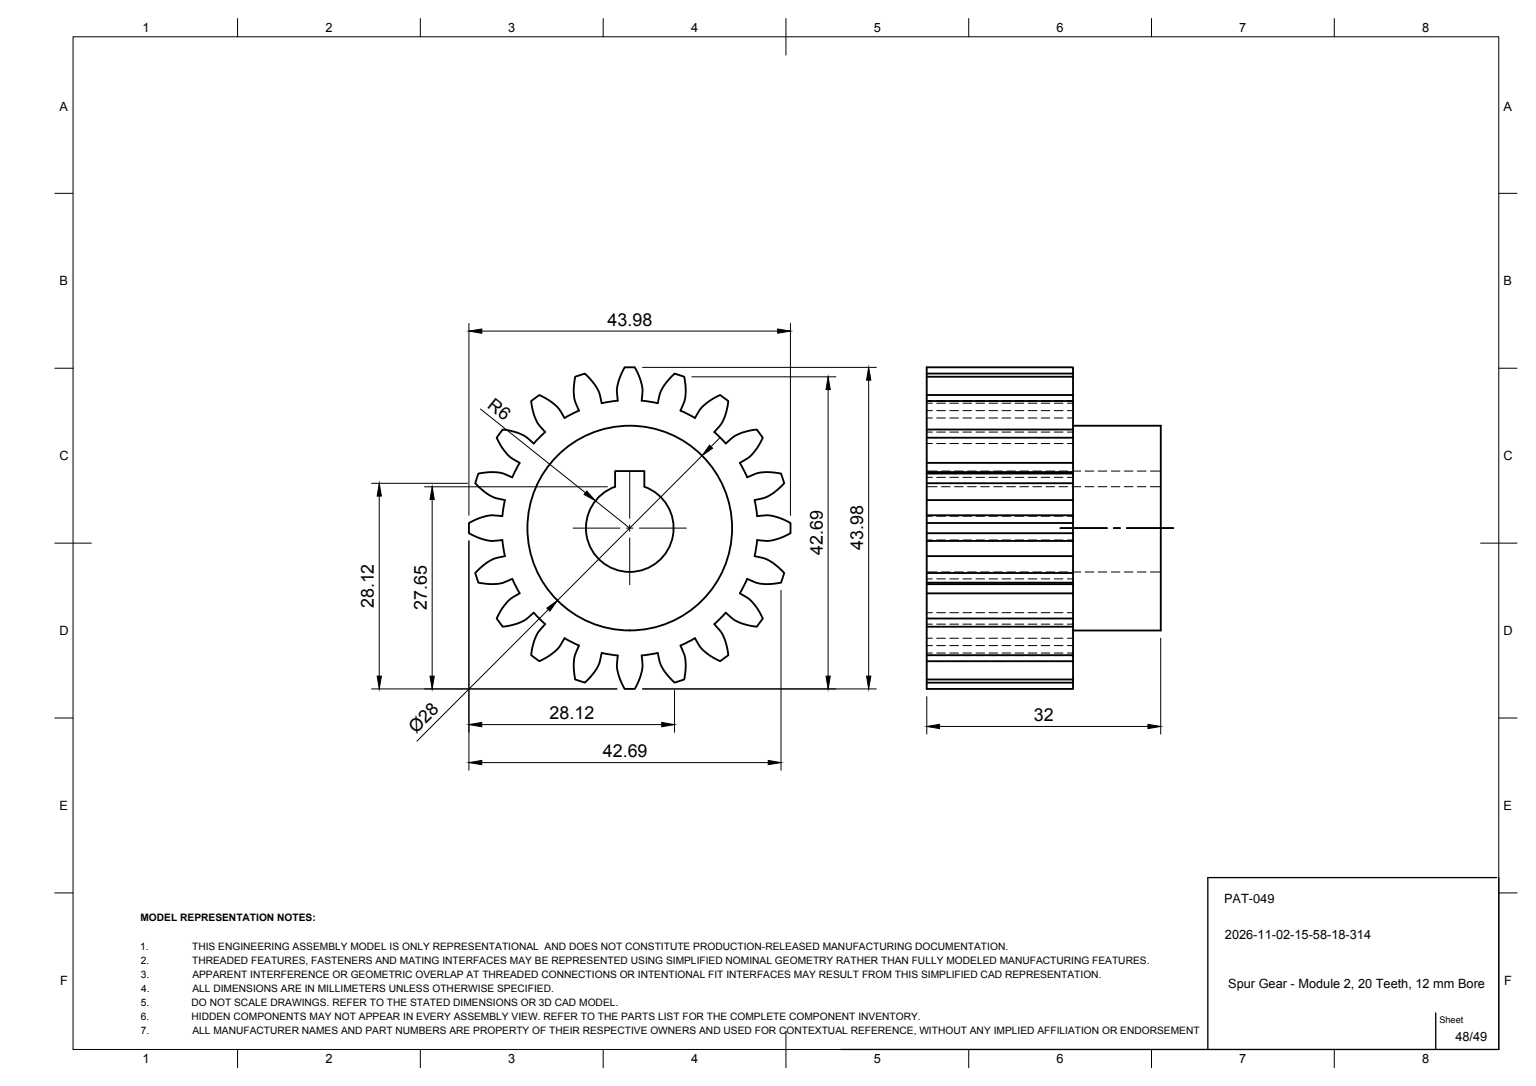
ISO-10303-21;
HEADER;
/* Generated by software containing ST-Developer
 * from STEP Tools, Inc. (www.steptools.com) 
 */

FILE_DESCRIPTION(
/* description */ ('Hand drill press frame (manual)'),
/* implementation_level */ '2;1');

FILE_NAME(
/* name */ 'Spur Gear - Module 2, 20 Teeth, 12 mm Bore.step',
/* time_stamp */ '2026-10-28T03:25:28-07:00',
/* author */ (''),
/* organization */ (''),
/* preprocessor_version */ 'ST-DEVELOPER v20.2',
/* originating_system */ 'Autodesk Translation Framework v15.17.0.0',
/* authorisation */ '');

FILE_SCHEMA (('AUTOMOTIVE_DESIGN { 1 0 10303 214 3 1 1 }'));
ENDSEC;

DATA;
#10=MECHANICAL_DESIGN_GEOMETRIC_PRESENTATION_REPRESENTATION('',(#666),#33299);
#11=(
BOUNDED_SURFACE()
B_SPLINE_SURFACE(5,1,((#24315,#24316),(#24317,#24318),(#24319,#24320),(#24321,
#24322),(#24323,#24324),(#24325,#24326),(#24327,#24328),(#24329,#24330),
(#24331,#24332),(#24333,#24334),(#24335,#24336),(#24337,#24338),(#24339,
#24340),(#24341,#24342),(#24343,#24344),(#24345,#24346),(#24347,#24348),
(#24349,#24350),(#24351,#24352),(#24353,#24354),(#24355,#24356),(#24357,
#24358),(#24359,#24360),(#24361,#24362),(#24363,#24364),(#24365,#24366),
(#24367,#24368),(#24369,#24370),(#24371,#24372),(#24373,#24374),(#24375,
#24376),(#24377,#24378),(#24379,#24380),(#24381,#24382),(#24383,#24384),
(#24385,#24386),(#24387,#24388),(#24389,#24390),(#24391,#24392),(#24393,
#24394),(#24395,#24396),(#24397,#24398),(#24399,#24400),(#24401,#24402),
(#24403,#24404),(#24405,#24406),(#24407,#24408),(#24409,#24410),(#24411,
#24412),(#24413,#24414),(#24415,#24416),(#24417,#24418),(#24419,#24420),
(#24421,#24422),(#24423,#24424),(#24425,#24426),(#24427,#24428),(#24429,
#24430),(#24431,#24432),(#24433,#24434),(#24435,#24436),(#24437,#24438),
(#24439,#24440),(#24441,#24442),(#24443,#24444),(#24445,#24446),(#24447,
#24448),(#24449,#24450),(#24451,#24452),(#24453,#24454)),.UNSPECIFIED.,
 .F.,.F.,.F.)
B_SPLINE_SURFACE_WITH_KNOTS((6,1,1,1,1,1,1,1,1,1,1,1,1,1,1,1,1,1,1,1,1,
1,1,1,1,1,1,1,1,1,1,1,1,1,1,1,1,1,1,1,1,1,1,1,1,1,1,1,1,1,1,1,1,1,1,1,1,
1,1,1,1,1,1,1,1,6),(2,2),(-1.,-0.984615384615383,-0.969230769230768,-0.953846153846152,
-0.938461538461537,-0.923076923076922,-0.907692307692306,-0.892307692307691,
-0.876923076923076,-0.86153846153846,-0.846153846153845,-0.83076923076923,
-0.815384615384614,-0.799999999999999,-0.784615384615384,-0.769230769230768,
-0.753846153846153,-0.738461538461538,-0.723076923076922,-0.707692307692307,
-0.692307692307692,-0.676923076923076,-0.661538461538461,-0.646153846153846,
-0.63076923076923,-0.615384615384615,-0.6,-0.584615384615384,-0.569230769230769,
-0.553846153846154,-0.538461538461538,-0.523076923076923,-0.507692307692308,
-0.492307692307692,-0.476923076923077,-0.461538461538462,-0.446153846153846,
-0.430769230769231,-0.415384615384615,-0.4,-0.384615384615385,-0.369230769230769,
-0.353846153846154,-0.338461538461538,-0.323076923076923,-0.307692307692308,
-0.292307692307692,-0.276923076923077,-0.261538461538462,-0.246153846153846,
-0.230769230769231,-0.215384615384615,-0.2,-0.184615384615385,-0.169230769230769,
-0.153846153846154,-0.138461538461538,-0.123076923076923,-0.107692307692308,
-0.0923076923076923,-0.0769230769230769,-0.0615384615384615,-0.0461538461538462,
-0.0307692307692308,-0.0153846153846154,0.),(-1.,1.),.UNSPECIFIED.)
GEOMETRIC_REPRESENTATION_ITEM()
RATIONAL_B_SPLINE_SURFACE(((1.,1.),(1.,1.),(1.,1.),(1.,1.),(1.,1.),(1.,
1.),(1.,1.),(1.,1.),(1.,1.),(1.,1.),(1.,1.),(1.,1.),(1.,1.),(1.,1.),(1.,
1.),(1.,1.),(1.,1.),(1.,1.),(1.,1.),(1.,1.),(1.,1.),(1.,1.),(1.,1.),(1.,
1.),(1.,1.),(1.,1.),(1.,1.),(1.,1.),(1.,1.),(1.,1.),(1.,1.),(1.,1.),(1.,
1.),(1.,1.),(1.,1.),(1.,1.),(1.,1.),(1.,1.),(1.,1.),(1.,1.),(1.,1.),(1.,
1.),(1.,1.),(1.,1.),(1.,1.),(1.,1.),(1.,1.),(1.,1.),(1.,1.),(1.,1.),(1.,
1.),(1.,1.),(1.,1.),(1.,1.),(1.,1.),(1.,1.),(1.,1.),(1.,1.),(1.,1.),(1.,
1.),(1.,1.),(1.,1.),(1.,1.),(1.,1.),(1.,1.),(1.,1.),(1.,1.),(1.,1.),(1.,
1.),(1.,1.)))
REPRESENTATION_ITEM('')
SURFACE()
);
#12=(
BOUNDED_SURFACE()
B_SPLINE_SURFACE(5,1,((#24533,#24534),(#24535,#24536),(#24537,#24538),(#24539,
#24540),(#24541,#24542),(#24543,#24544),(#24545,#24546),(#24547,#24548),
(#24549,#24550),(#24551,#24552),(#24553,#24554),(#24555,#24556),(#24557,
#24558),(#24559,#24560),(#24561,#24562),(#24563,#24564),(#24565,#24566),
(#24567,#24568),(#24569,#24570),(#24571,#24572),(#24573,#24574),(#24575,
#24576),(#24577,#24578),(#24579,#24580),(#24581,#24582),(#24583,#24584),
(#24585,#24586),(#24587,#24588),(#24589,#24590),(#24591,#24592),(#24593,
#24594),(#24595,#24596),(#24597,#24598),(#24599,#24600),(#24601,#24602),
(#24603,#24604),(#24605,#24606),(#24607,#24608),(#24609,#24610),(#24611,
#24612),(#24613,#24614),(#24615,#24616),(#24617,#24618),(#24619,#24620),
(#24621,#24622),(#24623,#24624),(#24625,#24626),(#24627,#24628),(#24629,
#24630),(#24631,#24632),(#24633,#24634),(#24635,#24636),(#24637,#24638),
(#24639,#24640),(#24641,#24642),(#24643,#24644),(#24645,#24646),(#24647,
#24648),(#24649,#24650),(#24651,#24652),(#24653,#24654),(#24655,#24656),
(#24657,#24658),(#24659,#24660),(#24661,#24662),(#24663,#24664),(#24665,
#24666),(#24667,#24668),(#24669,#24670),(#24671,#24672)),.UNSPECIFIED.,
 .F.,.F.,.F.)
B_SPLINE_SURFACE_WITH_KNOTS((6,1,1,1,1,1,1,1,1,1,1,1,1,1,1,1,1,1,1,1,1,
1,1,1,1,1,1,1,1,1,1,1,1,1,1,1,1,1,1,1,1,1,1,1,1,1,1,1,1,1,1,1,1,1,1,1,1,
1,1,1,1,1,1,1,1,6),(2,2),(-1.,-0.984615384615383,-0.969230769230768,-0.953846153846152,
-0.938461538461537,-0.923076923076922,-0.907692307692306,-0.892307692307691,
-0.876923076923076,-0.86153846153846,-0.846153846153845,-0.83076923076923,
-0.815384615384614,-0.799999999999999,-0.784615384615384,-0.769230769230768,
-0.753846153846153,-0.738461538461538,-0.723076923076922,-0.707692307692307,
-0.692307692307692,-0.676923076923076,-0.661538461538461,-0.646153846153846,
-0.63076923076923,-0.615384615384615,-0.6,-0.584615384615384,-0.569230769230769,
-0.553846153846154,-0.538461538461538,-0.523076923076923,-0.507692307692308,
-0.492307692307692,-0.476923076923077,-0.461538461538462,-0.446153846153846,
-0.430769230769231,-0.415384615384615,-0.4,-0.384615384615385,-0.369230769230769,
-0.353846153846154,-0.338461538461538,-0.323076923076923,-0.307692307692308,
-0.292307692307692,-0.276923076923077,-0.261538461538462,-0.246153846153846,
-0.230769230769231,-0.215384615384615,-0.2,-0.184615384615385,-0.169230769230769,
-0.153846153846154,-0.138461538461538,-0.123076923076923,-0.107692307692308,
-0.0923076923076923,-0.0769230769230769,-0.0615384615384615,-0.0461538461538462,
-0.0307692307692308,-0.0153846153846154,0.),(-1.,1.),.UNSPECIFIED.)
GEOMETRIC_REPRESENTATION_ITEM()
RATIONAL_B_SPLINE_SURFACE(((1.,1.),(1.,1.),(1.,1.),(1.,1.),(1.,1.),(1.,
1.),(1.,1.),(1.,1.),(1.,1.),(1.,1.),(1.,1.),(1.,1.),(1.,1.),(1.,1.),(1.,
1.),(1.,1.),(1.,1.),(1.,1.),(1.,1.),(1.,1.),(1.,1.),(1.,1.),(1.,1.),(1.,
1.),(1.,1.),(1.,1.),(1.,1.),(1.,1.),(1.,1.),(1.,1.),(1.,1.),(1.,1.),(1.,
1.),(1.,1.),(1.,1.),(1.,1.),(1.,1.),(1.,1.),(1.,1.),(1.,1.),(1.,1.),(1.,
1.),(1.,1.),(1.,1.),(1.,1.),(1.,1.),(1.,1.),(1.,1.),(1.,1.),(1.,1.),(1.,
1.),(1.,1.),(1.,1.),(1.,1.),(1.,1.),(1.,1.),(1.,1.),(1.,1.),(1.,1.),(1.,
1.),(1.,1.),(1.,1.),(1.,1.),(1.,1.),(1.,1.),(1.,1.),(1.,1.),(1.,1.),(1.,
1.),(1.,1.)))
REPRESENTATION_ITEM('')
SURFACE()
);
#13=(
BOUNDED_SURFACE()
B_SPLINE_SURFACE(5,1,((#24749,#24750),(#24751,#24752),(#24753,#24754),(#24755,
#24756),(#24757,#24758),(#24759,#24760),(#24761,#24762),(#24763,#24764),
(#24765,#24766),(#24767,#24768),(#24769,#24770),(#24771,#24772),(#24773,
#24774),(#24775,#24776),(#24777,#24778),(#24779,#24780),(#24781,#24782),
(#24783,#24784),(#24785,#24786),(#24787,#24788),(#24789,#24790),(#24791,
#24792),(#24793,#24794),(#24795,#24796),(#24797,#24798),(#24799,#24800),
(#24801,#24802),(#24803,#24804),(#24805,#24806),(#24807,#24808),(#24809,
#24810),(#24811,#24812),(#24813,#24814),(#24815,#24816),(#24817,#24818),
(#24819,#24820),(#24821,#24822),(#24823,#24824),(#24825,#24826),(#24827,
#24828),(#24829,#24830),(#24831,#24832),(#24833,#24834),(#24835,#24836),
(#24837,#24838),(#24839,#24840),(#24841,#24842),(#24843,#24844),(#24845,
#24846),(#24847,#24848),(#24849,#24850),(#24851,#24852),(#24853,#24854),
(#24855,#24856),(#24857,#24858),(#24859,#24860),(#24861,#24862),(#24863,
#24864),(#24865,#24866),(#24867,#24868),(#24869,#24870),(#24871,#24872),
(#24873,#24874),(#24875,#24876),(#24877,#24878),(#24879,#24880),(#24881,
#24882),(#24883,#24884),(#24885,#24886),(#24887,#24888)),.UNSPECIFIED.,
 .F.,.F.,.F.)
B_SPLINE_SURFACE_WITH_KNOTS((6,1,1,1,1,1,1,1,1,1,1,1,1,1,1,1,1,1,1,1,1,
1,1,1,1,1,1,1,1,1,1,1,1,1,1,1,1,1,1,1,1,1,1,1,1,1,1,1,1,1,1,1,1,1,1,1,1,
1,1,1,1,1,1,1,1,6),(2,2),(-1.,-0.984615384615383,-0.969230769230768,-0.953846153846152,
-0.938461538461537,-0.923076923076922,-0.907692307692306,-0.892307692307691,
-0.876923076923076,-0.86153846153846,-0.846153846153845,-0.83076923076923,
-0.815384615384614,-0.799999999999999,-0.784615384615384,-0.769230769230768,
-0.753846153846153,-0.738461538461538,-0.723076923076922,-0.707692307692307,
-0.692307692307692,-0.676923076923076,-0.661538461538461,-0.646153846153846,
-0.63076923076923,-0.615384615384615,-0.6,-0.584615384615384,-0.569230769230769,
-0.553846153846154,-0.538461538461538,-0.523076923076923,-0.507692307692308,
-0.492307692307692,-0.476923076923077,-0.461538461538462,-0.446153846153846,
-0.430769230769231,-0.415384615384615,-0.4,-0.384615384615385,-0.369230769230769,
-0.353846153846154,-0.338461538461538,-0.323076923076923,-0.307692307692308,
-0.292307692307692,-0.276923076923077,-0.261538461538462,-0.246153846153846,
-0.230769230769231,-0.215384615384615,-0.2,-0.184615384615385,-0.169230769230769,
-0.153846153846154,-0.138461538461538,-0.123076923076923,-0.107692307692308,
-0.0923076923076923,-0.0769230769230769,-0.0615384615384615,-0.0461538461538462,
-0.0307692307692308,-0.0153846153846154,0.),(-1.,1.),.UNSPECIFIED.)
GEOMETRIC_REPRESENTATION_ITEM()
RATIONAL_B_SPLINE_SURFACE(((1.,1.),(1.,1.),(1.,1.),(1.,1.),(1.,1.),(1.,
1.),(1.,1.),(1.,1.),(1.,1.),(1.,1.),(1.,1.),(1.,1.),(1.,1.),(1.,1.),(1.,
1.),(1.,1.),(1.,1.),(1.,1.),(1.,1.),(1.,1.),(1.,1.),(1.,1.),(1.,1.),(1.,
1.),(1.,1.),(1.,1.),(1.,1.),(1.,1.),(1.,1.),(1.,1.),(1.,1.),(1.,1.),(1.,
1.),(1.,1.),(1.,1.),(1.,1.),(1.,1.),(1.,1.),(1.,1.),(1.,1.),(1.,1.),(1.,
1.),(1.,1.),(1.,1.),(1.,1.),(1.,1.),(1.,1.),(1.,1.),(1.,1.),(1.,1.),(1.,
1.),(1.,1.),(1.,1.),(1.,1.),(1.,1.),(1.,1.),(1.,1.),(1.,1.),(1.,1.),(1.,
1.),(1.,1.),(1.,1.),(1.,1.),(1.,1.),(1.,1.),(1.,1.),(1.,1.),(1.,1.),(1.,
1.),(1.,1.)))
REPRESENTATION_ITEM('')
SURFACE()
);
#14=(
BOUNDED_SURFACE()
B_SPLINE_SURFACE(5,1,((#24965,#24966),(#24967,#24968),(#24969,#24970),(#24971,
#24972),(#24973,#24974),(#24975,#24976),(#24977,#24978),(#24979,#24980),
(#24981,#24982),(#24983,#24984),(#24985,#24986),(#24987,#24988),(#24989,
#24990),(#24991,#24992),(#24993,#24994),(#24995,#24996),(#24997,#24998),
(#24999,#25000),(#25001,#25002),(#25003,#25004),(#25005,#25006),(#25007,
#25008),(#25009,#25010),(#25011,#25012),(#25013,#25014),(#25015,#25016),
(#25017,#25018),(#25019,#25020),(#25021,#25022),(#25023,#25024),(#25025,
#25026),(#25027,#25028),(#25029,#25030),(#25031,#25032),(#25033,#25034),
(#25035,#25036),(#25037,#25038),(#25039,#25040),(#25041,#25042),(#25043,
#25044),(#25045,#25046),(#25047,#25048),(#25049,#25050),(#25051,#25052),
(#25053,#25054),(#25055,#25056),(#25057,#25058),(#25059,#25060),(#25061,
#25062),(#25063,#25064),(#25065,#25066),(#25067,#25068),(#25069,#25070),
(#25071,#25072),(#25073,#25074),(#25075,#25076),(#25077,#25078),(#25079,
#25080),(#25081,#25082),(#25083,#25084),(#25085,#25086),(#25087,#25088),
(#25089,#25090),(#25091,#25092),(#25093,#25094),(#25095,#25096),(#25097,
#25098),(#25099,#25100),(#25101,#25102),(#25103,#25104)),.UNSPECIFIED.,
 .F.,.F.,.F.)
B_SPLINE_SURFACE_WITH_KNOTS((6,1,1,1,1,1,1,1,1,1,1,1,1,1,1,1,1,1,1,1,1,
1,1,1,1,1,1,1,1,1,1,1,1,1,1,1,1,1,1,1,1,1,1,1,1,1,1,1,1,1,1,1,1,1,1,1,1,
1,1,1,1,1,1,1,1,6),(2,2),(-1.,-0.984615384615383,-0.969230769230768,-0.953846153846152,
-0.938461538461537,-0.923076923076922,-0.907692307692306,-0.892307692307691,
-0.876923076923076,-0.86153846153846,-0.846153846153845,-0.83076923076923,
-0.815384615384614,-0.799999999999999,-0.784615384615384,-0.769230769230768,
-0.753846153846153,-0.738461538461538,-0.723076923076922,-0.707692307692307,
-0.692307692307692,-0.676923076923076,-0.661538461538461,-0.646153846153846,
-0.63076923076923,-0.615384615384615,-0.6,-0.584615384615384,-0.569230769230769,
-0.553846153846154,-0.538461538461538,-0.523076923076923,-0.507692307692308,
-0.492307692307692,-0.476923076923077,-0.461538461538462,-0.446153846153846,
-0.430769230769231,-0.415384615384615,-0.4,-0.384615384615385,-0.369230769230769,
-0.353846153846154,-0.338461538461538,-0.323076923076923,-0.307692307692308,
-0.292307692307692,-0.276923076923077,-0.261538461538462,-0.246153846153846,
-0.230769230769231,-0.215384615384615,-0.2,-0.184615384615385,-0.169230769230769,
-0.153846153846154,-0.138461538461538,-0.123076923076923,-0.107692307692308,
-0.0923076923076923,-0.0769230769230769,-0.0615384615384615,-0.0461538461538462,
-0.0307692307692308,-0.0153846153846154,0.),(-1.,1.),.UNSPECIFIED.)
GEOMETRIC_REPRESENTATION_ITEM()
RATIONAL_B_SPLINE_SURFACE(((1.,1.),(1.,1.),(1.,1.),(1.,1.),(1.,1.),(1.,
1.),(1.,1.),(1.,1.),(1.,1.),(1.,1.),(1.,1.),(1.,1.),(1.,1.),(1.,1.),(1.,
1.),(1.,1.),(1.,1.),(1.,1.),(1.,1.),(1.,1.),(1.,1.),(1.,1.),(1.,1.),(1.,
1.),(1.,1.),(1.,1.),(1.,1.),(1.,1.),(1.,1.),(1.,1.),(1.,1.),(1.,1.),(1.,
1.),(1.,1.),(1.,1.),(1.,1.),(1.,1.),(1.,1.),(1.,1.),(1.,1.),(1.,1.),(1.,
1.),(1.,1.),(1.,1.),(1.,1.),(1.,1.),(1.,1.),(1.,1.),(1.,1.),(1.,1.),(1.,
1.),(1.,1.),(1.,1.),(1.,1.),(1.,1.),(1.,1.),(1.,1.),(1.,1.),(1.,1.),(1.,
1.),(1.,1.),(1.,1.),(1.,1.),(1.,1.),(1.,1.),(1.,1.),(1.,1.),(1.,1.),(1.,
1.),(1.,1.)))
REPRESENTATION_ITEM('')
SURFACE()
);
#15=(
BOUNDED_SURFACE()
B_SPLINE_SURFACE(5,1,((#25181,#25182),(#25183,#25184),(#25185,#25186),(#25187,
#25188),(#25189,#25190),(#25191,#25192),(#25193,#25194),(#25195,#25196),
(#25197,#25198),(#25199,#25200),(#25201,#25202),(#25203,#25204),(#25205,
#25206),(#25207,#25208),(#25209,#25210),(#25211,#25212),(#25213,#25214),
(#25215,#25216),(#25217,#25218),(#25219,#25220),(#25221,#25222),(#25223,
#25224),(#25225,#25226),(#25227,#25228),(#25229,#25230),(#25231,#25232),
(#25233,#25234),(#25235,#25236),(#25237,#25238),(#25239,#25240),(#25241,
#25242),(#25243,#25244),(#25245,#25246),(#25247,#25248),(#25249,#25250),
(#25251,#25252),(#25253,#25254),(#25255,#25256),(#25257,#25258),(#25259,
#25260),(#25261,#25262),(#25263,#25264),(#25265,#25266),(#25267,#25268),
(#25269,#25270),(#25271,#25272),(#25273,#25274),(#25275,#25276),(#25277,
#25278),(#25279,#25280),(#25281,#25282),(#25283,#25284),(#25285,#25286),
(#25287,#25288),(#25289,#25290),(#25291,#25292),(#25293,#25294),(#25295,
#25296),(#25297,#25298),(#25299,#25300),(#25301,#25302),(#25303,#25304),
(#25305,#25306),(#25307,#25308),(#25309,#25310),(#25311,#25312),(#25313,
#25314),(#25315,#25316),(#25317,#25318),(#25319,#25320)),.UNSPECIFIED.,
 .F.,.F.,.F.)
B_SPLINE_SURFACE_WITH_KNOTS((6,1,1,1,1,1,1,1,1,1,1,1,1,1,1,1,1,1,1,1,1,
1,1,1,1,1,1,1,1,1,1,1,1,1,1,1,1,1,1,1,1,1,1,1,1,1,1,1,1,1,1,1,1,1,1,1,1,
1,1,1,1,1,1,1,1,6),(2,2),(-1.,-0.984615384615383,-0.969230769230768,-0.953846153846152,
-0.938461538461537,-0.923076923076922,-0.907692307692306,-0.892307692307691,
-0.876923076923076,-0.86153846153846,-0.846153846153845,-0.83076923076923,
-0.815384615384614,-0.799999999999999,-0.784615384615384,-0.769230769230768,
-0.753846153846153,-0.738461538461538,-0.723076923076922,-0.707692307692307,
-0.692307692307692,-0.676923076923076,-0.661538461538461,-0.646153846153846,
-0.63076923076923,-0.615384615384615,-0.6,-0.584615384615384,-0.569230769230769,
-0.553846153846154,-0.538461538461538,-0.523076923076923,-0.507692307692308,
-0.492307692307692,-0.476923076923077,-0.461538461538462,-0.446153846153846,
-0.430769230769231,-0.415384615384615,-0.4,-0.384615384615385,-0.369230769230769,
-0.353846153846154,-0.338461538461538,-0.323076923076923,-0.307692307692308,
-0.292307692307692,-0.276923076923077,-0.261538461538462,-0.246153846153846,
-0.230769230769231,-0.215384615384615,-0.2,-0.184615384615385,-0.169230769230769,
-0.153846153846154,-0.138461538461538,-0.123076923076923,-0.107692307692308,
-0.0923076923076923,-0.0769230769230769,-0.0615384615384615,-0.0461538461538462,
-0.0307692307692308,-0.0153846153846154,0.),(-1.,1.),.UNSPECIFIED.)
GEOMETRIC_REPRESENTATION_ITEM()
RATIONAL_B_SPLINE_SURFACE(((1.,1.),(1.,1.),(1.,1.),(1.,1.),(1.,1.),(1.,
1.),(1.,1.),(1.,1.),(1.,1.),(1.,1.),(1.,1.),(1.,1.),(1.,1.),(1.,1.),(1.,
1.),(1.,1.),(1.,1.),(1.,1.),(1.,1.),(1.,1.),(1.,1.),(1.,1.),(1.,1.),(1.,
1.),(1.,1.),(1.,1.),(1.,1.),(1.,1.),(1.,1.),(1.,1.),(1.,1.),(1.,1.),(1.,
1.),(1.,1.),(1.,1.),(1.,1.),(1.,1.),(1.,1.),(1.,1.),(1.,1.),(1.,1.),(1.,
1.),(1.,1.),(1.,1.),(1.,1.),(1.,1.),(1.,1.),(1.,1.),(1.,1.),(1.,1.),(1.,
1.),(1.,1.),(1.,1.),(1.,1.),(1.,1.),(1.,1.),(1.,1.),(1.,1.),(1.,1.),(1.,
1.),(1.,1.),(1.,1.),(1.,1.),(1.,1.),(1.,1.),(1.,1.),(1.,1.),(1.,1.),(1.,
1.),(1.,1.)))
REPRESENTATION_ITEM('')
SURFACE()
);
#16=(
BOUNDED_SURFACE()
B_SPLINE_SURFACE(5,1,((#25397,#25398),(#25399,#25400),(#25401,#25402),(#25403,
#25404),(#25405,#25406),(#25407,#25408),(#25409,#25410),(#25411,#25412),
(#25413,#25414),(#25415,#25416),(#25417,#25418),(#25419,#25420),(#25421,
#25422),(#25423,#25424),(#25425,#25426),(#25427,#25428),(#25429,#25430),
(#25431,#25432),(#25433,#25434),(#25435,#25436),(#25437,#25438),(#25439,
#25440),(#25441,#25442),(#25443,#25444),(#25445,#25446),(#25447,#25448),
(#25449,#25450),(#25451,#25452),(#25453,#25454),(#25455,#25456),(#25457,
#25458),(#25459,#25460),(#25461,#25462),(#25463,#25464),(#25465,#25466),
(#25467,#25468),(#25469,#25470),(#25471,#25472),(#25473,#25474),(#25475,
#25476),(#25477,#25478),(#25479,#25480),(#25481,#25482),(#25483,#25484),
(#25485,#25486),(#25487,#25488),(#25489,#25490),(#25491,#25492),(#25493,
#25494),(#25495,#25496),(#25497,#25498),(#25499,#25500),(#25501,#25502),
(#25503,#25504),(#25505,#25506),(#25507,#25508),(#25509,#25510),(#25511,
#25512),(#25513,#25514),(#25515,#25516),(#25517,#25518),(#25519,#25520),
(#25521,#25522),(#25523,#25524),(#25525,#25526),(#25527,#25528),(#25529,
#25530),(#25531,#25532),(#25533,#25534),(#25535,#25536)),.UNSPECIFIED.,
 .F.,.F.,.F.)
B_SPLINE_SURFACE_WITH_KNOTS((6,1,1,1,1,1,1,1,1,1,1,1,1,1,1,1,1,1,1,1,1,
1,1,1,1,1,1,1,1,1,1,1,1,1,1,1,1,1,1,1,1,1,1,1,1,1,1,1,1,1,1,1,1,1,1,1,1,
1,1,1,1,1,1,1,1,6),(2,2),(-1.,-0.984615384615383,-0.969230769230768,-0.953846153846152,
-0.938461538461537,-0.923076923076922,-0.907692307692306,-0.892307692307691,
-0.876923076923076,-0.86153846153846,-0.846153846153845,-0.83076923076923,
-0.815384615384614,-0.799999999999999,-0.784615384615384,-0.769230769230768,
-0.753846153846153,-0.738461538461538,-0.723076923076922,-0.707692307692307,
-0.692307692307692,-0.676923076923076,-0.661538461538461,-0.646153846153846,
-0.63076923076923,-0.615384615384615,-0.6,-0.584615384615384,-0.569230769230769,
-0.553846153846154,-0.538461538461538,-0.523076923076923,-0.507692307692308,
-0.492307692307692,-0.476923076923077,-0.461538461538462,-0.446153846153846,
-0.430769230769231,-0.415384615384615,-0.4,-0.384615384615385,-0.369230769230769,
-0.353846153846154,-0.338461538461538,-0.323076923076923,-0.307692307692308,
-0.292307692307692,-0.276923076923077,-0.261538461538462,-0.246153846153846,
-0.230769230769231,-0.215384615384615,-0.2,-0.184615384615385,-0.169230769230769,
-0.153846153846154,-0.138461538461538,-0.123076923076923,-0.107692307692308,
-0.0923076923076923,-0.0769230769230769,-0.0615384615384615,-0.0461538461538462,
-0.0307692307692308,-0.0153846153846154,0.),(-1.,1.),.UNSPECIFIED.)
GEOMETRIC_REPRESENTATION_ITEM()
RATIONAL_B_SPLINE_SURFACE(((1.,1.),(1.,1.),(1.,1.),(1.,1.),(1.,1.),(1.,
1.),(1.,1.),(1.,1.),(1.,1.),(1.,1.),(1.,1.),(1.,1.),(1.,1.),(1.,1.),(1.,
1.),(1.,1.),(1.,1.),(1.,1.),(1.,1.),(1.,1.),(1.,1.),(1.,1.),(1.,1.),(1.,
1.),(1.,1.),(1.,1.),(1.,1.),(1.,1.),(1.,1.),(1.,1.),(1.,1.),(1.,1.),(1.,
1.),(1.,1.),(1.,1.),(1.,1.),(1.,1.),(1.,1.),(1.,1.),(1.,1.),(1.,1.),(1.,
1.),(1.,1.),(1.,1.),(1.,1.),(1.,1.),(1.,1.),(1.,1.),(1.,1.),(1.,1.),(1.,
1.),(1.,1.),(1.,1.),(1.,1.),(1.,1.),(1.,1.),(1.,1.),(1.,1.),(1.,1.),(1.,
1.),(1.,1.),(1.,1.),(1.,1.),(1.,1.),(1.,1.),(1.,1.),(1.,1.),(1.,1.),(1.,
1.),(1.,1.)))
REPRESENTATION_ITEM('')
SURFACE()
);
#17=(
BOUNDED_SURFACE()
B_SPLINE_SURFACE(5,1,((#25613,#25614),(#25615,#25616),(#25617,#25618),(#25619,
#25620),(#25621,#25622),(#25623,#25624),(#25625,#25626),(#25627,#25628),
(#25629,#25630),(#25631,#25632),(#25633,#25634),(#25635,#25636),(#25637,
#25638),(#25639,#25640),(#25641,#25642),(#25643,#25644),(#25645,#25646),
(#25647,#25648),(#25649,#25650),(#25651,#25652),(#25653,#25654),(#25655,
#25656),(#25657,#25658),(#25659,#25660),(#25661,#25662),(#25663,#25664),
(#25665,#25666),(#25667,#25668),(#25669,#25670),(#25671,#25672),(#25673,
#25674),(#25675,#25676),(#25677,#25678),(#25679,#25680),(#25681,#25682),
(#25683,#25684),(#25685,#25686),(#25687,#25688),(#25689,#25690),(#25691,
#25692),(#25693,#25694),(#25695,#25696),(#25697,#25698),(#25699,#25700),
(#25701,#25702),(#25703,#25704),(#25705,#25706),(#25707,#25708),(#25709,
#25710),(#25711,#25712),(#25713,#25714),(#25715,#25716),(#25717,#25718),
(#25719,#25720),(#25721,#25722),(#25723,#25724),(#25725,#25726),(#25727,
#25728),(#25729,#25730),(#25731,#25732),(#25733,#25734),(#25735,#25736),
(#25737,#25738),(#25739,#25740),(#25741,#25742),(#25743,#25744),(#25745,
#25746),(#25747,#25748),(#25749,#25750),(#25751,#25752)),.UNSPECIFIED.,
 .F.,.F.,.F.)
B_SPLINE_SURFACE_WITH_KNOTS((6,1,1,1,1,1,1,1,1,1,1,1,1,1,1,1,1,1,1,1,1,
1,1,1,1,1,1,1,1,1,1,1,1,1,1,1,1,1,1,1,1,1,1,1,1,1,1,1,1,1,1,1,1,1,1,1,1,
1,1,1,1,1,1,1,1,6),(2,2),(-1.,-0.984615384615383,-0.969230769230768,-0.953846153846152,
-0.938461538461537,-0.923076923076922,-0.907692307692306,-0.892307692307691,
-0.876923076923076,-0.86153846153846,-0.846153846153845,-0.83076923076923,
-0.815384615384614,-0.799999999999999,-0.784615384615384,-0.769230769230768,
-0.753846153846153,-0.738461538461538,-0.723076923076922,-0.707692307692307,
-0.692307692307692,-0.676923076923076,-0.661538461538461,-0.646153846153846,
-0.63076923076923,-0.615384615384615,-0.6,-0.584615384615384,-0.569230769230769,
-0.553846153846154,-0.538461538461538,-0.523076923076923,-0.507692307692308,
-0.492307692307692,-0.476923076923077,-0.461538461538462,-0.446153846153846,
-0.430769230769231,-0.415384615384615,-0.4,-0.384615384615385,-0.369230769230769,
-0.353846153846154,-0.338461538461538,-0.323076923076923,-0.307692307692308,
-0.292307692307692,-0.276923076923077,-0.261538461538462,-0.246153846153846,
-0.230769230769231,-0.215384615384615,-0.2,-0.184615384615385,-0.169230769230769,
-0.153846153846154,-0.138461538461538,-0.123076923076923,-0.107692307692308,
-0.0923076923076923,-0.0769230769230769,-0.0615384615384615,-0.0461538461538462,
-0.0307692307692308,-0.0153846153846154,0.),(-1.,1.),.UNSPECIFIED.)
GEOMETRIC_REPRESENTATION_ITEM()
RATIONAL_B_SPLINE_SURFACE(((1.,1.),(1.,1.),(1.,1.),(1.,1.),(1.,1.),(1.,
1.),(1.,1.),(1.,1.),(1.,1.),(1.,1.),(1.,1.),(1.,1.),(1.,1.),(1.,1.),(1.,
1.),(1.,1.),(1.,1.),(1.,1.),(1.,1.),(1.,1.),(1.,1.),(1.,1.),(1.,1.),(1.,
1.),(1.,1.),(1.,1.),(1.,1.),(1.,1.),(1.,1.),(1.,1.),(1.,1.),(1.,1.),(1.,
1.),(1.,1.),(1.,1.),(1.,1.),(1.,1.),(1.,1.),(1.,1.),(1.,1.),(1.,1.),(1.,
1.),(1.,1.),(1.,1.),(1.,1.),(1.,1.),(1.,1.),(1.,1.),(1.,1.),(1.,1.),(1.,
1.),(1.,1.),(1.,1.),(1.,1.),(1.,1.),(1.,1.),(1.,1.),(1.,1.),(1.,1.),(1.,
1.),(1.,1.),(1.,1.),(1.,1.),(1.,1.),(1.,1.),(1.,1.),(1.,1.),(1.,1.),(1.,
1.),(1.,1.)))
REPRESENTATION_ITEM('')
SURFACE()
);
#18=(
BOUNDED_SURFACE()
B_SPLINE_SURFACE(5,1,((#25829,#25830),(#25831,#25832),(#25833,#25834),(#25835,
#25836),(#25837,#25838),(#25839,#25840),(#25841,#25842),(#25843,#25844),
(#25845,#25846),(#25847,#25848),(#25849,#25850),(#25851,#25852),(#25853,
#25854),(#25855,#25856),(#25857,#25858),(#25859,#25860),(#25861,#25862),
(#25863,#25864),(#25865,#25866),(#25867,#25868),(#25869,#25870),(#25871,
#25872),(#25873,#25874),(#25875,#25876),(#25877,#25878),(#25879,#25880),
(#25881,#25882),(#25883,#25884),(#25885,#25886),(#25887,#25888),(#25889,
#25890),(#25891,#25892),(#25893,#25894),(#25895,#25896),(#25897,#25898),
(#25899,#25900),(#25901,#25902),(#25903,#25904),(#25905,#25906),(#25907,
#25908),(#25909,#25910),(#25911,#25912),(#25913,#25914),(#25915,#25916),
(#25917,#25918),(#25919,#25920),(#25921,#25922),(#25923,#25924),(#25925,
#25926),(#25927,#25928),(#25929,#25930),(#25931,#25932),(#25933,#25934),
(#25935,#25936),(#25937,#25938),(#25939,#25940),(#25941,#25942),(#25943,
#25944),(#25945,#25946),(#25947,#25948),(#25949,#25950),(#25951,#25952),
(#25953,#25954),(#25955,#25956),(#25957,#25958),(#25959,#25960),(#25961,
#25962),(#25963,#25964),(#25965,#25966),(#25967,#25968)),.UNSPECIFIED.,
 .F.,.F.,.F.)
B_SPLINE_SURFACE_WITH_KNOTS((6,1,1,1,1,1,1,1,1,1,1,1,1,1,1,1,1,1,1,1,1,
1,1,1,1,1,1,1,1,1,1,1,1,1,1,1,1,1,1,1,1,1,1,1,1,1,1,1,1,1,1,1,1,1,1,1,1,
1,1,1,1,1,1,1,1,6),(2,2),(-1.,-0.984615384615383,-0.969230769230768,-0.953846153846152,
-0.938461538461537,-0.923076923076922,-0.907692307692306,-0.892307692307691,
-0.876923076923076,-0.86153846153846,-0.846153846153845,-0.83076923076923,
-0.815384615384614,-0.799999999999999,-0.784615384615384,-0.769230769230768,
-0.753846153846153,-0.738461538461538,-0.723076923076922,-0.707692307692307,
-0.692307692307692,-0.676923076923076,-0.661538461538461,-0.646153846153846,
-0.63076923076923,-0.615384615384615,-0.6,-0.584615384615384,-0.569230769230769,
-0.553846153846154,-0.538461538461538,-0.523076923076923,-0.507692307692308,
-0.492307692307692,-0.476923076923077,-0.461538461538462,-0.446153846153846,
-0.430769230769231,-0.415384615384615,-0.4,-0.384615384615385,-0.369230769230769,
-0.353846153846154,-0.338461538461538,-0.323076923076923,-0.307692307692308,
-0.292307692307692,-0.276923076923077,-0.261538461538462,-0.246153846153846,
-0.230769230769231,-0.215384615384615,-0.2,-0.184615384615385,-0.169230769230769,
-0.153846153846154,-0.138461538461538,-0.123076923076923,-0.107692307692308,
-0.0923076923076923,-0.0769230769230769,-0.0615384615384615,-0.0461538461538462,
-0.0307692307692308,-0.0153846153846154,0.),(-1.,1.),.UNSPECIFIED.)
GEOMETRIC_REPRESENTATION_ITEM()
RATIONAL_B_SPLINE_SURFACE(((1.,1.),(1.,1.),(1.,1.),(1.,1.),(1.,1.),(1.,
1.),(1.,1.),(1.,1.),(1.,1.),(1.,1.),(1.,1.),(1.,1.),(1.,1.),(1.,1.),(1.,
1.),(1.,1.),(1.,1.),(1.,1.),(1.,1.),(1.,1.),(1.,1.),(1.,1.),(1.,1.),(1.,
1.),(1.,1.),(1.,1.),(1.,1.),(1.,1.),(1.,1.),(1.,1.),(1.,1.),(1.,1.),(1.,
1.),(1.,1.),(1.,1.),(1.,1.),(1.,1.),(1.,1.),(1.,1.),(1.,1.),(1.,1.),(1.,
1.),(1.,1.),(1.,1.),(1.,1.),(1.,1.),(1.,1.),(1.,1.),(1.,1.),(1.,1.),(1.,
1.),(1.,1.),(1.,1.),(1.,1.),(1.,1.),(1.,1.),(1.,1.),(1.,1.),(1.,1.),(1.,
1.),(1.,1.),(1.,1.),(1.,1.),(1.,1.),(1.,1.),(1.,1.),(1.,1.),(1.,1.),(1.,
1.),(1.,1.)))
REPRESENTATION_ITEM('')
SURFACE()
);
#19=(
BOUNDED_SURFACE()
B_SPLINE_SURFACE(5,1,((#26045,#26046),(#26047,#26048),(#26049,#26050),(#26051,
#26052),(#26053,#26054),(#26055,#26056),(#26057,#26058),(#26059,#26060),
(#26061,#26062),(#26063,#26064),(#26065,#26066),(#26067,#26068),(#26069,
#26070),(#26071,#26072),(#26073,#26074),(#26075,#26076),(#26077,#26078),
(#26079,#26080),(#26081,#26082),(#26083,#26084),(#26085,#26086),(#26087,
#26088),(#26089,#26090),(#26091,#26092),(#26093,#26094),(#26095,#26096),
(#26097,#26098),(#26099,#26100),(#26101,#26102),(#26103,#26104),(#26105,
#26106),(#26107,#26108),(#26109,#26110),(#26111,#26112),(#26113,#26114),
(#26115,#26116),(#26117,#26118),(#26119,#26120),(#26121,#26122),(#26123,
#26124),(#26125,#26126),(#26127,#26128),(#26129,#26130),(#26131,#26132),
(#26133,#26134),(#26135,#26136),(#26137,#26138),(#26139,#26140),(#26141,
#26142),(#26143,#26144),(#26145,#26146),(#26147,#26148),(#26149,#26150),
(#26151,#26152),(#26153,#26154),(#26155,#26156),(#26157,#26158),(#26159,
#26160),(#26161,#26162),(#26163,#26164),(#26165,#26166),(#26167,#26168),
(#26169,#26170),(#26171,#26172),(#26173,#26174),(#26175,#26176),(#26177,
#26178),(#26179,#26180),(#26181,#26182),(#26183,#26184)),.UNSPECIFIED.,
 .F.,.F.,.F.)
B_SPLINE_SURFACE_WITH_KNOTS((6,1,1,1,1,1,1,1,1,1,1,1,1,1,1,1,1,1,1,1,1,
1,1,1,1,1,1,1,1,1,1,1,1,1,1,1,1,1,1,1,1,1,1,1,1,1,1,1,1,1,1,1,1,1,1,1,1,
1,1,1,1,1,1,1,1,6),(2,2),(-1.,-0.984615384615383,-0.969230769230768,-0.953846153846152,
-0.938461538461537,-0.923076923076922,-0.907692307692306,-0.892307692307691,
-0.876923076923076,-0.86153846153846,-0.846153846153845,-0.83076923076923,
-0.815384615384614,-0.799999999999999,-0.784615384615384,-0.769230769230768,
-0.753846153846153,-0.738461538461538,-0.723076923076922,-0.707692307692307,
-0.692307692307692,-0.676923076923076,-0.661538461538461,-0.646153846153846,
-0.63076923076923,-0.615384615384615,-0.6,-0.584615384615384,-0.569230769230769,
-0.553846153846154,-0.538461538461538,-0.523076923076923,-0.507692307692308,
-0.492307692307692,-0.476923076923077,-0.461538461538462,-0.446153846153846,
-0.430769230769231,-0.415384615384615,-0.4,-0.384615384615385,-0.369230769230769,
-0.353846153846154,-0.338461538461538,-0.323076923076923,-0.307692307692308,
-0.292307692307692,-0.276923076923077,-0.261538461538462,-0.246153846153846,
-0.230769230769231,-0.215384615384615,-0.2,-0.184615384615385,-0.169230769230769,
-0.153846153846154,-0.138461538461538,-0.123076923076923,-0.107692307692308,
-0.0923076923076923,-0.0769230769230769,-0.0615384615384615,-0.0461538461538462,
-0.0307692307692308,-0.0153846153846154,0.),(-1.,1.),.UNSPECIFIED.)
GEOMETRIC_REPRESENTATION_ITEM()
RATIONAL_B_SPLINE_SURFACE(((1.,1.),(1.,1.),(1.,1.),(1.,1.),(1.,1.),(1.,
1.),(1.,1.),(1.,1.),(1.,1.),(1.,1.),(1.,1.),(1.,1.),(1.,1.),(1.,1.),(1.,
1.),(1.,1.),(1.,1.),(1.,1.),(1.,1.),(1.,1.),(1.,1.),(1.,1.),(1.,1.),(1.,
1.),(1.,1.),(1.,1.),(1.,1.),(1.,1.),(1.,1.),(1.,1.),(1.,1.),(1.,1.),(1.,
1.),(1.,1.),(1.,1.),(1.,1.),(1.,1.),(1.,1.),(1.,1.),(1.,1.),(1.,1.),(1.,
1.),(1.,1.),(1.,1.),(1.,1.),(1.,1.),(1.,1.),(1.,1.),(1.,1.),(1.,1.),(1.,
1.),(1.,1.),(1.,1.),(1.,1.),(1.,1.),(1.,1.),(1.,1.),(1.,1.),(1.,1.),(1.,
1.),(1.,1.),(1.,1.),(1.,1.),(1.,1.),(1.,1.),(1.,1.),(1.,1.),(1.,1.),(1.,
1.),(1.,1.)))
REPRESENTATION_ITEM('')
SURFACE()
);
#20=(
BOUNDED_SURFACE()
B_SPLINE_SURFACE(5,1,((#26261,#26262),(#26263,#26264),(#26265,#26266),(#26267,
#26268),(#26269,#26270),(#26271,#26272),(#26273,#26274),(#26275,#26276),
(#26277,#26278),(#26279,#26280),(#26281,#26282),(#26283,#26284),(#26285,
#26286),(#26287,#26288),(#26289,#26290),(#26291,#26292),(#26293,#26294),
(#26295,#26296),(#26297,#26298),(#26299,#26300),(#26301,#26302),(#26303,
#26304),(#26305,#26306),(#26307,#26308),(#26309,#26310),(#26311,#26312),
(#26313,#26314),(#26315,#26316),(#26317,#26318),(#26319,#26320),(#26321,
#26322),(#26323,#26324),(#26325,#26326),(#26327,#26328),(#26329,#26330),
(#26331,#26332),(#26333,#26334),(#26335,#26336),(#26337,#26338),(#26339,
#26340),(#26341,#26342),(#26343,#26344),(#26345,#26346),(#26347,#26348),
(#26349,#26350),(#26351,#26352),(#26353,#26354),(#26355,#26356),(#26357,
#26358),(#26359,#26360),(#26361,#26362),(#26363,#26364),(#26365,#26366),
(#26367,#26368),(#26369,#26370),(#26371,#26372),(#26373,#26374),(#26375,
#26376),(#26377,#26378),(#26379,#26380),(#26381,#26382),(#26383,#26384),
(#26385,#26386),(#26387,#26388),(#26389,#26390),(#26391,#26392),(#26393,
#26394),(#26395,#26396),(#26397,#26398),(#26399,#26400)),.UNSPECIFIED.,
 .F.,.F.,.F.)
B_SPLINE_SURFACE_WITH_KNOTS((6,1,1,1,1,1,1,1,1,1,1,1,1,1,1,1,1,1,1,1,1,
1,1,1,1,1,1,1,1,1,1,1,1,1,1,1,1,1,1,1,1,1,1,1,1,1,1,1,1,1,1,1,1,1,1,1,1,
1,1,1,1,1,1,1,1,6),(2,2),(-1.,-0.984615384615383,-0.969230769230768,-0.953846153846152,
-0.938461538461537,-0.923076923076922,-0.907692307692306,-0.892307692307691,
-0.876923076923076,-0.86153846153846,-0.846153846153845,-0.83076923076923,
-0.815384615384614,-0.799999999999999,-0.784615384615384,-0.769230769230768,
-0.753846153846153,-0.738461538461538,-0.723076923076922,-0.707692307692307,
-0.692307692307692,-0.676923076923076,-0.661538461538461,-0.646153846153846,
-0.63076923076923,-0.615384615384615,-0.6,-0.584615384615384,-0.569230769230769,
-0.553846153846154,-0.538461538461538,-0.523076923076923,-0.507692307692308,
-0.492307692307692,-0.476923076923077,-0.461538461538462,-0.446153846153846,
-0.430769230769231,-0.415384615384615,-0.4,-0.384615384615385,-0.369230769230769,
-0.353846153846154,-0.338461538461538,-0.323076923076923,-0.307692307692308,
-0.292307692307692,-0.276923076923077,-0.261538461538462,-0.246153846153846,
-0.230769230769231,-0.215384615384615,-0.2,-0.184615384615385,-0.169230769230769,
-0.153846153846154,-0.138461538461538,-0.123076923076923,-0.107692307692308,
-0.0923076923076923,-0.0769230769230769,-0.0615384615384615,-0.0461538461538462,
-0.0307692307692308,-0.0153846153846154,0.),(-1.,1.),.UNSPECIFIED.)
GEOMETRIC_REPRESENTATION_ITEM()
RATIONAL_B_SPLINE_SURFACE(((1.,1.),(1.,1.),(1.,1.),(1.,1.),(1.,1.),(1.,
1.),(1.,1.),(1.,1.),(1.,1.),(1.,1.),(1.,1.),(1.,1.),(1.,1.),(1.,1.),(1.,
1.),(1.,1.),(1.,1.),(1.,1.),(1.,1.),(1.,1.),(1.,1.),(1.,1.),(1.,1.),(1.,
1.),(1.,1.),(1.,1.),(1.,1.),(1.,1.),(1.,1.),(1.,1.),(1.,1.),(1.,1.),(1.,
1.),(1.,1.),(1.,1.),(1.,1.),(1.,1.),(1.,1.),(1.,1.),(1.,1.),(1.,1.),(1.,
1.),(1.,1.),(1.,1.),(1.,1.),(1.,1.),(1.,1.),(1.,1.),(1.,1.),(1.,1.),(1.,
1.),(1.,1.),(1.,1.),(1.,1.),(1.,1.),(1.,1.),(1.,1.),(1.,1.),(1.,1.),(1.,
1.),(1.,1.),(1.,1.),(1.,1.),(1.,1.),(1.,1.),(1.,1.),(1.,1.),(1.,1.),(1.,
1.),(1.,1.)))
REPRESENTATION_ITEM('')
SURFACE()
);
#21=(
BOUNDED_SURFACE()
B_SPLINE_SURFACE(5,1,((#26477,#26478),(#26479,#26480),(#26481,#26482),(#26483,
#26484),(#26485,#26486),(#26487,#26488),(#26489,#26490),(#26491,#26492),
(#26493,#26494),(#26495,#26496),(#26497,#26498),(#26499,#26500),(#26501,
#26502),(#26503,#26504),(#26505,#26506),(#26507,#26508),(#26509,#26510),
(#26511,#26512),(#26513,#26514),(#26515,#26516),(#26517,#26518),(#26519,
#26520),(#26521,#26522),(#26523,#26524),(#26525,#26526),(#26527,#26528),
(#26529,#26530),(#26531,#26532),(#26533,#26534),(#26535,#26536),(#26537,
#26538),(#26539,#26540),(#26541,#26542),(#26543,#26544),(#26545,#26546),
(#26547,#26548),(#26549,#26550),(#26551,#26552),(#26553,#26554),(#26555,
#26556),(#26557,#26558),(#26559,#26560),(#26561,#26562),(#26563,#26564),
(#26565,#26566),(#26567,#26568),(#26569,#26570),(#26571,#26572),(#26573,
#26574),(#26575,#26576),(#26577,#26578),(#26579,#26580),(#26581,#26582),
(#26583,#26584),(#26585,#26586),(#26587,#26588),(#26589,#26590),(#26591,
#26592),(#26593,#26594),(#26595,#26596),(#26597,#26598),(#26599,#26600),
(#26601,#26602),(#26603,#26604),(#26605,#26606),(#26607,#26608),(#26609,
#26610),(#26611,#26612),(#26613,#26614),(#26615,#26616)),.UNSPECIFIED.,
 .F.,.F.,.F.)
B_SPLINE_SURFACE_WITH_KNOTS((6,1,1,1,1,1,1,1,1,1,1,1,1,1,1,1,1,1,1,1,1,
1,1,1,1,1,1,1,1,1,1,1,1,1,1,1,1,1,1,1,1,1,1,1,1,1,1,1,1,1,1,1,1,1,1,1,1,
1,1,1,1,1,1,1,1,6),(2,2),(-1.,-0.984615384615383,-0.969230769230768,-0.953846153846152,
-0.938461538461537,-0.923076923076922,-0.907692307692306,-0.892307692307691,
-0.876923076923076,-0.86153846153846,-0.846153846153845,-0.83076923076923,
-0.815384615384614,-0.799999999999999,-0.784615384615384,-0.769230769230768,
-0.753846153846153,-0.738461538461538,-0.723076923076922,-0.707692307692307,
-0.692307692307692,-0.676923076923076,-0.661538461538461,-0.646153846153846,
-0.63076923076923,-0.615384615384615,-0.6,-0.584615384615384,-0.569230769230769,
-0.553846153846154,-0.538461538461538,-0.523076923076923,-0.507692307692308,
-0.492307692307692,-0.476923076923077,-0.461538461538462,-0.446153846153846,
-0.430769230769231,-0.415384615384615,-0.4,-0.384615384615385,-0.369230769230769,
-0.353846153846154,-0.338461538461538,-0.323076923076923,-0.307692307692308,
-0.292307692307692,-0.276923076923077,-0.261538461538462,-0.246153846153846,
-0.230769230769231,-0.215384615384615,-0.2,-0.184615384615385,-0.169230769230769,
-0.153846153846154,-0.138461538461538,-0.123076923076923,-0.107692307692308,
-0.0923076923076923,-0.0769230769230769,-0.0615384615384615,-0.0461538461538462,
-0.0307692307692308,-0.0153846153846154,0.),(-1.,1.),.UNSPECIFIED.)
GEOMETRIC_REPRESENTATION_ITEM()
RATIONAL_B_SPLINE_SURFACE(((1.,1.),(1.,1.),(1.,1.),(1.,1.),(1.,1.),(1.,
1.),(1.,1.),(1.,1.),(1.,1.),(1.,1.),(1.,1.),(1.,1.),(1.,1.),(1.,1.),(1.,
1.),(1.,1.),(1.,1.),(1.,1.),(1.,1.),(1.,1.),(1.,1.),(1.,1.),(1.,1.),(1.,
1.),(1.,1.),(1.,1.),(1.,1.),(1.,1.),(1.,1.),(1.,1.),(1.,1.),(1.,1.),(1.,
1.),(1.,1.),(1.,1.),(1.,1.),(1.,1.),(1.,1.),(1.,1.),(1.,1.),(1.,1.),(1.,
1.),(1.,1.),(1.,1.),(1.,1.),(1.,1.),(1.,1.),(1.,1.),(1.,1.),(1.,1.),(1.,
1.),(1.,1.),(1.,1.),(1.,1.),(1.,1.),(1.,1.),(1.,1.),(1.,1.),(1.,1.),(1.,
1.),(1.,1.),(1.,1.),(1.,1.),(1.,1.),(1.,1.),(1.,1.),(1.,1.),(1.,1.),(1.,
1.),(1.,1.)))
REPRESENTATION_ITEM('')
SURFACE()
);
#22=(
BOUNDED_SURFACE()
B_SPLINE_SURFACE(5,1,((#26693,#26694),(#26695,#26696),(#26697,#26698),(#26699,
#26700),(#26701,#26702),(#26703,#26704),(#26705,#26706),(#26707,#26708),
(#26709,#26710),(#26711,#26712),(#26713,#26714),(#26715,#26716),(#26717,
#26718),(#26719,#26720),(#26721,#26722),(#26723,#26724),(#26725,#26726),
(#26727,#26728),(#26729,#26730),(#26731,#26732),(#26733,#26734),(#26735,
#26736),(#26737,#26738),(#26739,#26740),(#26741,#26742),(#26743,#26744),
(#26745,#26746),(#26747,#26748),(#26749,#26750),(#26751,#26752),(#26753,
#26754),(#26755,#26756),(#26757,#26758),(#26759,#26760),(#26761,#26762),
(#26763,#26764),(#26765,#26766),(#26767,#26768),(#26769,#26770),(#26771,
#26772),(#26773,#26774),(#26775,#26776),(#26777,#26778),(#26779,#26780),
(#26781,#26782),(#26783,#26784),(#26785,#26786),(#26787,#26788),(#26789,
#26790),(#26791,#26792),(#26793,#26794),(#26795,#26796),(#26797,#26798),
(#26799,#26800),(#26801,#26802),(#26803,#26804),(#26805,#26806),(#26807,
#26808),(#26809,#26810),(#26811,#26812),(#26813,#26814),(#26815,#26816),
(#26817,#26818),(#26819,#26820),(#26821,#26822),(#26823,#26824),(#26825,
#26826),(#26827,#26828),(#26829,#26830),(#26831,#26832)),.UNSPECIFIED.,
 .F.,.F.,.F.)
B_SPLINE_SURFACE_WITH_KNOTS((6,1,1,1,1,1,1,1,1,1,1,1,1,1,1,1,1,1,1,1,1,
1,1,1,1,1,1,1,1,1,1,1,1,1,1,1,1,1,1,1,1,1,1,1,1,1,1,1,1,1,1,1,1,1,1,1,1,
1,1,1,1,1,1,1,1,6),(2,2),(-1.,-0.984615384615383,-0.969230769230768,-0.953846153846152,
-0.938461538461537,-0.923076923076922,-0.907692307692306,-0.892307692307691,
-0.876923076923076,-0.86153846153846,-0.846153846153845,-0.83076923076923,
-0.815384615384614,-0.799999999999999,-0.784615384615384,-0.769230769230768,
-0.753846153846153,-0.738461538461538,-0.723076923076922,-0.707692307692307,
-0.692307692307692,-0.676923076923076,-0.661538461538461,-0.646153846153846,
-0.63076923076923,-0.615384615384615,-0.6,-0.584615384615384,-0.569230769230769,
-0.553846153846154,-0.538461538461538,-0.523076923076923,-0.507692307692308,
-0.492307692307692,-0.476923076923077,-0.461538461538462,-0.446153846153846,
-0.430769230769231,-0.415384615384615,-0.4,-0.384615384615385,-0.369230769230769,
-0.353846153846154,-0.338461538461538,-0.323076923076923,-0.307692307692308,
-0.292307692307692,-0.276923076923077,-0.261538461538462,-0.246153846153846,
-0.230769230769231,-0.215384615384615,-0.2,-0.184615384615385,-0.169230769230769,
-0.153846153846154,-0.138461538461538,-0.123076923076923,-0.107692307692308,
-0.0923076923076923,-0.0769230769230769,-0.0615384615384615,-0.0461538461538462,
-0.0307692307692308,-0.0153846153846154,0.),(-1.,1.),.UNSPECIFIED.)
GEOMETRIC_REPRESENTATION_ITEM()
RATIONAL_B_SPLINE_SURFACE(((1.,1.),(1.,1.),(1.,1.),(1.,1.),(1.,1.),(1.,
1.),(1.,1.),(1.,1.),(1.,1.),(1.,1.),(1.,1.),(1.,1.),(1.,1.),(1.,1.),(1.,
1.),(1.,1.),(1.,1.),(1.,1.),(1.,1.),(1.,1.),(1.,1.),(1.,1.),(1.,1.),(1.,
1.),(1.,1.),(1.,1.),(1.,1.),(1.,1.),(1.,1.),(1.,1.),(1.,1.),(1.,1.),(1.,
1.),(1.,1.),(1.,1.),(1.,1.),(1.,1.),(1.,1.),(1.,1.),(1.,1.),(1.,1.),(1.,
1.),(1.,1.),(1.,1.),(1.,1.),(1.,1.),(1.,1.),(1.,1.),(1.,1.),(1.,1.),(1.,
1.),(1.,1.),(1.,1.),(1.,1.),(1.,1.),(1.,1.),(1.,1.),(1.,1.),(1.,1.),(1.,
1.),(1.,1.),(1.,1.),(1.,1.),(1.,1.),(1.,1.),(1.,1.),(1.,1.),(1.,1.),(1.,
1.),(1.,1.)))
REPRESENTATION_ITEM('')
SURFACE()
);
#23=(
BOUNDED_SURFACE()
B_SPLINE_SURFACE(5,1,((#26909,#26910),(#26911,#26912),(#26913,#26914),(#26915,
#26916),(#26917,#26918),(#26919,#26920),(#26921,#26922),(#26923,#26924),
(#26925,#26926),(#26927,#26928),(#26929,#26930),(#26931,#26932),(#26933,
#26934),(#26935,#26936),(#26937,#26938),(#26939,#26940),(#26941,#26942),
(#26943,#26944),(#26945,#26946),(#26947,#26948),(#26949,#26950),(#26951,
#26952),(#26953,#26954),(#26955,#26956),(#26957,#26958),(#26959,#26960),
(#26961,#26962),(#26963,#26964),(#26965,#26966),(#26967,#26968),(#26969,
#26970),(#26971,#26972),(#26973,#26974),(#26975,#26976),(#26977,#26978),
(#26979,#26980),(#26981,#26982),(#26983,#26984),(#26985,#26986),(#26987,
#26988),(#26989,#26990),(#26991,#26992),(#26993,#26994),(#26995,#26996),
(#26997,#26998),(#26999,#27000),(#27001,#27002),(#27003,#27004),(#27005,
#27006),(#27007,#27008),(#27009,#27010),(#27011,#27012),(#27013,#27014),
(#27015,#27016),(#27017,#27018),(#27019,#27020),(#27021,#27022),(#27023,
#27024),(#27025,#27026),(#27027,#27028),(#27029,#27030),(#27031,#27032),
(#27033,#27034),(#27035,#27036),(#27037,#27038),(#27039,#27040),(#27041,
#27042),(#27043,#27044),(#27045,#27046),(#27047,#27048)),.UNSPECIFIED.,
 .F.,.F.,.F.)
B_SPLINE_SURFACE_WITH_KNOTS((6,1,1,1,1,1,1,1,1,1,1,1,1,1,1,1,1,1,1,1,1,
1,1,1,1,1,1,1,1,1,1,1,1,1,1,1,1,1,1,1,1,1,1,1,1,1,1,1,1,1,1,1,1,1,1,1,1,
1,1,1,1,1,1,1,1,6),(2,2),(-1.,-0.984615384615383,-0.969230769230768,-0.953846153846152,
-0.938461538461537,-0.923076923076922,-0.907692307692306,-0.892307692307691,
-0.876923076923076,-0.86153846153846,-0.846153846153845,-0.83076923076923,
-0.815384615384614,-0.799999999999999,-0.784615384615384,-0.769230769230768,
-0.753846153846153,-0.738461538461538,-0.723076923076922,-0.707692307692307,
-0.692307692307692,-0.676923076923076,-0.661538461538461,-0.646153846153846,
-0.63076923076923,-0.615384615384615,-0.6,-0.584615384615384,-0.569230769230769,
-0.553846153846154,-0.538461538461538,-0.523076923076923,-0.507692307692308,
-0.492307692307692,-0.476923076923077,-0.461538461538462,-0.446153846153846,
-0.430769230769231,-0.415384615384615,-0.4,-0.384615384615385,-0.369230769230769,
-0.353846153846154,-0.338461538461538,-0.323076923076923,-0.307692307692308,
-0.292307692307692,-0.276923076923077,-0.261538461538462,-0.246153846153846,
-0.230769230769231,-0.215384615384615,-0.2,-0.184615384615385,-0.169230769230769,
-0.153846153846154,-0.138461538461538,-0.123076923076923,-0.107692307692308,
-0.0923076923076923,-0.0769230769230769,-0.0615384615384615,-0.0461538461538462,
-0.0307692307692308,-0.0153846153846154,0.),(-1.,1.),.UNSPECIFIED.)
GEOMETRIC_REPRESENTATION_ITEM()
RATIONAL_B_SPLINE_SURFACE(((1.,1.),(1.,1.),(1.,1.),(1.,1.),(1.,1.),(1.,
1.),(1.,1.),(1.,1.),(1.,1.),(1.,1.),(1.,1.),(1.,1.),(1.,1.),(1.,1.),(1.,
1.),(1.,1.),(1.,1.),(1.,1.),(1.,1.),(1.,1.),(1.,1.),(1.,1.),(1.,1.),(1.,
1.),(1.,1.),(1.,1.),(1.,1.),(1.,1.),(1.,1.),(1.,1.),(1.,1.),(1.,1.),(1.,
1.),(1.,1.),(1.,1.),(1.,1.),(1.,1.),(1.,1.),(1.,1.),(1.,1.),(1.,1.),(1.,
1.),(1.,1.),(1.,1.),(1.,1.),(1.,1.),(1.,1.),(1.,1.),(1.,1.),(1.,1.),(1.,
1.),(1.,1.),(1.,1.),(1.,1.),(1.,1.),(1.,1.),(1.,1.),(1.,1.),(1.,1.),(1.,
1.),(1.,1.),(1.,1.),(1.,1.),(1.,1.),(1.,1.),(1.,1.),(1.,1.),(1.,1.),(1.,
1.),(1.,1.)))
REPRESENTATION_ITEM('')
SURFACE()
);
#24=(
BOUNDED_SURFACE()
B_SPLINE_SURFACE(5,1,((#27125,#27126),(#27127,#27128),(#27129,#27130),(#27131,
#27132),(#27133,#27134),(#27135,#27136),(#27137,#27138),(#27139,#27140),
(#27141,#27142),(#27143,#27144),(#27145,#27146),(#27147,#27148),(#27149,
#27150),(#27151,#27152),(#27153,#27154),(#27155,#27156),(#27157,#27158),
(#27159,#27160),(#27161,#27162),(#27163,#27164),(#27165,#27166),(#27167,
#27168),(#27169,#27170),(#27171,#27172),(#27173,#27174),(#27175,#27176),
(#27177,#27178),(#27179,#27180),(#27181,#27182),(#27183,#27184),(#27185,
#27186),(#27187,#27188),(#27189,#27190),(#27191,#27192),(#27193,#27194),
(#27195,#27196),(#27197,#27198),(#27199,#27200),(#27201,#27202),(#27203,
#27204),(#27205,#27206),(#27207,#27208),(#27209,#27210),(#27211,#27212),
(#27213,#27214),(#27215,#27216),(#27217,#27218),(#27219,#27220),(#27221,
#27222),(#27223,#27224),(#27225,#27226),(#27227,#27228),(#27229,#27230),
(#27231,#27232),(#27233,#27234),(#27235,#27236),(#27237,#27238),(#27239,
#27240),(#27241,#27242),(#27243,#27244),(#27245,#27246),(#27247,#27248),
(#27249,#27250),(#27251,#27252),(#27253,#27254),(#27255,#27256),(#27257,
#27258),(#27259,#27260),(#27261,#27262),(#27263,#27264)),.UNSPECIFIED.,
 .F.,.F.,.F.)
B_SPLINE_SURFACE_WITH_KNOTS((6,1,1,1,1,1,1,1,1,1,1,1,1,1,1,1,1,1,1,1,1,
1,1,1,1,1,1,1,1,1,1,1,1,1,1,1,1,1,1,1,1,1,1,1,1,1,1,1,1,1,1,1,1,1,1,1,1,
1,1,1,1,1,1,1,1,6),(2,2),(-1.,-0.984615384615383,-0.969230769230768,-0.953846153846152,
-0.938461538461537,-0.923076923076922,-0.907692307692306,-0.892307692307691,
-0.876923076923076,-0.86153846153846,-0.846153846153845,-0.83076923076923,
-0.815384615384614,-0.799999999999999,-0.784615384615384,-0.769230769230768,
-0.753846153846153,-0.738461538461538,-0.723076923076922,-0.707692307692307,
-0.692307692307692,-0.676923076923076,-0.661538461538461,-0.646153846153846,
-0.63076923076923,-0.615384615384615,-0.6,-0.584615384615384,-0.569230769230769,
-0.553846153846154,-0.538461538461538,-0.523076923076923,-0.507692307692308,
-0.492307692307692,-0.476923076923077,-0.461538461538462,-0.446153846153846,
-0.430769230769231,-0.415384615384615,-0.4,-0.384615384615385,-0.369230769230769,
-0.353846153846154,-0.338461538461538,-0.323076923076923,-0.307692307692308,
-0.292307692307692,-0.276923076923077,-0.261538461538462,-0.246153846153846,
-0.230769230769231,-0.215384615384615,-0.2,-0.184615384615385,-0.169230769230769,
-0.153846153846154,-0.138461538461538,-0.123076923076923,-0.107692307692308,
-0.0923076923076923,-0.0769230769230769,-0.0615384615384615,-0.0461538461538462,
-0.0307692307692308,-0.0153846153846154,0.),(-1.,1.),.UNSPECIFIED.)
GEOMETRIC_REPRESENTATION_ITEM()
RATIONAL_B_SPLINE_SURFACE(((1.,1.),(1.,1.),(1.,1.),(1.,1.),(1.,1.),(1.,
1.),(1.,1.),(1.,1.),(1.,1.),(1.,1.),(1.,1.),(1.,1.),(1.,1.),(1.,1.),(1.,
1.),(1.,1.),(1.,1.),(1.,1.),(1.,1.),(1.,1.),(1.,1.),(1.,1.),(1.,1.),(1.,
1.),(1.,1.),(1.,1.),(1.,1.),(1.,1.),(1.,1.),(1.,1.),(1.,1.),(1.,1.),(1.,
1.),(1.,1.),(1.,1.),(1.,1.),(1.,1.),(1.,1.),(1.,1.),(1.,1.),(1.,1.),(1.,
1.),(1.,1.),(1.,1.),(1.,1.),(1.,1.),(1.,1.),(1.,1.),(1.,1.),(1.,1.),(1.,
1.),(1.,1.),(1.,1.),(1.,1.),(1.,1.),(1.,1.),(1.,1.),(1.,1.),(1.,1.),(1.,
1.),(1.,1.),(1.,1.),(1.,1.),(1.,1.),(1.,1.),(1.,1.),(1.,1.),(1.,1.),(1.,
1.),(1.,1.)))
REPRESENTATION_ITEM('')
SURFACE()
);
#25=(
BOUNDED_SURFACE()
B_SPLINE_SURFACE(5,1,((#27341,#27342),(#27343,#27344),(#27345,#27346),(#27347,
#27348),(#27349,#27350),(#27351,#27352),(#27353,#27354),(#27355,#27356),
(#27357,#27358),(#27359,#27360),(#27361,#27362),(#27363,#27364),(#27365,
#27366),(#27367,#27368),(#27369,#27370),(#27371,#27372),(#27373,#27374),
(#27375,#27376),(#27377,#27378),(#27379,#27380),(#27381,#27382),(#27383,
#27384),(#27385,#27386),(#27387,#27388),(#27389,#27390),(#27391,#27392),
(#27393,#27394),(#27395,#27396),(#27397,#27398),(#27399,#27400),(#27401,
#27402),(#27403,#27404),(#27405,#27406),(#27407,#27408),(#27409,#27410),
(#27411,#27412),(#27413,#27414),(#27415,#27416),(#27417,#27418),(#27419,
#27420),(#27421,#27422),(#27423,#27424),(#27425,#27426),(#27427,#27428),
(#27429,#27430),(#27431,#27432),(#27433,#27434),(#27435,#27436),(#27437,
#27438),(#27439,#27440),(#27441,#27442),(#27443,#27444),(#27445,#27446),
(#27447,#27448),(#27449,#27450),(#27451,#27452),(#27453,#27454),(#27455,
#27456),(#27457,#27458),(#27459,#27460),(#27461,#27462),(#27463,#27464),
(#27465,#27466),(#27467,#27468),(#27469,#27470),(#27471,#27472),(#27473,
#27474),(#27475,#27476),(#27477,#27478),(#27479,#27480)),.UNSPECIFIED.,
 .F.,.F.,.F.)
B_SPLINE_SURFACE_WITH_KNOTS((6,1,1,1,1,1,1,1,1,1,1,1,1,1,1,1,1,1,1,1,1,
1,1,1,1,1,1,1,1,1,1,1,1,1,1,1,1,1,1,1,1,1,1,1,1,1,1,1,1,1,1,1,1,1,1,1,1,
1,1,1,1,1,1,1,1,6),(2,2),(-1.,-0.984615384615383,-0.969230769230768,-0.953846153846152,
-0.938461538461537,-0.923076923076922,-0.907692307692306,-0.892307692307691,
-0.876923076923076,-0.86153846153846,-0.846153846153845,-0.83076923076923,
-0.815384615384614,-0.799999999999999,-0.784615384615384,-0.769230769230768,
-0.753846153846153,-0.738461538461538,-0.723076923076922,-0.707692307692307,
-0.692307692307692,-0.676923076923076,-0.661538461538461,-0.646153846153846,
-0.63076923076923,-0.615384615384615,-0.6,-0.584615384615384,-0.569230769230769,
-0.553846153846154,-0.538461538461538,-0.523076923076923,-0.507692307692308,
-0.492307692307692,-0.476923076923077,-0.461538461538462,-0.446153846153846,
-0.430769230769231,-0.415384615384615,-0.4,-0.384615384615385,-0.369230769230769,
-0.353846153846154,-0.338461538461538,-0.323076923076923,-0.307692307692308,
-0.292307692307692,-0.276923076923077,-0.261538461538462,-0.246153846153846,
-0.230769230769231,-0.215384615384615,-0.2,-0.184615384615385,-0.169230769230769,
-0.153846153846154,-0.138461538461538,-0.123076923076923,-0.107692307692308,
-0.0923076923076923,-0.0769230769230769,-0.0615384615384615,-0.0461538461538462,
-0.0307692307692308,-0.0153846153846154,0.),(-1.,1.),.UNSPECIFIED.)
GEOMETRIC_REPRESENTATION_ITEM()
RATIONAL_B_SPLINE_SURFACE(((1.,1.),(1.,1.),(1.,1.),(1.,1.),(1.,1.),(1.,
1.),(1.,1.),(1.,1.),(1.,1.),(1.,1.),(1.,1.),(1.,1.),(1.,1.),(1.,1.),(1.,
1.),(1.,1.),(1.,1.),(1.,1.),(1.,1.),(1.,1.),(1.,1.),(1.,1.),(1.,1.),(1.,
1.),(1.,1.),(1.,1.),(1.,1.),(1.,1.),(1.,1.),(1.,1.),(1.,1.),(1.,1.),(1.,
1.),(1.,1.),(1.,1.),(1.,1.),(1.,1.),(1.,1.),(1.,1.),(1.,1.),(1.,1.),(1.,
1.),(1.,1.),(1.,1.),(1.,1.),(1.,1.),(1.,1.),(1.,1.),(1.,1.),(1.,1.),(1.,
1.),(1.,1.),(1.,1.),(1.,1.),(1.,1.),(1.,1.),(1.,1.),(1.,1.),(1.,1.),(1.,
1.),(1.,1.),(1.,1.),(1.,1.),(1.,1.),(1.,1.),(1.,1.),(1.,1.),(1.,1.),(1.,
1.),(1.,1.)))
REPRESENTATION_ITEM('')
SURFACE()
);
#26=(
BOUNDED_SURFACE()
B_SPLINE_SURFACE(5,1,((#27557,#27558),(#27559,#27560),(#27561,#27562),(#27563,
#27564),(#27565,#27566),(#27567,#27568),(#27569,#27570),(#27571,#27572),
(#27573,#27574),(#27575,#27576),(#27577,#27578),(#27579,#27580),(#27581,
#27582),(#27583,#27584),(#27585,#27586),(#27587,#27588),(#27589,#27590),
(#27591,#27592),(#27593,#27594),(#27595,#27596),(#27597,#27598),(#27599,
#27600),(#27601,#27602),(#27603,#27604),(#27605,#27606),(#27607,#27608),
(#27609,#27610),(#27611,#27612),(#27613,#27614),(#27615,#27616),(#27617,
#27618),(#27619,#27620),(#27621,#27622),(#27623,#27624),(#27625,#27626),
(#27627,#27628),(#27629,#27630),(#27631,#27632),(#27633,#27634),(#27635,
#27636),(#27637,#27638),(#27639,#27640),(#27641,#27642),(#27643,#27644),
(#27645,#27646),(#27647,#27648),(#27649,#27650),(#27651,#27652),(#27653,
#27654),(#27655,#27656),(#27657,#27658),(#27659,#27660),(#27661,#27662),
(#27663,#27664),(#27665,#27666),(#27667,#27668),(#27669,#27670),(#27671,
#27672),(#27673,#27674),(#27675,#27676),(#27677,#27678),(#27679,#27680),
(#27681,#27682),(#27683,#27684),(#27685,#27686),(#27687,#27688),(#27689,
#27690),(#27691,#27692),(#27693,#27694),(#27695,#27696)),.UNSPECIFIED.,
 .F.,.F.,.F.)
B_SPLINE_SURFACE_WITH_KNOTS((6,1,1,1,1,1,1,1,1,1,1,1,1,1,1,1,1,1,1,1,1,
1,1,1,1,1,1,1,1,1,1,1,1,1,1,1,1,1,1,1,1,1,1,1,1,1,1,1,1,1,1,1,1,1,1,1,1,
1,1,1,1,1,1,1,1,6),(2,2),(-1.,-0.984615384615383,-0.969230769230768,-0.953846153846152,
-0.938461538461537,-0.923076923076922,-0.907692307692306,-0.892307692307691,
-0.876923076923076,-0.86153846153846,-0.846153846153845,-0.83076923076923,
-0.815384615384614,-0.799999999999999,-0.784615384615384,-0.769230769230768,
-0.753846153846153,-0.738461538461538,-0.723076923076922,-0.707692307692307,
-0.692307692307692,-0.676923076923076,-0.661538461538461,-0.646153846153846,
-0.63076923076923,-0.615384615384615,-0.6,-0.584615384615384,-0.569230769230769,
-0.553846153846154,-0.538461538461538,-0.523076923076923,-0.507692307692308,
-0.492307692307692,-0.476923076923077,-0.461538461538462,-0.446153846153846,
-0.430769230769231,-0.415384615384615,-0.4,-0.384615384615385,-0.369230769230769,
-0.353846153846154,-0.338461538461538,-0.323076923076923,-0.307692307692308,
-0.292307692307692,-0.276923076923077,-0.261538461538462,-0.246153846153846,
-0.230769230769231,-0.215384615384615,-0.2,-0.184615384615385,-0.169230769230769,
-0.153846153846154,-0.138461538461538,-0.123076923076923,-0.107692307692308,
-0.0923076923076923,-0.0769230769230769,-0.0615384615384615,-0.0461538461538462,
-0.0307692307692308,-0.0153846153846154,0.),(-1.,1.),.UNSPECIFIED.)
GEOMETRIC_REPRESENTATION_ITEM()
RATIONAL_B_SPLINE_SURFACE(((1.,1.),(1.,1.),(1.,1.),(1.,1.),(1.,1.),(1.,
1.),(1.,1.),(1.,1.),(1.,1.),(1.,1.),(1.,1.),(1.,1.),(1.,1.),(1.,1.),(1.,
1.),(1.,1.),(1.,1.),(1.,1.),(1.,1.),(1.,1.),(1.,1.),(1.,1.),(1.,1.),(1.,
1.),(1.,1.),(1.,1.),(1.,1.),(1.,1.),(1.,1.),(1.,1.),(1.,1.),(1.,1.),(1.,
1.),(1.,1.),(1.,1.),(1.,1.),(1.,1.),(1.,1.),(1.,1.),(1.,1.),(1.,1.),(1.,
1.),(1.,1.),(1.,1.),(1.,1.),(1.,1.),(1.,1.),(1.,1.),(1.,1.),(1.,1.),(1.,
1.),(1.,1.),(1.,1.),(1.,1.),(1.,1.),(1.,1.),(1.,1.),(1.,1.),(1.,1.),(1.,
1.),(1.,1.),(1.,1.),(1.,1.),(1.,1.),(1.,1.),(1.,1.),(1.,1.),(1.,1.),(1.,
1.),(1.,1.)))
REPRESENTATION_ITEM('')
SURFACE()
);
#27=(
BOUNDED_SURFACE()
B_SPLINE_SURFACE(5,1,((#27773,#27774),(#27775,#27776),(#27777,#27778),(#27779,
#27780),(#27781,#27782),(#27783,#27784),(#27785,#27786),(#27787,#27788),
(#27789,#27790),(#27791,#27792),(#27793,#27794),(#27795,#27796),(#27797,
#27798),(#27799,#27800),(#27801,#27802),(#27803,#27804),(#27805,#27806),
(#27807,#27808),(#27809,#27810),(#27811,#27812),(#27813,#27814),(#27815,
#27816),(#27817,#27818),(#27819,#27820),(#27821,#27822),(#27823,#27824),
(#27825,#27826),(#27827,#27828),(#27829,#27830),(#27831,#27832),(#27833,
#27834),(#27835,#27836),(#27837,#27838),(#27839,#27840),(#27841,#27842),
(#27843,#27844),(#27845,#27846),(#27847,#27848),(#27849,#27850),(#27851,
#27852),(#27853,#27854),(#27855,#27856),(#27857,#27858),(#27859,#27860),
(#27861,#27862),(#27863,#27864),(#27865,#27866),(#27867,#27868),(#27869,
#27870),(#27871,#27872),(#27873,#27874),(#27875,#27876),(#27877,#27878),
(#27879,#27880),(#27881,#27882),(#27883,#27884),(#27885,#27886),(#27887,
#27888),(#27889,#27890),(#27891,#27892),(#27893,#27894),(#27895,#27896),
(#27897,#27898),(#27899,#27900),(#27901,#27902),(#27903,#27904),(#27905,
#27906),(#27907,#27908),(#27909,#27910),(#27911,#27912)),.UNSPECIFIED.,
 .F.,.F.,.F.)
B_SPLINE_SURFACE_WITH_KNOTS((6,1,1,1,1,1,1,1,1,1,1,1,1,1,1,1,1,1,1,1,1,
1,1,1,1,1,1,1,1,1,1,1,1,1,1,1,1,1,1,1,1,1,1,1,1,1,1,1,1,1,1,1,1,1,1,1,1,
1,1,1,1,1,1,1,1,6),(2,2),(-1.,-0.984615384615383,-0.969230769230768,-0.953846153846152,
-0.938461538461537,-0.923076923076922,-0.907692307692306,-0.892307692307691,
-0.876923076923076,-0.86153846153846,-0.846153846153845,-0.83076923076923,
-0.815384615384614,-0.799999999999999,-0.784615384615384,-0.769230769230768,
-0.753846153846153,-0.738461538461538,-0.723076923076922,-0.707692307692307,
-0.692307692307692,-0.676923076923076,-0.661538461538461,-0.646153846153846,
-0.63076923076923,-0.615384615384615,-0.6,-0.584615384615384,-0.569230769230769,
-0.553846153846154,-0.538461538461538,-0.523076923076923,-0.507692307692308,
-0.492307692307692,-0.476923076923077,-0.461538461538462,-0.446153846153846,
-0.430769230769231,-0.415384615384615,-0.4,-0.384615384615385,-0.369230769230769,
-0.353846153846154,-0.338461538461538,-0.323076923076923,-0.307692307692308,
-0.292307692307692,-0.276923076923077,-0.261538461538462,-0.246153846153846,
-0.230769230769231,-0.215384615384615,-0.2,-0.184615384615385,-0.169230769230769,
-0.153846153846154,-0.138461538461538,-0.123076923076923,-0.107692307692308,
-0.0923076923076923,-0.0769230769230769,-0.0615384615384615,-0.0461538461538462,
-0.0307692307692308,-0.0153846153846154,0.),(-1.,1.),.UNSPECIFIED.)
GEOMETRIC_REPRESENTATION_ITEM()
RATIONAL_B_SPLINE_SURFACE(((1.,1.),(1.,1.),(1.,1.),(1.,1.),(1.,1.),(1.,
1.),(1.,1.),(1.,1.),(1.,1.),(1.,1.),(1.,1.),(1.,1.),(1.,1.),(1.,1.),(1.,
1.),(1.,1.),(1.,1.),(1.,1.),(1.,1.),(1.,1.),(1.,1.),(1.,1.),(1.,1.),(1.,
1.),(1.,1.),(1.,1.),(1.,1.),(1.,1.),(1.,1.),(1.,1.),(1.,1.),(1.,1.),(1.,
1.),(1.,1.),(1.,1.),(1.,1.),(1.,1.),(1.,1.),(1.,1.),(1.,1.),(1.,1.),(1.,
1.),(1.,1.),(1.,1.),(1.,1.),(1.,1.),(1.,1.),(1.,1.),(1.,1.),(1.,1.),(1.,
1.),(1.,1.),(1.,1.),(1.,1.),(1.,1.),(1.,1.),(1.,1.),(1.,1.),(1.,1.),(1.,
1.),(1.,1.),(1.,1.),(1.,1.),(1.,1.),(1.,1.),(1.,1.),(1.,1.),(1.,1.),(1.,
1.),(1.,1.)))
REPRESENTATION_ITEM('')
SURFACE()
);
#28=(
BOUNDED_SURFACE()
B_SPLINE_SURFACE(5,1,((#27989,#27990),(#27991,#27992),(#27993,#27994),(#27995,
#27996),(#27997,#27998),(#27999,#28000),(#28001,#28002),(#28003,#28004),
(#28005,#28006),(#28007,#28008),(#28009,#28010),(#28011,#28012),(#28013,
#28014),(#28015,#28016),(#28017,#28018),(#28019,#28020),(#28021,#28022),
(#28023,#28024),(#28025,#28026),(#28027,#28028),(#28029,#28030),(#28031,
#28032),(#28033,#28034),(#28035,#28036),(#28037,#28038),(#28039,#28040),
(#28041,#28042),(#28043,#28044),(#28045,#28046),(#28047,#28048),(#28049,
#28050),(#28051,#28052),(#28053,#28054),(#28055,#28056),(#28057,#28058),
(#28059,#28060),(#28061,#28062),(#28063,#28064),(#28065,#28066),(#28067,
#28068),(#28069,#28070),(#28071,#28072),(#28073,#28074),(#28075,#28076),
(#28077,#28078),(#28079,#28080),(#28081,#28082),(#28083,#28084),(#28085,
#28086),(#28087,#28088),(#28089,#28090),(#28091,#28092),(#28093,#28094),
(#28095,#28096),(#28097,#28098),(#28099,#28100),(#28101,#28102),(#28103,
#28104),(#28105,#28106),(#28107,#28108),(#28109,#28110),(#28111,#28112),
(#28113,#28114),(#28115,#28116),(#28117,#28118),(#28119,#28120),(#28121,
#28122),(#28123,#28124),(#28125,#28126),(#28127,#28128)),.UNSPECIFIED.,
 .F.,.F.,.F.)
B_SPLINE_SURFACE_WITH_KNOTS((6,1,1,1,1,1,1,1,1,1,1,1,1,1,1,1,1,1,1,1,1,
1,1,1,1,1,1,1,1,1,1,1,1,1,1,1,1,1,1,1,1,1,1,1,1,1,1,1,1,1,1,1,1,1,1,1,1,
1,1,1,1,1,1,1,1,6),(2,2),(-1.,-0.984615384615383,-0.969230769230768,-0.953846153846152,
-0.938461538461537,-0.923076923076922,-0.907692307692306,-0.892307692307691,
-0.876923076923076,-0.86153846153846,-0.846153846153845,-0.83076923076923,
-0.815384615384614,-0.799999999999999,-0.784615384615384,-0.769230769230768,
-0.753846153846153,-0.738461538461538,-0.723076923076922,-0.707692307692307,
-0.692307692307692,-0.676923076923076,-0.661538461538461,-0.646153846153846,
-0.63076923076923,-0.615384615384615,-0.6,-0.584615384615384,-0.569230769230769,
-0.553846153846154,-0.538461538461538,-0.523076923076923,-0.507692307692308,
-0.492307692307692,-0.476923076923077,-0.461538461538462,-0.446153846153846,
-0.430769230769231,-0.415384615384615,-0.4,-0.384615384615385,-0.369230769230769,
-0.353846153846154,-0.338461538461538,-0.323076923076923,-0.307692307692308,
-0.292307692307692,-0.276923076923077,-0.261538461538462,-0.246153846153846,
-0.230769230769231,-0.215384615384615,-0.2,-0.184615384615385,-0.169230769230769,
-0.153846153846154,-0.138461538461538,-0.123076923076923,-0.107692307692308,
-0.0923076923076923,-0.0769230769230769,-0.0615384615384615,-0.0461538461538462,
-0.0307692307692308,-0.0153846153846154,0.),(-1.,1.),.UNSPECIFIED.)
GEOMETRIC_REPRESENTATION_ITEM()
RATIONAL_B_SPLINE_SURFACE(((1.,1.),(1.,1.),(1.,1.),(1.,1.),(1.,1.),(1.,
1.),(1.,1.),(1.,1.),(1.,1.),(1.,1.),(1.,1.),(1.,1.),(1.,1.),(1.,1.),(1.,
1.),(1.,1.),(1.,1.),(1.,1.),(1.,1.),(1.,1.),(1.,1.),(1.,1.),(1.,1.),(1.,
1.),(1.,1.),(1.,1.),(1.,1.),(1.,1.),(1.,1.),(1.,1.),(1.,1.),(1.,1.),(1.,
1.),(1.,1.),(1.,1.),(1.,1.),(1.,1.),(1.,1.),(1.,1.),(1.,1.),(1.,1.),(1.,
1.),(1.,1.),(1.,1.),(1.,1.),(1.,1.),(1.,1.),(1.,1.),(1.,1.),(1.,1.),(1.,
1.),(1.,1.),(1.,1.),(1.,1.),(1.,1.),(1.,1.),(1.,1.),(1.,1.),(1.,1.),(1.,
1.),(1.,1.),(1.,1.),(1.,1.),(1.,1.),(1.,1.),(1.,1.),(1.,1.),(1.,1.),(1.,
1.),(1.,1.)))
REPRESENTATION_ITEM('')
SURFACE()
);
#29=(
BOUNDED_SURFACE()
B_SPLINE_SURFACE(5,1,((#28205,#28206),(#28207,#28208),(#28209,#28210),(#28211,
#28212),(#28213,#28214),(#28215,#28216),(#28217,#28218),(#28219,#28220),
(#28221,#28222),(#28223,#28224),(#28225,#28226),(#28227,#28228),(#28229,
#28230),(#28231,#28232),(#28233,#28234),(#28235,#28236),(#28237,#28238),
(#28239,#28240),(#28241,#28242),(#28243,#28244),(#28245,#28246),(#28247,
#28248),(#28249,#28250),(#28251,#28252),(#28253,#28254),(#28255,#28256),
(#28257,#28258),(#28259,#28260),(#28261,#28262),(#28263,#28264),(#28265,
#28266),(#28267,#28268),(#28269,#28270),(#28271,#28272),(#28273,#28274),
(#28275,#28276),(#28277,#28278),(#28279,#28280),(#28281,#28282),(#28283,
#28284),(#28285,#28286),(#28287,#28288),(#28289,#28290),(#28291,#28292),
(#28293,#28294),(#28295,#28296),(#28297,#28298),(#28299,#28300),(#28301,
#28302),(#28303,#28304),(#28305,#28306),(#28307,#28308),(#28309,#28310),
(#28311,#28312),(#28313,#28314),(#28315,#28316),(#28317,#28318),(#28319,
#28320),(#28321,#28322),(#28323,#28324),(#28325,#28326),(#28327,#28328),
(#28329,#28330),(#28331,#28332),(#28333,#28334),(#28335,#28336),(#28337,
#28338),(#28339,#28340),(#28341,#28342),(#28343,#28344)),.UNSPECIFIED.,
 .F.,.F.,.F.)
B_SPLINE_SURFACE_WITH_KNOTS((6,1,1,1,1,1,1,1,1,1,1,1,1,1,1,1,1,1,1,1,1,
1,1,1,1,1,1,1,1,1,1,1,1,1,1,1,1,1,1,1,1,1,1,1,1,1,1,1,1,1,1,1,1,1,1,1,1,
1,1,1,1,1,1,1,1,6),(2,2),(-1.,-0.984615384615383,-0.969230769230768,-0.953846153846152,
-0.938461538461537,-0.923076923076922,-0.907692307692306,-0.892307692307691,
-0.876923076923076,-0.86153846153846,-0.846153846153845,-0.83076923076923,
-0.815384615384614,-0.799999999999999,-0.784615384615384,-0.769230769230768,
-0.753846153846153,-0.738461538461538,-0.723076923076922,-0.707692307692307,
-0.692307692307692,-0.676923076923076,-0.661538461538461,-0.646153846153846,
-0.63076923076923,-0.615384615384615,-0.6,-0.584615384615384,-0.569230769230769,
-0.553846153846154,-0.538461538461538,-0.523076923076923,-0.507692307692308,
-0.492307692307692,-0.476923076923077,-0.461538461538462,-0.446153846153846,
-0.430769230769231,-0.415384615384615,-0.4,-0.384615384615385,-0.369230769230769,
-0.353846153846154,-0.338461538461538,-0.323076923076923,-0.307692307692308,
-0.292307692307692,-0.276923076923077,-0.261538461538462,-0.246153846153846,
-0.230769230769231,-0.215384615384615,-0.2,-0.184615384615385,-0.169230769230769,
-0.153846153846154,-0.138461538461538,-0.123076923076923,-0.107692307692308,
-0.0923076923076923,-0.0769230769230769,-0.0615384615384615,-0.0461538461538462,
-0.0307692307692308,-0.0153846153846154,0.),(-1.,1.),.UNSPECIFIED.)
GEOMETRIC_REPRESENTATION_ITEM()
RATIONAL_B_SPLINE_SURFACE(((1.,1.),(1.,1.),(1.,1.),(1.,1.),(1.,1.),(1.,
1.),(1.,1.),(1.,1.),(1.,1.),(1.,1.),(1.,1.),(1.,1.),(1.,1.),(1.,1.),(1.,
1.),(1.,1.),(1.,1.),(1.,1.),(1.,1.),(1.,1.),(1.,1.),(1.,1.),(1.,1.),(1.,
1.),(1.,1.),(1.,1.),(1.,1.),(1.,1.),(1.,1.),(1.,1.),(1.,1.),(1.,1.),(1.,
1.),(1.,1.),(1.,1.),(1.,1.),(1.,1.),(1.,1.),(1.,1.),(1.,1.),(1.,1.),(1.,
1.),(1.,1.),(1.,1.),(1.,1.),(1.,1.),(1.,1.),(1.,1.),(1.,1.),(1.,1.),(1.,
1.),(1.,1.),(1.,1.),(1.,1.),(1.,1.),(1.,1.),(1.,1.),(1.,1.),(1.,1.),(1.,
1.),(1.,1.),(1.,1.),(1.,1.),(1.,1.),(1.,1.),(1.,1.),(1.,1.),(1.,1.),(1.,
1.),(1.,1.)))
REPRESENTATION_ITEM('')
SURFACE()
);
#30=(
BOUNDED_SURFACE()
B_SPLINE_SURFACE(5,1,((#28421,#28422),(#28423,#28424),(#28425,#28426),(#28427,
#28428),(#28429,#28430),(#28431,#28432),(#28433,#28434),(#28435,#28436),
(#28437,#28438),(#28439,#28440),(#28441,#28442),(#28443,#28444),(#28445,
#28446),(#28447,#28448),(#28449,#28450),(#28451,#28452),(#28453,#28454),
(#28455,#28456),(#28457,#28458),(#28459,#28460),(#28461,#28462),(#28463,
#28464),(#28465,#28466),(#28467,#28468),(#28469,#28470),(#28471,#28472),
(#28473,#28474),(#28475,#28476),(#28477,#28478),(#28479,#28480),(#28481,
#28482),(#28483,#28484),(#28485,#28486),(#28487,#28488),(#28489,#28490),
(#28491,#28492),(#28493,#28494),(#28495,#28496),(#28497,#28498),(#28499,
#28500),(#28501,#28502),(#28503,#28504),(#28505,#28506),(#28507,#28508),
(#28509,#28510),(#28511,#28512),(#28513,#28514),(#28515,#28516),(#28517,
#28518),(#28519,#28520),(#28521,#28522),(#28523,#28524),(#28525,#28526),
(#28527,#28528),(#28529,#28530),(#28531,#28532),(#28533,#28534),(#28535,
#28536),(#28537,#28538),(#28539,#28540),(#28541,#28542),(#28543,#28544),
(#28545,#28546),(#28547,#28548),(#28549,#28550),(#28551,#28552),(#28553,
#28554),(#28555,#28556),(#28557,#28558),(#28559,#28560)),.UNSPECIFIED.,
 .F.,.F.,.F.)
B_SPLINE_SURFACE_WITH_KNOTS((6,1,1,1,1,1,1,1,1,1,1,1,1,1,1,1,1,1,1,1,1,
1,1,1,1,1,1,1,1,1,1,1,1,1,1,1,1,1,1,1,1,1,1,1,1,1,1,1,1,1,1,1,1,1,1,1,1,
1,1,1,1,1,1,1,1,6),(2,2),(-1.,-0.984615384615383,-0.969230769230768,-0.953846153846152,
-0.938461538461537,-0.923076923076922,-0.907692307692306,-0.892307692307691,
-0.876923076923076,-0.86153846153846,-0.846153846153845,-0.83076923076923,
-0.815384615384614,-0.799999999999999,-0.784615384615384,-0.769230769230768,
-0.753846153846153,-0.738461538461538,-0.723076923076922,-0.707692307692307,
-0.692307692307692,-0.676923076923076,-0.661538461538461,-0.646153846153846,
-0.63076923076923,-0.615384615384615,-0.6,-0.584615384615384,-0.569230769230769,
-0.553846153846154,-0.538461538461538,-0.523076923076923,-0.507692307692308,
-0.492307692307692,-0.476923076923077,-0.461538461538462,-0.446153846153846,
-0.430769230769231,-0.415384615384615,-0.4,-0.384615384615385,-0.369230769230769,
-0.353846153846154,-0.338461538461538,-0.323076923076923,-0.307692307692308,
-0.292307692307692,-0.276923076923077,-0.261538461538462,-0.246153846153846,
-0.230769230769231,-0.215384615384615,-0.2,-0.184615384615385,-0.169230769230769,
-0.153846153846154,-0.138461538461538,-0.123076923076923,-0.107692307692308,
-0.0923076923076923,-0.0769230769230769,-0.0615384615384615,-0.0461538461538462,
-0.0307692307692308,-0.0153846153846154,0.),(-1.,1.),.UNSPECIFIED.)
GEOMETRIC_REPRESENTATION_ITEM()
RATIONAL_B_SPLINE_SURFACE(((1.,1.),(1.,1.),(1.,1.),(1.,1.),(1.,1.),(1.,
1.),(1.,1.),(1.,1.),(1.,1.),(1.,1.),(1.,1.),(1.,1.),(1.,1.),(1.,1.),(1.,
1.),(1.,1.),(1.,1.),(1.,1.),(1.,1.),(1.,1.),(1.,1.),(1.,1.),(1.,1.),(1.,
1.),(1.,1.),(1.,1.),(1.,1.),(1.,1.),(1.,1.),(1.,1.),(1.,1.),(1.,1.),(1.,
1.),(1.,1.),(1.,1.),(1.,1.),(1.,1.),(1.,1.),(1.,1.),(1.,1.),(1.,1.),(1.,
1.),(1.,1.),(1.,1.),(1.,1.),(1.,1.),(1.,1.),(1.,1.),(1.,1.),(1.,1.),(1.,
1.),(1.,1.),(1.,1.),(1.,1.),(1.,1.),(1.,1.),(1.,1.),(1.,1.),(1.,1.),(1.,
1.),(1.,1.),(1.,1.),(1.,1.),(1.,1.),(1.,1.),(1.,1.),(1.,1.),(1.,1.),(1.,
1.),(1.,1.)))
REPRESENTATION_ITEM('')
SURFACE()
);
#31=(
BOUNDED_SURFACE()
B_SPLINE_SURFACE(5,1,((#28637,#28638),(#28639,#28640),(#28641,#28642),(#28643,
#28644),(#28645,#28646),(#28647,#28648),(#28649,#28650),(#28651,#28652),
(#28653,#28654),(#28655,#28656),(#28657,#28658),(#28659,#28660),(#28661,
#28662),(#28663,#28664),(#28665,#28666),(#28667,#28668),(#28669,#28670),
(#28671,#28672),(#28673,#28674),(#28675,#28676),(#28677,#28678),(#28679,
#28680),(#28681,#28682),(#28683,#28684),(#28685,#28686),(#28687,#28688),
(#28689,#28690),(#28691,#28692),(#28693,#28694),(#28695,#28696),(#28697,
#28698),(#28699,#28700),(#28701,#28702),(#28703,#28704),(#28705,#28706),
(#28707,#28708),(#28709,#28710),(#28711,#28712),(#28713,#28714),(#28715,
#28716),(#28717,#28718),(#28719,#28720),(#28721,#28722),(#28723,#28724),
(#28725,#28726),(#28727,#28728),(#28729,#28730),(#28731,#28732),(#28733,
#28734),(#28735,#28736),(#28737,#28738),(#28739,#28740),(#28741,#28742),
(#28743,#28744),(#28745,#28746),(#28747,#28748),(#28749,#28750),(#28751,
#28752),(#28753,#28754),(#28755,#28756),(#28757,#28758),(#28759,#28760),
(#28761,#28762),(#28763,#28764),(#28765,#28766),(#28767,#28768),(#28769,
#28770),(#28771,#28772),(#28773,#28774),(#28775,#28776)),.UNSPECIFIED.,
 .F.,.F.,.F.)
B_SPLINE_SURFACE_WITH_KNOTS((6,1,1,1,1,1,1,1,1,1,1,1,1,1,1,1,1,1,1,1,1,
1,1,1,1,1,1,1,1,1,1,1,1,1,1,1,1,1,1,1,1,1,1,1,1,1,1,1,1,1,1,1,1,1,1,1,1,
1,1,1,1,1,1,1,1,6),(2,2),(-1.,-0.984615384615383,-0.969230769230768,-0.953846153846152,
-0.938461538461537,-0.923076923076922,-0.907692307692306,-0.892307692307691,
-0.876923076923076,-0.86153846153846,-0.846153846153845,-0.83076923076923,
-0.815384615384614,-0.799999999999999,-0.784615384615384,-0.769230769230768,
-0.753846153846153,-0.738461538461538,-0.723076923076922,-0.707692307692307,
-0.692307692307692,-0.676923076923076,-0.661538461538461,-0.646153846153846,
-0.63076923076923,-0.615384615384615,-0.6,-0.584615384615384,-0.569230769230769,
-0.553846153846154,-0.538461538461538,-0.523076923076923,-0.507692307692308,
-0.492307692307692,-0.476923076923077,-0.461538461538462,-0.446153846153846,
-0.430769230769231,-0.415384615384615,-0.4,-0.384615384615385,-0.369230769230769,
-0.353846153846154,-0.338461538461538,-0.323076923076923,-0.307692307692308,
-0.292307692307692,-0.276923076923077,-0.261538461538462,-0.246153846153846,
-0.230769230769231,-0.215384615384615,-0.2,-0.184615384615385,-0.169230769230769,
-0.153846153846154,-0.138461538461538,-0.123076923076923,-0.107692307692308,
-0.0923076923076923,-0.0769230769230769,-0.0615384615384615,-0.0461538461538462,
-0.0307692307692308,-0.0153846153846154,0.),(-1.,1.),.UNSPECIFIED.)
GEOMETRIC_REPRESENTATION_ITEM()
RATIONAL_B_SPLINE_SURFACE(((1.,1.),(1.,1.),(1.,1.),(1.,1.),(1.,1.),(1.,
1.),(1.,1.),(1.,1.),(1.,1.),(1.,1.),(1.,1.),(1.,1.),(1.,1.),(1.,1.),(1.,
1.),(1.,1.),(1.,1.),(1.,1.),(1.,1.),(1.,1.),(1.,1.),(1.,1.),(1.,1.),(1.,
1.),(1.,1.),(1.,1.),(1.,1.),(1.,1.),(1.,1.),(1.,1.),(1.,1.),(1.,1.),(1.,
1.),(1.,1.),(1.,1.),(1.,1.),(1.,1.),(1.,1.),(1.,1.),(1.,1.),(1.,1.),(1.,
1.),(1.,1.),(1.,1.),(1.,1.),(1.,1.),(1.,1.),(1.,1.),(1.,1.),(1.,1.),(1.,
1.),(1.,1.),(1.,1.),(1.,1.),(1.,1.),(1.,1.),(1.,1.),(1.,1.),(1.,1.),(1.,
1.),(1.,1.),(1.,1.),(1.,1.),(1.,1.),(1.,1.),(1.,1.),(1.,1.),(1.,1.),(1.,
1.),(1.,1.)))
REPRESENTATION_ITEM('')
SURFACE()
);
#32=(
BOUNDED_SURFACE()
B_SPLINE_SURFACE(5,1,((#28853,#28854),(#28855,#28856),(#28857,#28858),(#28859,
#28860),(#28861,#28862),(#28863,#28864),(#28865,#28866),(#28867,#28868),
(#28869,#28870),(#28871,#28872),(#28873,#28874),(#28875,#28876),(#28877,
#28878),(#28879,#28880),(#28881,#28882),(#28883,#28884),(#28885,#28886),
(#28887,#28888),(#28889,#28890),(#28891,#28892),(#28893,#28894),(#28895,
#28896),(#28897,#28898),(#28899,#28900),(#28901,#28902),(#28903,#28904),
(#28905,#28906),(#28907,#28908),(#28909,#28910),(#28911,#28912),(#28913,
#28914),(#28915,#28916),(#28917,#28918),(#28919,#28920),(#28921,#28922),
(#28923,#28924),(#28925,#28926),(#28927,#28928),(#28929,#28930),(#28931,
#28932),(#28933,#28934),(#28935,#28936),(#28937,#28938),(#28939,#28940),
(#28941,#28942),(#28943,#28944),(#28945,#28946),(#28947,#28948),(#28949,
#28950),(#28951,#28952),(#28953,#28954),(#28955,#28956),(#28957,#28958),
(#28959,#28960),(#28961,#28962),(#28963,#28964),(#28965,#28966),(#28967,
#28968),(#28969,#28970),(#28971,#28972),(#28973,#28974),(#28975,#28976),
(#28977,#28978),(#28979,#28980),(#28981,#28982),(#28983,#28984),(#28985,
#28986),(#28987,#28988),(#28989,#28990),(#28991,#28992)),.UNSPECIFIED.,
 .F.,.F.,.F.)
B_SPLINE_SURFACE_WITH_KNOTS((6,1,1,1,1,1,1,1,1,1,1,1,1,1,1,1,1,1,1,1,1,
1,1,1,1,1,1,1,1,1,1,1,1,1,1,1,1,1,1,1,1,1,1,1,1,1,1,1,1,1,1,1,1,1,1,1,1,
1,1,1,1,1,1,1,1,6),(2,2),(-1.,-0.984615384615383,-0.969230769230768,-0.953846153846152,
-0.938461538461537,-0.923076923076922,-0.907692307692306,-0.892307692307691,
-0.876923076923076,-0.86153846153846,-0.846153846153845,-0.83076923076923,
-0.815384615384614,-0.799999999999999,-0.784615384615384,-0.769230769230768,
-0.753846153846153,-0.738461538461538,-0.723076923076922,-0.707692307692307,
-0.692307692307692,-0.676923076923076,-0.661538461538461,-0.646153846153846,
-0.63076923076923,-0.615384615384615,-0.6,-0.584615384615384,-0.569230769230769,
-0.553846153846154,-0.538461538461538,-0.523076923076923,-0.507692307692308,
-0.492307692307692,-0.476923076923077,-0.461538461538462,-0.446153846153846,
-0.430769230769231,-0.415384615384615,-0.4,-0.384615384615385,-0.369230769230769,
-0.353846153846154,-0.338461538461538,-0.323076923076923,-0.307692307692308,
-0.292307692307692,-0.276923076923077,-0.261538461538462,-0.246153846153846,
-0.230769230769231,-0.215384615384615,-0.2,-0.184615384615385,-0.169230769230769,
-0.153846153846154,-0.138461538461538,-0.123076923076923,-0.107692307692308,
-0.0923076923076923,-0.0769230769230769,-0.0615384615384615,-0.0461538461538462,
-0.0307692307692308,-0.0153846153846154,0.),(-1.,1.),.UNSPECIFIED.)
GEOMETRIC_REPRESENTATION_ITEM()
RATIONAL_B_SPLINE_SURFACE(((1.,1.),(1.,1.),(1.,1.),(1.,1.),(1.,1.),(1.,
1.),(1.,1.),(1.,1.),(1.,1.),(1.,1.),(1.,1.),(1.,1.),(1.,1.),(1.,1.),(1.,
1.),(1.,1.),(1.,1.),(1.,1.),(1.,1.),(1.,1.),(1.,1.),(1.,1.),(1.,1.),(1.,
1.),(1.,1.),(1.,1.),(1.,1.),(1.,1.),(1.,1.),(1.,1.),(1.,1.),(1.,1.),(1.,
1.),(1.,1.),(1.,1.),(1.,1.),(1.,1.),(1.,1.),(1.,1.),(1.,1.),(1.,1.),(1.,
1.),(1.,1.),(1.,1.),(1.,1.),(1.,1.),(1.,1.),(1.,1.),(1.,1.),(1.,1.),(1.,
1.),(1.,1.),(1.,1.),(1.,1.),(1.,1.),(1.,1.),(1.,1.),(1.,1.),(1.,1.),(1.,
1.),(1.,1.),(1.,1.),(1.,1.),(1.,1.),(1.,1.),(1.,1.),(1.,1.),(1.,1.),(1.,
1.),(1.,1.)))
REPRESENTATION_ITEM('')
SURFACE()
);
#33=(
BOUNDED_SURFACE()
B_SPLINE_SURFACE(5,1,((#29069,#29070),(#29071,#29072),(#29073,#29074),(#29075,
#29076),(#29077,#29078),(#29079,#29080),(#29081,#29082),(#29083,#29084),
(#29085,#29086),(#29087,#29088),(#29089,#29090),(#29091,#29092),(#29093,
#29094),(#29095,#29096),(#29097,#29098),(#29099,#29100),(#29101,#29102),
(#29103,#29104),(#29105,#29106),(#29107,#29108),(#29109,#29110),(#29111,
#29112),(#29113,#29114),(#29115,#29116),(#29117,#29118),(#29119,#29120),
(#29121,#29122),(#29123,#29124),(#29125,#29126),(#29127,#29128),(#29129,
#29130),(#29131,#29132),(#29133,#29134),(#29135,#29136),(#29137,#29138),
(#29139,#29140),(#29141,#29142),(#29143,#29144),(#29145,#29146),(#29147,
#29148),(#29149,#29150),(#29151,#29152),(#29153,#29154),(#29155,#29156),
(#29157,#29158),(#29159,#29160),(#29161,#29162),(#29163,#29164),(#29165,
#29166),(#29167,#29168),(#29169,#29170),(#29171,#29172),(#29173,#29174),
(#29175,#29176),(#29177,#29178),(#29179,#29180),(#29181,#29182),(#29183,
#29184),(#29185,#29186),(#29187,#29188),(#29189,#29190),(#29191,#29192),
(#29193,#29194),(#29195,#29196),(#29197,#29198),(#29199,#29200),(#29201,
#29202),(#29203,#29204),(#29205,#29206),(#29207,#29208)),.UNSPECIFIED.,
 .F.,.F.,.F.)
B_SPLINE_SURFACE_WITH_KNOTS((6,1,1,1,1,1,1,1,1,1,1,1,1,1,1,1,1,1,1,1,1,
1,1,1,1,1,1,1,1,1,1,1,1,1,1,1,1,1,1,1,1,1,1,1,1,1,1,1,1,1,1,1,1,1,1,1,1,
1,1,1,1,1,1,1,1,6),(2,2),(-1.,-0.984615384615383,-0.969230769230768,-0.953846153846152,
-0.938461538461537,-0.923076923076922,-0.907692307692306,-0.892307692307691,
-0.876923076923076,-0.86153846153846,-0.846153846153845,-0.83076923076923,
-0.815384615384614,-0.799999999999999,-0.784615384615384,-0.769230769230768,
-0.753846153846153,-0.738461538461538,-0.723076923076922,-0.707692307692307,
-0.692307692307692,-0.676923076923076,-0.661538461538461,-0.646153846153846,
-0.63076923076923,-0.615384615384615,-0.6,-0.584615384615384,-0.569230769230769,
-0.553846153846154,-0.538461538461538,-0.523076923076923,-0.507692307692308,
-0.492307692307692,-0.476923076923077,-0.461538461538462,-0.446153846153846,
-0.430769230769231,-0.415384615384615,-0.4,-0.384615384615385,-0.369230769230769,
-0.353846153846154,-0.338461538461538,-0.323076923076923,-0.307692307692308,
-0.292307692307692,-0.276923076923077,-0.261538461538462,-0.246153846153846,
-0.230769230769231,-0.215384615384615,-0.2,-0.184615384615385,-0.169230769230769,
-0.153846153846154,-0.138461538461538,-0.123076923076923,-0.107692307692308,
-0.0923076923076923,-0.0769230769230769,-0.0615384615384615,-0.0461538461538462,
-0.0307692307692308,-0.0153846153846154,0.),(-1.,1.),.UNSPECIFIED.)
GEOMETRIC_REPRESENTATION_ITEM()
RATIONAL_B_SPLINE_SURFACE(((1.,1.),(1.,1.),(1.,1.),(1.,1.),(1.,1.),(1.,
1.),(1.,1.),(1.,1.),(1.,1.),(1.,1.),(1.,1.),(1.,1.),(1.,1.),(1.,1.),(1.,
1.),(1.,1.),(1.,1.),(1.,1.),(1.,1.),(1.,1.),(1.,1.),(1.,1.),(1.,1.),(1.,
1.),(1.,1.),(1.,1.),(1.,1.),(1.,1.),(1.,1.),(1.,1.),(1.,1.),(1.,1.),(1.,
1.),(1.,1.),(1.,1.),(1.,1.),(1.,1.),(1.,1.),(1.,1.),(1.,1.),(1.,1.),(1.,
1.),(1.,1.),(1.,1.),(1.,1.),(1.,1.),(1.,1.),(1.,1.),(1.,1.),(1.,1.),(1.,
1.),(1.,1.),(1.,1.),(1.,1.),(1.,1.),(1.,1.),(1.,1.),(1.,1.),(1.,1.),(1.,
1.),(1.,1.),(1.,1.),(1.,1.),(1.,1.),(1.,1.),(1.,1.),(1.,1.),(1.,1.),(1.,
1.),(1.,1.)))
REPRESENTATION_ITEM('')
SURFACE()
);
#34=(
BOUNDED_SURFACE()
B_SPLINE_SURFACE(5,1,((#29285,#29286),(#29287,#29288),(#29289,#29290),(#29291,
#29292),(#29293,#29294),(#29295,#29296),(#29297,#29298),(#29299,#29300),
(#29301,#29302),(#29303,#29304),(#29305,#29306),(#29307,#29308),(#29309,
#29310),(#29311,#29312),(#29313,#29314),(#29315,#29316),(#29317,#29318),
(#29319,#29320),(#29321,#29322),(#29323,#29324),(#29325,#29326),(#29327,
#29328),(#29329,#29330),(#29331,#29332),(#29333,#29334),(#29335,#29336),
(#29337,#29338),(#29339,#29340),(#29341,#29342),(#29343,#29344),(#29345,
#29346),(#29347,#29348),(#29349,#29350),(#29351,#29352),(#29353,#29354),
(#29355,#29356),(#29357,#29358),(#29359,#29360),(#29361,#29362),(#29363,
#29364),(#29365,#29366),(#29367,#29368),(#29369,#29370),(#29371,#29372),
(#29373,#29374),(#29375,#29376),(#29377,#29378),(#29379,#29380),(#29381,
#29382),(#29383,#29384),(#29385,#29386),(#29387,#29388),(#29389,#29390),
(#29391,#29392),(#29393,#29394),(#29395,#29396),(#29397,#29398),(#29399,
#29400),(#29401,#29402),(#29403,#29404),(#29405,#29406),(#29407,#29408),
(#29409,#29410),(#29411,#29412),(#29413,#29414),(#29415,#29416),(#29417,
#29418),(#29419,#29420),(#29421,#29422),(#29423,#29424)),.UNSPECIFIED.,
 .F.,.F.,.F.)
B_SPLINE_SURFACE_WITH_KNOTS((6,1,1,1,1,1,1,1,1,1,1,1,1,1,1,1,1,1,1,1,1,
1,1,1,1,1,1,1,1,1,1,1,1,1,1,1,1,1,1,1,1,1,1,1,1,1,1,1,1,1,1,1,1,1,1,1,1,
1,1,1,1,1,1,1,1,6),(2,2),(-1.,-0.984615384615383,-0.969230769230768,-0.953846153846152,
-0.938461538461537,-0.923076923076922,-0.907692307692306,-0.892307692307691,
-0.876923076923076,-0.86153846153846,-0.846153846153845,-0.83076923076923,
-0.815384615384614,-0.799999999999999,-0.784615384615384,-0.769230769230768,
-0.753846153846153,-0.738461538461538,-0.723076923076922,-0.707692307692307,
-0.692307692307692,-0.676923076923076,-0.661538461538461,-0.646153846153846,
-0.63076923076923,-0.615384615384615,-0.6,-0.584615384615384,-0.569230769230769,
-0.553846153846154,-0.538461538461538,-0.523076923076923,-0.507692307692308,
-0.492307692307692,-0.476923076923077,-0.461538461538462,-0.446153846153846,
-0.430769230769231,-0.415384615384615,-0.4,-0.384615384615385,-0.369230769230769,
-0.353846153846154,-0.338461538461538,-0.323076923076923,-0.307692307692308,
-0.292307692307692,-0.276923076923077,-0.261538461538462,-0.246153846153846,
-0.230769230769231,-0.215384615384615,-0.2,-0.184615384615385,-0.169230769230769,
-0.153846153846154,-0.138461538461538,-0.123076923076923,-0.107692307692308,
-0.0923076923076923,-0.0769230769230769,-0.0615384615384615,-0.0461538461538462,
-0.0307692307692308,-0.0153846153846154,0.),(-1.,1.),.UNSPECIFIED.)
GEOMETRIC_REPRESENTATION_ITEM()
RATIONAL_B_SPLINE_SURFACE(((1.,1.),(1.,1.),(1.,1.),(1.,1.),(1.,1.),(1.,
1.),(1.,1.),(1.,1.),(1.,1.),(1.,1.),(1.,1.),(1.,1.),(1.,1.),(1.,1.),(1.,
1.),(1.,1.),(1.,1.),(1.,1.),(1.,1.),(1.,1.),(1.,1.),(1.,1.),(1.,1.),(1.,
1.),(1.,1.),(1.,1.),(1.,1.),(1.,1.),(1.,1.),(1.,1.),(1.,1.),(1.,1.),(1.,
1.),(1.,1.),(1.,1.),(1.,1.),(1.,1.),(1.,1.),(1.,1.),(1.,1.),(1.,1.),(1.,
1.),(1.,1.),(1.,1.),(1.,1.),(1.,1.),(1.,1.),(1.,1.),(1.,1.),(1.,1.),(1.,
1.),(1.,1.),(1.,1.),(1.,1.),(1.,1.),(1.,1.),(1.,1.),(1.,1.),(1.,1.),(1.,
1.),(1.,1.),(1.,1.),(1.,1.),(1.,1.),(1.,1.),(1.,1.),(1.,1.),(1.,1.),(1.,
1.),(1.,1.)))
REPRESENTATION_ITEM('')
SURFACE()
);
#35=(
BOUNDED_SURFACE()
B_SPLINE_SURFACE(5,1,((#29501,#29502),(#29503,#29504),(#29505,#29506),(#29507,
#29508),(#29509,#29510),(#29511,#29512),(#29513,#29514),(#29515,#29516),
(#29517,#29518),(#29519,#29520),(#29521,#29522),(#29523,#29524),(#29525,
#29526),(#29527,#29528),(#29529,#29530),(#29531,#29532),(#29533,#29534),
(#29535,#29536),(#29537,#29538),(#29539,#29540),(#29541,#29542),(#29543,
#29544),(#29545,#29546),(#29547,#29548),(#29549,#29550),(#29551,#29552),
(#29553,#29554),(#29555,#29556),(#29557,#29558),(#29559,#29560),(#29561,
#29562),(#29563,#29564),(#29565,#29566),(#29567,#29568),(#29569,#29570),
(#29571,#29572),(#29573,#29574),(#29575,#29576),(#29577,#29578),(#29579,
#29580),(#29581,#29582),(#29583,#29584),(#29585,#29586),(#29587,#29588),
(#29589,#29590),(#29591,#29592),(#29593,#29594),(#29595,#29596),(#29597,
#29598),(#29599,#29600),(#29601,#29602),(#29603,#29604),(#29605,#29606),
(#29607,#29608),(#29609,#29610),(#29611,#29612),(#29613,#29614),(#29615,
#29616),(#29617,#29618),(#29619,#29620),(#29621,#29622),(#29623,#29624),
(#29625,#29626),(#29627,#29628),(#29629,#29630),(#29631,#29632),(#29633,
#29634),(#29635,#29636),(#29637,#29638),(#29639,#29640)),.UNSPECIFIED.,
 .F.,.F.,.F.)
B_SPLINE_SURFACE_WITH_KNOTS((6,1,1,1,1,1,1,1,1,1,1,1,1,1,1,1,1,1,1,1,1,
1,1,1,1,1,1,1,1,1,1,1,1,1,1,1,1,1,1,1,1,1,1,1,1,1,1,1,1,1,1,1,1,1,1,1,1,
1,1,1,1,1,1,1,1,6),(2,2),(-1.,-0.984615384615383,-0.969230769230768,-0.953846153846152,
-0.938461538461537,-0.923076923076922,-0.907692307692306,-0.892307692307691,
-0.876923076923076,-0.86153846153846,-0.846153846153845,-0.83076923076923,
-0.815384615384614,-0.799999999999999,-0.784615384615384,-0.769230769230768,
-0.753846153846153,-0.738461538461538,-0.723076923076922,-0.707692307692307,
-0.692307692307692,-0.676923076923076,-0.661538461538461,-0.646153846153846,
-0.63076923076923,-0.615384615384615,-0.6,-0.584615384615384,-0.569230769230769,
-0.553846153846154,-0.538461538461538,-0.523076923076923,-0.507692307692308,
-0.492307692307692,-0.476923076923077,-0.461538461538462,-0.446153846153846,
-0.430769230769231,-0.415384615384615,-0.4,-0.384615384615385,-0.369230769230769,
-0.353846153846154,-0.338461538461538,-0.323076923076923,-0.307692307692308,
-0.292307692307692,-0.276923076923077,-0.261538461538462,-0.246153846153846,
-0.230769230769231,-0.215384615384615,-0.2,-0.184615384615385,-0.169230769230769,
-0.153846153846154,-0.138461538461538,-0.123076923076923,-0.107692307692308,
-0.0923076923076923,-0.0769230769230769,-0.0615384615384615,-0.0461538461538462,
-0.0307692307692308,-0.0153846153846154,0.),(-1.,1.),.UNSPECIFIED.)
GEOMETRIC_REPRESENTATION_ITEM()
RATIONAL_B_SPLINE_SURFACE(((1.,1.),(1.,1.),(1.,1.),(1.,1.),(1.,1.),(1.,
1.),(1.,1.),(1.,1.),(1.,1.),(1.,1.),(1.,1.),(1.,1.),(1.,1.),(1.,1.),(1.,
1.),(1.,1.),(1.,1.),(1.,1.),(1.,1.),(1.,1.),(1.,1.),(1.,1.),(1.,1.),(1.,
1.),(1.,1.),(1.,1.),(1.,1.),(1.,1.),(1.,1.),(1.,1.),(1.,1.),(1.,1.),(1.,
1.),(1.,1.),(1.,1.),(1.,1.),(1.,1.),(1.,1.),(1.,1.),(1.,1.),(1.,1.),(1.,
1.),(1.,1.),(1.,1.),(1.,1.),(1.,1.),(1.,1.),(1.,1.),(1.,1.),(1.,1.),(1.,
1.),(1.,1.),(1.,1.),(1.,1.),(1.,1.),(1.,1.),(1.,1.),(1.,1.),(1.,1.),(1.,
1.),(1.,1.),(1.,1.),(1.,1.),(1.,1.),(1.,1.),(1.,1.),(1.,1.),(1.,1.),(1.,
1.),(1.,1.)))
REPRESENTATION_ITEM('')
SURFACE()
);
#36=(
BOUNDED_SURFACE()
B_SPLINE_SURFACE(5,1,((#29717,#29718),(#29719,#29720),(#29721,#29722),(#29723,
#29724),(#29725,#29726),(#29727,#29728),(#29729,#29730),(#29731,#29732),
(#29733,#29734),(#29735,#29736),(#29737,#29738),(#29739,#29740),(#29741,
#29742),(#29743,#29744),(#29745,#29746),(#29747,#29748),(#29749,#29750),
(#29751,#29752),(#29753,#29754),(#29755,#29756),(#29757,#29758),(#29759,
#29760),(#29761,#29762),(#29763,#29764),(#29765,#29766),(#29767,#29768),
(#29769,#29770),(#29771,#29772),(#29773,#29774),(#29775,#29776),(#29777,
#29778),(#29779,#29780),(#29781,#29782),(#29783,#29784),(#29785,#29786),
(#29787,#29788),(#29789,#29790),(#29791,#29792),(#29793,#29794),(#29795,
#29796),(#29797,#29798),(#29799,#29800),(#29801,#29802),(#29803,#29804),
(#29805,#29806),(#29807,#29808),(#29809,#29810),(#29811,#29812),(#29813,
#29814),(#29815,#29816),(#29817,#29818),(#29819,#29820),(#29821,#29822),
(#29823,#29824),(#29825,#29826),(#29827,#29828),(#29829,#29830),(#29831,
#29832),(#29833,#29834),(#29835,#29836),(#29837,#29838),(#29839,#29840),
(#29841,#29842),(#29843,#29844),(#29845,#29846),(#29847,#29848),(#29849,
#29850),(#29851,#29852),(#29853,#29854),(#29855,#29856)),.UNSPECIFIED.,
 .F.,.F.,.F.)
B_SPLINE_SURFACE_WITH_KNOTS((6,1,1,1,1,1,1,1,1,1,1,1,1,1,1,1,1,1,1,1,1,
1,1,1,1,1,1,1,1,1,1,1,1,1,1,1,1,1,1,1,1,1,1,1,1,1,1,1,1,1,1,1,1,1,1,1,1,
1,1,1,1,1,1,1,1,6),(2,2),(-1.,-0.984615384615383,-0.969230769230768,-0.953846153846152,
-0.938461538461537,-0.923076923076922,-0.907692307692306,-0.892307692307691,
-0.876923076923076,-0.86153846153846,-0.846153846153845,-0.83076923076923,
-0.815384615384614,-0.799999999999999,-0.784615384615384,-0.769230769230768,
-0.753846153846153,-0.738461538461538,-0.723076923076922,-0.707692307692307,
-0.692307692307692,-0.676923076923076,-0.661538461538461,-0.646153846153846,
-0.63076923076923,-0.615384615384615,-0.6,-0.584615384615384,-0.569230769230769,
-0.553846153846154,-0.538461538461538,-0.523076923076923,-0.507692307692308,
-0.492307692307692,-0.476923076923077,-0.461538461538462,-0.446153846153846,
-0.430769230769231,-0.415384615384615,-0.4,-0.384615384615385,-0.369230769230769,
-0.353846153846154,-0.338461538461538,-0.323076923076923,-0.307692307692308,
-0.292307692307692,-0.276923076923077,-0.261538461538462,-0.246153846153846,
-0.230769230769231,-0.215384615384615,-0.2,-0.184615384615385,-0.169230769230769,
-0.153846153846154,-0.138461538461538,-0.123076923076923,-0.107692307692308,
-0.0923076923076923,-0.0769230769230769,-0.0615384615384615,-0.0461538461538462,
-0.0307692307692308,-0.0153846153846154,0.),(-1.,1.),.UNSPECIFIED.)
GEOMETRIC_REPRESENTATION_ITEM()
RATIONAL_B_SPLINE_SURFACE(((1.,1.),(1.,1.),(1.,1.),(1.,1.),(1.,1.),(1.,
1.),(1.,1.),(1.,1.),(1.,1.),(1.,1.),(1.,1.),(1.,1.),(1.,1.),(1.,1.),(1.,
1.),(1.,1.),(1.,1.),(1.,1.),(1.,1.),(1.,1.),(1.,1.),(1.,1.),(1.,1.),(1.,
1.),(1.,1.),(1.,1.),(1.,1.),(1.,1.),(1.,1.),(1.,1.),(1.,1.),(1.,1.),(1.,
1.),(1.,1.),(1.,1.),(1.,1.),(1.,1.),(1.,1.),(1.,1.),(1.,1.),(1.,1.),(1.,
1.),(1.,1.),(1.,1.),(1.,1.),(1.,1.),(1.,1.),(1.,1.),(1.,1.),(1.,1.),(1.,
1.),(1.,1.),(1.,1.),(1.,1.),(1.,1.),(1.,1.),(1.,1.),(1.,1.),(1.,1.),(1.,
1.),(1.,1.),(1.,1.),(1.,1.),(1.,1.),(1.,1.),(1.,1.),(1.,1.),(1.,1.),(1.,
1.),(1.,1.)))
REPRESENTATION_ITEM('')
SURFACE()
);
#37=(
BOUNDED_SURFACE()
B_SPLINE_SURFACE(5,1,((#29933,#29934),(#29935,#29936),(#29937,#29938),(#29939,
#29940),(#29941,#29942),(#29943,#29944),(#29945,#29946),(#29947,#29948),
(#29949,#29950),(#29951,#29952),(#29953,#29954),(#29955,#29956),(#29957,
#29958),(#29959,#29960),(#29961,#29962),(#29963,#29964),(#29965,#29966),
(#29967,#29968),(#29969,#29970),(#29971,#29972),(#29973,#29974),(#29975,
#29976),(#29977,#29978),(#29979,#29980),(#29981,#29982),(#29983,#29984),
(#29985,#29986),(#29987,#29988),(#29989,#29990),(#29991,#29992),(#29993,
#29994),(#29995,#29996),(#29997,#29998),(#29999,#30000),(#30001,#30002),
(#30003,#30004),(#30005,#30006),(#30007,#30008),(#30009,#30010),(#30011,
#30012),(#30013,#30014),(#30015,#30016),(#30017,#30018),(#30019,#30020),
(#30021,#30022),(#30023,#30024),(#30025,#30026),(#30027,#30028),(#30029,
#30030),(#30031,#30032),(#30033,#30034),(#30035,#30036),(#30037,#30038),
(#30039,#30040),(#30041,#30042),(#30043,#30044),(#30045,#30046),(#30047,
#30048),(#30049,#30050),(#30051,#30052),(#30053,#30054),(#30055,#30056),
(#30057,#30058),(#30059,#30060),(#30061,#30062),(#30063,#30064),(#30065,
#30066),(#30067,#30068),(#30069,#30070),(#30071,#30072)),.UNSPECIFIED.,
 .F.,.F.,.F.)
B_SPLINE_SURFACE_WITH_KNOTS((6,1,1,1,1,1,1,1,1,1,1,1,1,1,1,1,1,1,1,1,1,
1,1,1,1,1,1,1,1,1,1,1,1,1,1,1,1,1,1,1,1,1,1,1,1,1,1,1,1,1,1,1,1,1,1,1,1,
1,1,1,1,1,1,1,1,6),(2,2),(-1.,-0.984615384615383,-0.969230769230768,-0.953846153846152,
-0.938461538461537,-0.923076923076922,-0.907692307692306,-0.892307692307691,
-0.876923076923076,-0.86153846153846,-0.846153846153845,-0.83076923076923,
-0.815384615384614,-0.799999999999999,-0.784615384615384,-0.769230769230768,
-0.753846153846153,-0.738461538461538,-0.723076923076922,-0.707692307692307,
-0.692307692307692,-0.676923076923076,-0.661538461538461,-0.646153846153846,
-0.63076923076923,-0.615384615384615,-0.6,-0.584615384615384,-0.569230769230769,
-0.553846153846154,-0.538461538461538,-0.523076923076923,-0.507692307692308,
-0.492307692307692,-0.476923076923077,-0.461538461538462,-0.446153846153846,
-0.430769230769231,-0.415384615384615,-0.4,-0.384615384615385,-0.369230769230769,
-0.353846153846154,-0.338461538461538,-0.323076923076923,-0.307692307692308,
-0.292307692307692,-0.276923076923077,-0.261538461538462,-0.246153846153846,
-0.230769230769231,-0.215384615384615,-0.2,-0.184615384615385,-0.169230769230769,
-0.153846153846154,-0.138461538461538,-0.123076923076923,-0.107692307692308,
-0.0923076923076923,-0.0769230769230769,-0.0615384615384615,-0.0461538461538462,
-0.0307692307692308,-0.0153846153846154,0.),(-1.,1.),.UNSPECIFIED.)
GEOMETRIC_REPRESENTATION_ITEM()
RATIONAL_B_SPLINE_SURFACE(((1.,1.),(1.,1.),(1.,1.),(1.,1.),(1.,1.),(1.,
1.),(1.,1.),(1.,1.),(1.,1.),(1.,1.),(1.,1.),(1.,1.),(1.,1.),(1.,1.),(1.,
1.),(1.,1.),(1.,1.),(1.,1.),(1.,1.),(1.,1.),(1.,1.),(1.,1.),(1.,1.),(1.,
1.),(1.,1.),(1.,1.),(1.,1.),(1.,1.),(1.,1.),(1.,1.),(1.,1.),(1.,1.),(1.,
1.),(1.,1.),(1.,1.),(1.,1.),(1.,1.),(1.,1.),(1.,1.),(1.,1.),(1.,1.),(1.,
1.),(1.,1.),(1.,1.),(1.,1.),(1.,1.),(1.,1.),(1.,1.),(1.,1.),(1.,1.),(1.,
1.),(1.,1.),(1.,1.),(1.,1.),(1.,1.),(1.,1.),(1.,1.),(1.,1.),(1.,1.),(1.,
1.),(1.,1.),(1.,1.),(1.,1.),(1.,1.),(1.,1.),(1.,1.),(1.,1.),(1.,1.),(1.,
1.),(1.,1.)))
REPRESENTATION_ITEM('')
SURFACE()
);
#38=(
BOUNDED_SURFACE()
B_SPLINE_SURFACE(5,1,((#30149,#30150),(#30151,#30152),(#30153,#30154),(#30155,
#30156),(#30157,#30158),(#30159,#30160),(#30161,#30162),(#30163,#30164),
(#30165,#30166),(#30167,#30168),(#30169,#30170),(#30171,#30172),(#30173,
#30174),(#30175,#30176),(#30177,#30178),(#30179,#30180),(#30181,#30182),
(#30183,#30184),(#30185,#30186),(#30187,#30188),(#30189,#30190),(#30191,
#30192),(#30193,#30194),(#30195,#30196),(#30197,#30198),(#30199,#30200),
(#30201,#30202),(#30203,#30204),(#30205,#30206),(#30207,#30208),(#30209,
#30210),(#30211,#30212),(#30213,#30214),(#30215,#30216),(#30217,#30218),
(#30219,#30220),(#30221,#30222),(#30223,#30224),(#30225,#30226),(#30227,
#30228),(#30229,#30230),(#30231,#30232),(#30233,#30234),(#30235,#30236),
(#30237,#30238),(#30239,#30240),(#30241,#30242),(#30243,#30244),(#30245,
#30246),(#30247,#30248),(#30249,#30250),(#30251,#30252),(#30253,#30254),
(#30255,#30256),(#30257,#30258),(#30259,#30260),(#30261,#30262),(#30263,
#30264),(#30265,#30266),(#30267,#30268),(#30269,#30270),(#30271,#30272),
(#30273,#30274),(#30275,#30276),(#30277,#30278),(#30279,#30280),(#30281,
#30282),(#30283,#30284),(#30285,#30286),(#30287,#30288)),.UNSPECIFIED.,
 .F.,.F.,.F.)
B_SPLINE_SURFACE_WITH_KNOTS((6,1,1,1,1,1,1,1,1,1,1,1,1,1,1,1,1,1,1,1,1,
1,1,1,1,1,1,1,1,1,1,1,1,1,1,1,1,1,1,1,1,1,1,1,1,1,1,1,1,1,1,1,1,1,1,1,1,
1,1,1,1,1,1,1,1,6),(2,2),(-1.,-0.984615384615383,-0.969230769230768,-0.953846153846152,
-0.938461538461537,-0.923076923076922,-0.907692307692306,-0.892307692307691,
-0.876923076923076,-0.86153846153846,-0.846153846153845,-0.83076923076923,
-0.815384615384614,-0.799999999999999,-0.784615384615384,-0.769230769230768,
-0.753846153846153,-0.738461538461538,-0.723076923076922,-0.707692307692307,
-0.692307692307692,-0.676923076923076,-0.661538461538461,-0.646153846153846,
-0.63076923076923,-0.615384615384615,-0.6,-0.584615384615384,-0.569230769230769,
-0.553846153846154,-0.538461538461538,-0.523076923076923,-0.507692307692308,
-0.492307692307692,-0.476923076923077,-0.461538461538462,-0.446153846153846,
-0.430769230769231,-0.415384615384615,-0.4,-0.384615384615385,-0.369230769230769,
-0.353846153846154,-0.338461538461538,-0.323076923076923,-0.307692307692308,
-0.292307692307692,-0.276923076923077,-0.261538461538462,-0.246153846153846,
-0.230769230769231,-0.215384615384615,-0.2,-0.184615384615385,-0.169230769230769,
-0.153846153846154,-0.138461538461538,-0.123076923076923,-0.107692307692308,
-0.0923076923076923,-0.0769230769230769,-0.0615384615384615,-0.0461538461538462,
-0.0307692307692308,-0.0153846153846154,0.),(-1.,1.),.UNSPECIFIED.)
GEOMETRIC_REPRESENTATION_ITEM()
RATIONAL_B_SPLINE_SURFACE(((1.,1.),(1.,1.),(1.,1.),(1.,1.),(1.,1.),(1.,
1.),(1.,1.),(1.,1.),(1.,1.),(1.,1.),(1.,1.),(1.,1.),(1.,1.),(1.,1.),(1.,
1.),(1.,1.),(1.,1.),(1.,1.),(1.,1.),(1.,1.),(1.,1.),(1.,1.),(1.,1.),(1.,
1.),(1.,1.),(1.,1.),(1.,1.),(1.,1.),(1.,1.),(1.,1.),(1.,1.),(1.,1.),(1.,
1.),(1.,1.),(1.,1.),(1.,1.),(1.,1.),(1.,1.),(1.,1.),(1.,1.),(1.,1.),(1.,
1.),(1.,1.),(1.,1.),(1.,1.),(1.,1.),(1.,1.),(1.,1.),(1.,1.),(1.,1.),(1.,
1.),(1.,1.),(1.,1.),(1.,1.),(1.,1.),(1.,1.),(1.,1.),(1.,1.),(1.,1.),(1.,
1.),(1.,1.),(1.,1.),(1.,1.),(1.,1.),(1.,1.),(1.,1.),(1.,1.),(1.,1.),(1.,
1.),(1.,1.)))
REPRESENTATION_ITEM('')
SURFACE()
);
#39=(
BOUNDED_SURFACE()
B_SPLINE_SURFACE(5,1,((#30365,#30366),(#30367,#30368),(#30369,#30370),(#30371,
#30372),(#30373,#30374),(#30375,#30376),(#30377,#30378),(#30379,#30380),
(#30381,#30382),(#30383,#30384),(#30385,#30386),(#30387,#30388),(#30389,
#30390),(#30391,#30392),(#30393,#30394),(#30395,#30396),(#30397,#30398),
(#30399,#30400),(#30401,#30402),(#30403,#30404),(#30405,#30406),(#30407,
#30408),(#30409,#30410),(#30411,#30412),(#30413,#30414),(#30415,#30416),
(#30417,#30418),(#30419,#30420),(#30421,#30422),(#30423,#30424),(#30425,
#30426),(#30427,#30428),(#30429,#30430),(#30431,#30432),(#30433,#30434),
(#30435,#30436),(#30437,#30438),(#30439,#30440),(#30441,#30442),(#30443,
#30444),(#30445,#30446),(#30447,#30448),(#30449,#30450),(#30451,#30452),
(#30453,#30454),(#30455,#30456),(#30457,#30458),(#30459,#30460),(#30461,
#30462),(#30463,#30464),(#30465,#30466),(#30467,#30468),(#30469,#30470),
(#30471,#30472),(#30473,#30474),(#30475,#30476),(#30477,#30478),(#30479,
#30480),(#30481,#30482),(#30483,#30484),(#30485,#30486),(#30487,#30488),
(#30489,#30490),(#30491,#30492),(#30493,#30494),(#30495,#30496),(#30497,
#30498),(#30499,#30500),(#30501,#30502),(#30503,#30504)),.UNSPECIFIED.,
 .F.,.F.,.F.)
B_SPLINE_SURFACE_WITH_KNOTS((6,1,1,1,1,1,1,1,1,1,1,1,1,1,1,1,1,1,1,1,1,
1,1,1,1,1,1,1,1,1,1,1,1,1,1,1,1,1,1,1,1,1,1,1,1,1,1,1,1,1,1,1,1,1,1,1,1,
1,1,1,1,1,1,1,1,6),(2,2),(-1.,-0.984615384615383,-0.969230769230768,-0.953846153846152,
-0.938461538461537,-0.923076923076922,-0.907692307692306,-0.892307692307691,
-0.876923076923076,-0.86153846153846,-0.846153846153845,-0.83076923076923,
-0.815384615384614,-0.799999999999999,-0.784615384615384,-0.769230769230768,
-0.753846153846153,-0.738461538461538,-0.723076923076922,-0.707692307692307,
-0.692307692307692,-0.676923076923076,-0.661538461538461,-0.646153846153846,
-0.63076923076923,-0.615384615384615,-0.6,-0.584615384615384,-0.569230769230769,
-0.553846153846154,-0.538461538461538,-0.523076923076923,-0.507692307692308,
-0.492307692307692,-0.476923076923077,-0.461538461538462,-0.446153846153846,
-0.430769230769231,-0.415384615384615,-0.4,-0.384615384615385,-0.369230769230769,
-0.353846153846154,-0.338461538461538,-0.323076923076923,-0.307692307692308,
-0.292307692307692,-0.276923076923077,-0.261538461538462,-0.246153846153846,
-0.230769230769231,-0.215384615384615,-0.2,-0.184615384615385,-0.169230769230769,
-0.153846153846154,-0.138461538461538,-0.123076923076923,-0.107692307692308,
-0.0923076923076923,-0.0769230769230769,-0.0615384615384615,-0.0461538461538462,
-0.0307692307692308,-0.0153846153846154,0.),(-1.,1.),.UNSPECIFIED.)
GEOMETRIC_REPRESENTATION_ITEM()
RATIONAL_B_SPLINE_SURFACE(((1.,1.),(1.,1.),(1.,1.),(1.,1.),(1.,1.),(1.,
1.),(1.,1.),(1.,1.),(1.,1.),(1.,1.),(1.,1.),(1.,1.),(1.,1.),(1.,1.),(1.,
1.),(1.,1.),(1.,1.),(1.,1.),(1.,1.),(1.,1.),(1.,1.),(1.,1.),(1.,1.),(1.,
1.),(1.,1.),(1.,1.),(1.,1.),(1.,1.),(1.,1.),(1.,1.),(1.,1.),(1.,1.),(1.,
1.),(1.,1.),(1.,1.),(1.,1.),(1.,1.),(1.,1.),(1.,1.),(1.,1.),(1.,1.),(1.,
1.),(1.,1.),(1.,1.),(1.,1.),(1.,1.),(1.,1.),(1.,1.),(1.,1.),(1.,1.),(1.,
1.),(1.,1.),(1.,1.),(1.,1.),(1.,1.),(1.,1.),(1.,1.),(1.,1.),(1.,1.),(1.,
1.),(1.,1.),(1.,1.),(1.,1.),(1.,1.),(1.,1.),(1.,1.),(1.,1.),(1.,1.),(1.,
1.),(1.,1.)))
REPRESENTATION_ITEM('')
SURFACE()
);
#40=(
BOUNDED_SURFACE()
B_SPLINE_SURFACE(5,1,((#30581,#30582),(#30583,#30584),(#30585,#30586),(#30587,
#30588),(#30589,#30590),(#30591,#30592),(#30593,#30594),(#30595,#30596),
(#30597,#30598),(#30599,#30600),(#30601,#30602),(#30603,#30604),(#30605,
#30606),(#30607,#30608),(#30609,#30610),(#30611,#30612),(#30613,#30614),
(#30615,#30616),(#30617,#30618),(#30619,#30620),(#30621,#30622),(#30623,
#30624),(#30625,#30626),(#30627,#30628),(#30629,#30630),(#30631,#30632),
(#30633,#30634),(#30635,#30636),(#30637,#30638),(#30639,#30640),(#30641,
#30642),(#30643,#30644),(#30645,#30646),(#30647,#30648),(#30649,#30650),
(#30651,#30652),(#30653,#30654),(#30655,#30656),(#30657,#30658),(#30659,
#30660),(#30661,#30662),(#30663,#30664),(#30665,#30666),(#30667,#30668),
(#30669,#30670),(#30671,#30672),(#30673,#30674),(#30675,#30676),(#30677,
#30678),(#30679,#30680),(#30681,#30682),(#30683,#30684),(#30685,#30686),
(#30687,#30688),(#30689,#30690),(#30691,#30692),(#30693,#30694),(#30695,
#30696),(#30697,#30698),(#30699,#30700),(#30701,#30702),(#30703,#30704),
(#30705,#30706),(#30707,#30708),(#30709,#30710),(#30711,#30712),(#30713,
#30714),(#30715,#30716),(#30717,#30718),(#30719,#30720)),.UNSPECIFIED.,
 .F.,.F.,.F.)
B_SPLINE_SURFACE_WITH_KNOTS((6,1,1,1,1,1,1,1,1,1,1,1,1,1,1,1,1,1,1,1,1,
1,1,1,1,1,1,1,1,1,1,1,1,1,1,1,1,1,1,1,1,1,1,1,1,1,1,1,1,1,1,1,1,1,1,1,1,
1,1,1,1,1,1,1,1,6),(2,2),(-1.,-0.984615384615383,-0.969230769230768,-0.953846153846152,
-0.938461538461537,-0.923076923076922,-0.907692307692306,-0.892307692307691,
-0.876923076923076,-0.86153846153846,-0.846153846153845,-0.83076923076923,
-0.815384615384614,-0.799999999999999,-0.784615384615384,-0.769230769230768,
-0.753846153846153,-0.738461538461538,-0.723076923076922,-0.707692307692307,
-0.692307692307692,-0.676923076923076,-0.661538461538461,-0.646153846153846,
-0.63076923076923,-0.615384615384615,-0.6,-0.584615384615384,-0.569230769230769,
-0.553846153846154,-0.538461538461538,-0.523076923076923,-0.507692307692308,
-0.492307692307692,-0.476923076923077,-0.461538461538462,-0.446153846153846,
-0.430769230769231,-0.415384615384615,-0.4,-0.384615384615385,-0.369230769230769,
-0.353846153846154,-0.338461538461538,-0.323076923076923,-0.307692307692308,
-0.292307692307692,-0.276923076923077,-0.261538461538462,-0.246153846153846,
-0.230769230769231,-0.215384615384615,-0.2,-0.184615384615385,-0.169230769230769,
-0.153846153846154,-0.138461538461538,-0.123076923076923,-0.107692307692308,
-0.0923076923076923,-0.0769230769230769,-0.0615384615384615,-0.0461538461538462,
-0.0307692307692308,-0.0153846153846154,0.),(-1.,1.),.UNSPECIFIED.)
GEOMETRIC_REPRESENTATION_ITEM()
RATIONAL_B_SPLINE_SURFACE(((1.,1.),(1.,1.),(1.,1.),(1.,1.),(1.,1.),(1.,
1.),(1.,1.),(1.,1.),(1.,1.),(1.,1.),(1.,1.),(1.,1.),(1.,1.),(1.,1.),(1.,
1.),(1.,1.),(1.,1.),(1.,1.),(1.,1.),(1.,1.),(1.,1.),(1.,1.),(1.,1.),(1.,
1.),(1.,1.),(1.,1.),(1.,1.),(1.,1.),(1.,1.),(1.,1.),(1.,1.),(1.,1.),(1.,
1.),(1.,1.),(1.,1.),(1.,1.),(1.,1.),(1.,1.),(1.,1.),(1.,1.),(1.,1.),(1.,
1.),(1.,1.),(1.,1.),(1.,1.),(1.,1.),(1.,1.),(1.,1.),(1.,1.),(1.,1.),(1.,
1.),(1.,1.),(1.,1.),(1.,1.),(1.,1.),(1.,1.),(1.,1.),(1.,1.),(1.,1.),(1.,
1.),(1.,1.),(1.,1.),(1.,1.),(1.,1.),(1.,1.),(1.,1.),(1.,1.),(1.,1.),(1.,
1.),(1.,1.)))
REPRESENTATION_ITEM('')
SURFACE()
);
#41=(
BOUNDED_SURFACE()
B_SPLINE_SURFACE(5,1,((#30797,#30798),(#30799,#30800),(#30801,#30802),(#30803,
#30804),(#30805,#30806),(#30807,#30808),(#30809,#30810),(#30811,#30812),
(#30813,#30814),(#30815,#30816),(#30817,#30818),(#30819,#30820),(#30821,
#30822),(#30823,#30824),(#30825,#30826),(#30827,#30828),(#30829,#30830),
(#30831,#30832),(#30833,#30834),(#30835,#30836),(#30837,#30838),(#30839,
#30840),(#30841,#30842),(#30843,#30844),(#30845,#30846),(#30847,#30848),
(#30849,#30850),(#30851,#30852),(#30853,#30854),(#30855,#30856),(#30857,
#30858),(#30859,#30860),(#30861,#30862),(#30863,#30864),(#30865,#30866),
(#30867,#30868),(#30869,#30870),(#30871,#30872),(#30873,#30874),(#30875,
#30876),(#30877,#30878),(#30879,#30880),(#30881,#30882),(#30883,#30884),
(#30885,#30886),(#30887,#30888),(#30889,#30890),(#30891,#30892),(#30893,
#30894),(#30895,#30896),(#30897,#30898),(#30899,#30900),(#30901,#30902),
(#30903,#30904),(#30905,#30906),(#30907,#30908),(#30909,#30910),(#30911,
#30912),(#30913,#30914),(#30915,#30916),(#30917,#30918),(#30919,#30920),
(#30921,#30922),(#30923,#30924),(#30925,#30926),(#30927,#30928),(#30929,
#30930),(#30931,#30932),(#30933,#30934),(#30935,#30936)),.UNSPECIFIED.,
 .F.,.F.,.F.)
B_SPLINE_SURFACE_WITH_KNOTS((6,1,1,1,1,1,1,1,1,1,1,1,1,1,1,1,1,1,1,1,1,
1,1,1,1,1,1,1,1,1,1,1,1,1,1,1,1,1,1,1,1,1,1,1,1,1,1,1,1,1,1,1,1,1,1,1,1,
1,1,1,1,1,1,1,1,6),(2,2),(-1.,-0.984615384615383,-0.969230769230768,-0.953846153846152,
-0.938461538461537,-0.923076923076922,-0.907692307692306,-0.892307692307691,
-0.876923076923076,-0.86153846153846,-0.846153846153845,-0.83076923076923,
-0.815384615384614,-0.799999999999999,-0.784615384615384,-0.769230769230768,
-0.753846153846153,-0.738461538461538,-0.723076923076922,-0.707692307692307,
-0.692307692307692,-0.676923076923076,-0.661538461538461,-0.646153846153846,
-0.63076923076923,-0.615384615384615,-0.6,-0.584615384615384,-0.569230769230769,
-0.553846153846154,-0.538461538461538,-0.523076923076923,-0.507692307692308,
-0.492307692307692,-0.476923076923077,-0.461538461538462,-0.446153846153846,
-0.430769230769231,-0.415384615384615,-0.4,-0.384615384615385,-0.369230769230769,
-0.353846153846154,-0.338461538461538,-0.323076923076923,-0.307692307692308,
-0.292307692307692,-0.276923076923077,-0.261538461538462,-0.246153846153846,
-0.230769230769231,-0.215384615384615,-0.2,-0.184615384615385,-0.169230769230769,
-0.153846153846154,-0.138461538461538,-0.123076923076923,-0.107692307692308,
-0.0923076923076923,-0.0769230769230769,-0.0615384615384615,-0.0461538461538462,
-0.0307692307692308,-0.0153846153846154,0.),(-1.,1.),.UNSPECIFIED.)
GEOMETRIC_REPRESENTATION_ITEM()
RATIONAL_B_SPLINE_SURFACE(((1.,1.),(1.,1.),(1.,1.),(1.,1.),(1.,1.),(1.,
1.),(1.,1.),(1.,1.),(1.,1.),(1.,1.),(1.,1.),(1.,1.),(1.,1.),(1.,1.),(1.,
1.),(1.,1.),(1.,1.),(1.,1.),(1.,1.),(1.,1.),(1.,1.),(1.,1.),(1.,1.),(1.,
1.),(1.,1.),(1.,1.),(1.,1.),(1.,1.),(1.,1.),(1.,1.),(1.,1.),(1.,1.),(1.,
1.),(1.,1.),(1.,1.),(1.,1.),(1.,1.),(1.,1.),(1.,1.),(1.,1.),(1.,1.),(1.,
1.),(1.,1.),(1.,1.),(1.,1.),(1.,1.),(1.,1.),(1.,1.),(1.,1.),(1.,1.),(1.,
1.),(1.,1.),(1.,1.),(1.,1.),(1.,1.),(1.,1.),(1.,1.),(1.,1.),(1.,1.),(1.,
1.),(1.,1.),(1.,1.),(1.,1.),(1.,1.),(1.,1.),(1.,1.),(1.,1.),(1.,1.),(1.,
1.),(1.,1.)))
REPRESENTATION_ITEM('')
SURFACE()
);
#42=(
BOUNDED_SURFACE()
B_SPLINE_SURFACE(5,1,((#31013,#31014),(#31015,#31016),(#31017,#31018),(#31019,
#31020),(#31021,#31022),(#31023,#31024),(#31025,#31026),(#31027,#31028),
(#31029,#31030),(#31031,#31032),(#31033,#31034),(#31035,#31036),(#31037,
#31038),(#31039,#31040),(#31041,#31042),(#31043,#31044),(#31045,#31046),
(#31047,#31048),(#31049,#31050),(#31051,#31052),(#31053,#31054),(#31055,
#31056),(#31057,#31058),(#31059,#31060),(#31061,#31062),(#31063,#31064),
(#31065,#31066),(#31067,#31068),(#31069,#31070),(#31071,#31072),(#31073,
#31074),(#31075,#31076),(#31077,#31078),(#31079,#31080),(#31081,#31082),
(#31083,#31084),(#31085,#31086),(#31087,#31088),(#31089,#31090),(#31091,
#31092),(#31093,#31094),(#31095,#31096),(#31097,#31098),(#31099,#31100),
(#31101,#31102),(#31103,#31104),(#31105,#31106),(#31107,#31108),(#31109,
#31110),(#31111,#31112),(#31113,#31114),(#31115,#31116),(#31117,#31118),
(#31119,#31120),(#31121,#31122),(#31123,#31124),(#31125,#31126),(#31127,
#31128),(#31129,#31130),(#31131,#31132),(#31133,#31134),(#31135,#31136),
(#31137,#31138),(#31139,#31140),(#31141,#31142),(#31143,#31144),(#31145,
#31146),(#31147,#31148),(#31149,#31150),(#31151,#31152)),.UNSPECIFIED.,
 .F.,.F.,.F.)
B_SPLINE_SURFACE_WITH_KNOTS((6,1,1,1,1,1,1,1,1,1,1,1,1,1,1,1,1,1,1,1,1,
1,1,1,1,1,1,1,1,1,1,1,1,1,1,1,1,1,1,1,1,1,1,1,1,1,1,1,1,1,1,1,1,1,1,1,1,
1,1,1,1,1,1,1,1,6),(2,2),(-1.,-0.984615384615383,-0.969230769230768,-0.953846153846152,
-0.938461538461537,-0.923076923076922,-0.907692307692306,-0.892307692307691,
-0.876923076923076,-0.86153846153846,-0.846153846153845,-0.83076923076923,
-0.815384615384614,-0.799999999999999,-0.784615384615384,-0.769230769230768,
-0.753846153846153,-0.738461538461538,-0.723076923076922,-0.707692307692307,
-0.692307692307692,-0.676923076923076,-0.661538461538461,-0.646153846153846,
-0.63076923076923,-0.615384615384615,-0.6,-0.584615384615384,-0.569230769230769,
-0.553846153846154,-0.538461538461538,-0.523076923076923,-0.507692307692308,
-0.492307692307692,-0.476923076923077,-0.461538461538462,-0.446153846153846,
-0.430769230769231,-0.415384615384615,-0.4,-0.384615384615385,-0.369230769230769,
-0.353846153846154,-0.338461538461538,-0.323076923076923,-0.307692307692308,
-0.292307692307692,-0.276923076923077,-0.261538461538462,-0.246153846153846,
-0.230769230769231,-0.215384615384615,-0.2,-0.184615384615385,-0.169230769230769,
-0.153846153846154,-0.138461538461538,-0.123076923076923,-0.107692307692308,
-0.0923076923076923,-0.0769230769230769,-0.0615384615384615,-0.0461538461538462,
-0.0307692307692308,-0.0153846153846154,0.),(-1.,1.),.UNSPECIFIED.)
GEOMETRIC_REPRESENTATION_ITEM()
RATIONAL_B_SPLINE_SURFACE(((1.,1.),(1.,1.),(1.,1.),(1.,1.),(1.,1.),(1.,
1.),(1.,1.),(1.,1.),(1.,1.),(1.,1.),(1.,1.),(1.,1.),(1.,1.),(1.,1.),(1.,
1.),(1.,1.),(1.,1.),(1.,1.),(1.,1.),(1.,1.),(1.,1.),(1.,1.),(1.,1.),(1.,
1.),(1.,1.),(1.,1.),(1.,1.),(1.,1.),(1.,1.),(1.,1.),(1.,1.),(1.,1.),(1.,
1.),(1.,1.),(1.,1.),(1.,1.),(1.,1.),(1.,1.),(1.,1.),(1.,1.),(1.,1.),(1.,
1.),(1.,1.),(1.,1.),(1.,1.),(1.,1.),(1.,1.),(1.,1.),(1.,1.),(1.,1.),(1.,
1.),(1.,1.),(1.,1.),(1.,1.),(1.,1.),(1.,1.),(1.,1.),(1.,1.),(1.,1.),(1.,
1.),(1.,1.),(1.,1.),(1.,1.),(1.,1.),(1.,1.),(1.,1.),(1.,1.),(1.,1.),(1.,
1.),(1.,1.)))
REPRESENTATION_ITEM('')
SURFACE()
);
#43=(
BOUNDED_SURFACE()
B_SPLINE_SURFACE(5,1,((#31229,#31230),(#31231,#31232),(#31233,#31234),(#31235,
#31236),(#31237,#31238),(#31239,#31240),(#31241,#31242),(#31243,#31244),
(#31245,#31246),(#31247,#31248),(#31249,#31250),(#31251,#31252),(#31253,
#31254),(#31255,#31256),(#31257,#31258),(#31259,#31260),(#31261,#31262),
(#31263,#31264),(#31265,#31266),(#31267,#31268),(#31269,#31270),(#31271,
#31272),(#31273,#31274),(#31275,#31276),(#31277,#31278),(#31279,#31280),
(#31281,#31282),(#31283,#31284),(#31285,#31286),(#31287,#31288),(#31289,
#31290),(#31291,#31292),(#31293,#31294),(#31295,#31296),(#31297,#31298),
(#31299,#31300),(#31301,#31302),(#31303,#31304),(#31305,#31306),(#31307,
#31308),(#31309,#31310),(#31311,#31312),(#31313,#31314),(#31315,#31316),
(#31317,#31318),(#31319,#31320),(#31321,#31322),(#31323,#31324),(#31325,
#31326),(#31327,#31328),(#31329,#31330),(#31331,#31332),(#31333,#31334),
(#31335,#31336),(#31337,#31338),(#31339,#31340),(#31341,#31342),(#31343,
#31344),(#31345,#31346),(#31347,#31348),(#31349,#31350),(#31351,#31352),
(#31353,#31354),(#31355,#31356),(#31357,#31358),(#31359,#31360),(#31361,
#31362),(#31363,#31364),(#31365,#31366),(#31367,#31368)),.UNSPECIFIED.,
 .F.,.F.,.F.)
B_SPLINE_SURFACE_WITH_KNOTS((6,1,1,1,1,1,1,1,1,1,1,1,1,1,1,1,1,1,1,1,1,
1,1,1,1,1,1,1,1,1,1,1,1,1,1,1,1,1,1,1,1,1,1,1,1,1,1,1,1,1,1,1,1,1,1,1,1,
1,1,1,1,1,1,1,1,6),(2,2),(-1.,-0.984615384615383,-0.969230769230768,-0.953846153846152,
-0.938461538461537,-0.923076923076922,-0.907692307692306,-0.892307692307691,
-0.876923076923076,-0.86153846153846,-0.846153846153845,-0.83076923076923,
-0.815384615384614,-0.799999999999999,-0.784615384615384,-0.769230769230768,
-0.753846153846153,-0.738461538461538,-0.723076923076922,-0.707692307692307,
-0.692307692307692,-0.676923076923076,-0.661538461538461,-0.646153846153846,
-0.63076923076923,-0.615384615384615,-0.6,-0.584615384615384,-0.569230769230769,
-0.553846153846154,-0.538461538461538,-0.523076923076923,-0.507692307692308,
-0.492307692307692,-0.476923076923077,-0.461538461538462,-0.446153846153846,
-0.430769230769231,-0.415384615384615,-0.4,-0.384615384615385,-0.369230769230769,
-0.353846153846154,-0.338461538461538,-0.323076923076923,-0.307692307692308,
-0.292307692307692,-0.276923076923077,-0.261538461538462,-0.246153846153846,
-0.230769230769231,-0.215384615384615,-0.2,-0.184615384615385,-0.169230769230769,
-0.153846153846154,-0.138461538461538,-0.123076923076923,-0.107692307692308,
-0.0923076923076923,-0.0769230769230769,-0.0615384615384615,-0.0461538461538462,
-0.0307692307692308,-0.0153846153846154,0.),(-1.,1.),.UNSPECIFIED.)
GEOMETRIC_REPRESENTATION_ITEM()
RATIONAL_B_SPLINE_SURFACE(((1.,1.),(1.,1.),(1.,1.),(1.,1.),(1.,1.),(1.,
1.),(1.,1.),(1.,1.),(1.,1.),(1.,1.),(1.,1.),(1.,1.),(1.,1.),(1.,1.),(1.,
1.),(1.,1.),(1.,1.),(1.,1.),(1.,1.),(1.,1.),(1.,1.),(1.,1.),(1.,1.),(1.,
1.),(1.,1.),(1.,1.),(1.,1.),(1.,1.),(1.,1.),(1.,1.),(1.,1.),(1.,1.),(1.,
1.),(1.,1.),(1.,1.),(1.,1.),(1.,1.),(1.,1.),(1.,1.),(1.,1.),(1.,1.),(1.,
1.),(1.,1.),(1.,1.),(1.,1.),(1.,1.),(1.,1.),(1.,1.),(1.,1.),(1.,1.),(1.,
1.),(1.,1.),(1.,1.),(1.,1.),(1.,1.),(1.,1.),(1.,1.),(1.,1.),(1.,1.),(1.,
1.),(1.,1.),(1.,1.),(1.,1.),(1.,1.),(1.,1.),(1.,1.),(1.,1.),(1.,1.),(1.,
1.),(1.,1.)))
REPRESENTATION_ITEM('')
SURFACE()
);
#44=(
BOUNDED_SURFACE()
B_SPLINE_SURFACE(5,1,((#31445,#31446),(#31447,#31448),(#31449,#31450),(#31451,
#31452),(#31453,#31454),(#31455,#31456),(#31457,#31458),(#31459,#31460),
(#31461,#31462),(#31463,#31464),(#31465,#31466),(#31467,#31468),(#31469,
#31470),(#31471,#31472),(#31473,#31474),(#31475,#31476),(#31477,#31478),
(#31479,#31480),(#31481,#31482),(#31483,#31484),(#31485,#31486),(#31487,
#31488),(#31489,#31490),(#31491,#31492),(#31493,#31494),(#31495,#31496),
(#31497,#31498),(#31499,#31500),(#31501,#31502),(#31503,#31504),(#31505,
#31506),(#31507,#31508),(#31509,#31510),(#31511,#31512),(#31513,#31514),
(#31515,#31516),(#31517,#31518),(#31519,#31520),(#31521,#31522),(#31523,
#31524),(#31525,#31526),(#31527,#31528),(#31529,#31530),(#31531,#31532),
(#31533,#31534),(#31535,#31536),(#31537,#31538),(#31539,#31540),(#31541,
#31542),(#31543,#31544),(#31545,#31546),(#31547,#31548),(#31549,#31550),
(#31551,#31552),(#31553,#31554),(#31555,#31556),(#31557,#31558),(#31559,
#31560),(#31561,#31562),(#31563,#31564),(#31565,#31566),(#31567,#31568),
(#31569,#31570),(#31571,#31572),(#31573,#31574),(#31575,#31576),(#31577,
#31578),(#31579,#31580),(#31581,#31582),(#31583,#31584)),.UNSPECIFIED.,
 .F.,.F.,.F.)
B_SPLINE_SURFACE_WITH_KNOTS((6,1,1,1,1,1,1,1,1,1,1,1,1,1,1,1,1,1,1,1,1,
1,1,1,1,1,1,1,1,1,1,1,1,1,1,1,1,1,1,1,1,1,1,1,1,1,1,1,1,1,1,1,1,1,1,1,1,
1,1,1,1,1,1,1,1,6),(2,2),(-1.,-0.984615384615383,-0.969230769230768,-0.953846153846152,
-0.938461538461537,-0.923076923076922,-0.907692307692306,-0.892307692307691,
-0.876923076923076,-0.86153846153846,-0.846153846153845,-0.83076923076923,
-0.815384615384614,-0.799999999999999,-0.784615384615384,-0.769230769230768,
-0.753846153846153,-0.738461538461538,-0.723076923076922,-0.707692307692307,
-0.692307692307692,-0.676923076923076,-0.661538461538461,-0.646153846153846,
-0.63076923076923,-0.615384615384615,-0.6,-0.584615384615384,-0.569230769230769,
-0.553846153846154,-0.538461538461538,-0.523076923076923,-0.507692307692308,
-0.492307692307692,-0.476923076923077,-0.461538461538462,-0.446153846153846,
-0.430769230769231,-0.415384615384615,-0.4,-0.384615384615385,-0.369230769230769,
-0.353846153846154,-0.338461538461538,-0.323076923076923,-0.307692307692308,
-0.292307692307692,-0.276923076923077,-0.261538461538462,-0.246153846153846,
-0.230769230769231,-0.215384615384615,-0.2,-0.184615384615385,-0.169230769230769,
-0.153846153846154,-0.138461538461538,-0.123076923076923,-0.107692307692308,
-0.0923076923076923,-0.0769230769230769,-0.0615384615384615,-0.0461538461538462,
-0.0307692307692308,-0.0153846153846154,0.),(-1.,1.),.UNSPECIFIED.)
GEOMETRIC_REPRESENTATION_ITEM()
RATIONAL_B_SPLINE_SURFACE(((1.,1.),(1.,1.),(1.,1.),(1.,1.),(1.,1.),(1.,
1.),(1.,1.),(1.,1.),(1.,1.),(1.,1.),(1.,1.),(1.,1.),(1.,1.),(1.,1.),(1.,
1.),(1.,1.),(1.,1.),(1.,1.),(1.,1.),(1.,1.),(1.,1.),(1.,1.),(1.,1.),(1.,
1.),(1.,1.),(1.,1.),(1.,1.),(1.,1.),(1.,1.),(1.,1.),(1.,1.),(1.,1.),(1.,
1.),(1.,1.),(1.,1.),(1.,1.),(1.,1.),(1.,1.),(1.,1.),(1.,1.),(1.,1.),(1.,
1.),(1.,1.),(1.,1.),(1.,1.),(1.,1.),(1.,1.),(1.,1.),(1.,1.),(1.,1.),(1.,
1.),(1.,1.),(1.,1.),(1.,1.),(1.,1.),(1.,1.),(1.,1.),(1.,1.),(1.,1.),(1.,
1.),(1.,1.),(1.,1.),(1.,1.),(1.,1.),(1.,1.),(1.,1.),(1.,1.),(1.,1.),(1.,
1.),(1.,1.)))
REPRESENTATION_ITEM('')
SURFACE()
);
#45=(
BOUNDED_SURFACE()
B_SPLINE_SURFACE(5,1,((#31661,#31662),(#31663,#31664),(#31665,#31666),(#31667,
#31668),(#31669,#31670),(#31671,#31672),(#31673,#31674),(#31675,#31676),
(#31677,#31678),(#31679,#31680),(#31681,#31682),(#31683,#31684),(#31685,
#31686),(#31687,#31688),(#31689,#31690),(#31691,#31692),(#31693,#31694),
(#31695,#31696),(#31697,#31698),(#31699,#31700),(#31701,#31702),(#31703,
#31704),(#31705,#31706),(#31707,#31708),(#31709,#31710),(#31711,#31712),
(#31713,#31714),(#31715,#31716),(#31717,#31718),(#31719,#31720),(#31721,
#31722),(#31723,#31724),(#31725,#31726),(#31727,#31728),(#31729,#31730),
(#31731,#31732),(#31733,#31734),(#31735,#31736),(#31737,#31738),(#31739,
#31740),(#31741,#31742),(#31743,#31744),(#31745,#31746),(#31747,#31748),
(#31749,#31750),(#31751,#31752),(#31753,#31754),(#31755,#31756),(#31757,
#31758),(#31759,#31760),(#31761,#31762),(#31763,#31764),(#31765,#31766),
(#31767,#31768),(#31769,#31770),(#31771,#31772),(#31773,#31774),(#31775,
#31776),(#31777,#31778),(#31779,#31780),(#31781,#31782),(#31783,#31784),
(#31785,#31786),(#31787,#31788),(#31789,#31790),(#31791,#31792),(#31793,
#31794),(#31795,#31796),(#31797,#31798),(#31799,#31800)),.UNSPECIFIED.,
 .F.,.F.,.F.)
B_SPLINE_SURFACE_WITH_KNOTS((6,1,1,1,1,1,1,1,1,1,1,1,1,1,1,1,1,1,1,1,1,
1,1,1,1,1,1,1,1,1,1,1,1,1,1,1,1,1,1,1,1,1,1,1,1,1,1,1,1,1,1,1,1,1,1,1,1,
1,1,1,1,1,1,1,1,6),(2,2),(-1.,-0.984615384615383,-0.969230769230768,-0.953846153846152,
-0.938461538461537,-0.923076923076922,-0.907692307692306,-0.892307692307691,
-0.876923076923076,-0.86153846153846,-0.846153846153845,-0.83076923076923,
-0.815384615384614,-0.799999999999999,-0.784615384615384,-0.769230769230768,
-0.753846153846153,-0.738461538461538,-0.723076923076922,-0.707692307692307,
-0.692307692307692,-0.676923076923076,-0.661538461538461,-0.646153846153846,
-0.63076923076923,-0.615384615384615,-0.6,-0.584615384615384,-0.569230769230769,
-0.553846153846154,-0.538461538461538,-0.523076923076923,-0.507692307692308,
-0.492307692307692,-0.476923076923077,-0.461538461538462,-0.446153846153846,
-0.430769230769231,-0.415384615384615,-0.4,-0.384615384615385,-0.369230769230769,
-0.353846153846154,-0.338461538461538,-0.323076923076923,-0.307692307692308,
-0.292307692307692,-0.276923076923077,-0.261538461538462,-0.246153846153846,
-0.230769230769231,-0.215384615384615,-0.2,-0.184615384615385,-0.169230769230769,
-0.153846153846154,-0.138461538461538,-0.123076923076923,-0.107692307692308,
-0.0923076923076923,-0.0769230769230769,-0.0615384615384615,-0.0461538461538462,
-0.0307692307692308,-0.0153846153846154,0.),(-1.,1.),.UNSPECIFIED.)
GEOMETRIC_REPRESENTATION_ITEM()
RATIONAL_B_SPLINE_SURFACE(((1.,1.),(1.,1.),(1.,1.),(1.,1.),(1.,1.),(1.,
1.),(1.,1.),(1.,1.),(1.,1.),(1.,1.),(1.,1.),(1.,1.),(1.,1.),(1.,1.),(1.,
1.),(1.,1.),(1.,1.),(1.,1.),(1.,1.),(1.,1.),(1.,1.),(1.,1.),(1.,1.),(1.,
1.),(1.,1.),(1.,1.),(1.,1.),(1.,1.),(1.,1.),(1.,1.),(1.,1.),(1.,1.),(1.,
1.),(1.,1.),(1.,1.),(1.,1.),(1.,1.),(1.,1.),(1.,1.),(1.,1.),(1.,1.),(1.,
1.),(1.,1.),(1.,1.),(1.,1.),(1.,1.),(1.,1.),(1.,1.),(1.,1.),(1.,1.),(1.,
1.),(1.,1.),(1.,1.),(1.,1.),(1.,1.),(1.,1.),(1.,1.),(1.,1.),(1.,1.),(1.,
1.),(1.,1.),(1.,1.),(1.,1.),(1.,1.),(1.,1.),(1.,1.),(1.,1.),(1.,1.),(1.,
1.),(1.,1.)))
REPRESENTATION_ITEM('')
SURFACE()
);
#46=(
BOUNDED_SURFACE()
B_SPLINE_SURFACE(5,1,((#31877,#31878),(#31879,#31880),(#31881,#31882),(#31883,
#31884),(#31885,#31886),(#31887,#31888),(#31889,#31890),(#31891,#31892),
(#31893,#31894),(#31895,#31896),(#31897,#31898),(#31899,#31900),(#31901,
#31902),(#31903,#31904),(#31905,#31906),(#31907,#31908),(#31909,#31910),
(#31911,#31912),(#31913,#31914),(#31915,#31916),(#31917,#31918),(#31919,
#31920),(#31921,#31922),(#31923,#31924),(#31925,#31926),(#31927,#31928),
(#31929,#31930),(#31931,#31932),(#31933,#31934),(#31935,#31936),(#31937,
#31938),(#31939,#31940),(#31941,#31942),(#31943,#31944),(#31945,#31946),
(#31947,#31948),(#31949,#31950),(#31951,#31952),(#31953,#31954),(#31955,
#31956),(#31957,#31958),(#31959,#31960),(#31961,#31962),(#31963,#31964),
(#31965,#31966),(#31967,#31968),(#31969,#31970),(#31971,#31972),(#31973,
#31974),(#31975,#31976),(#31977,#31978),(#31979,#31980),(#31981,#31982),
(#31983,#31984),(#31985,#31986),(#31987,#31988),(#31989,#31990),(#31991,
#31992),(#31993,#31994),(#31995,#31996),(#31997,#31998),(#31999,#32000),
(#32001,#32002),(#32003,#32004),(#32005,#32006),(#32007,#32008),(#32009,
#32010),(#32011,#32012),(#32013,#32014),(#32015,#32016)),.UNSPECIFIED.,
 .F.,.F.,.F.)
B_SPLINE_SURFACE_WITH_KNOTS((6,1,1,1,1,1,1,1,1,1,1,1,1,1,1,1,1,1,1,1,1,
1,1,1,1,1,1,1,1,1,1,1,1,1,1,1,1,1,1,1,1,1,1,1,1,1,1,1,1,1,1,1,1,1,1,1,1,
1,1,1,1,1,1,1,1,6),(2,2),(-1.,-0.984615384615383,-0.969230769230768,-0.953846153846152,
-0.938461538461537,-0.923076923076922,-0.907692307692306,-0.892307692307691,
-0.876923076923076,-0.86153846153846,-0.846153846153845,-0.83076923076923,
-0.815384615384614,-0.799999999999999,-0.784615384615384,-0.769230769230768,
-0.753846153846153,-0.738461538461538,-0.723076923076922,-0.707692307692307,
-0.692307692307692,-0.676923076923076,-0.661538461538461,-0.646153846153846,
-0.63076923076923,-0.615384615384615,-0.6,-0.584615384615384,-0.569230769230769,
-0.553846153846154,-0.538461538461538,-0.523076923076923,-0.507692307692308,
-0.492307692307692,-0.476923076923077,-0.461538461538462,-0.446153846153846,
-0.430769230769231,-0.415384615384615,-0.4,-0.384615384615385,-0.369230769230769,
-0.353846153846154,-0.338461538461538,-0.323076923076923,-0.307692307692308,
-0.292307692307692,-0.276923076923077,-0.261538461538462,-0.246153846153846,
-0.230769230769231,-0.215384615384615,-0.2,-0.184615384615385,-0.169230769230769,
-0.153846153846154,-0.138461538461538,-0.123076923076923,-0.107692307692308,
-0.0923076923076923,-0.0769230769230769,-0.0615384615384615,-0.0461538461538462,
-0.0307692307692308,-0.0153846153846154,0.),(-1.,1.),.UNSPECIFIED.)
GEOMETRIC_REPRESENTATION_ITEM()
RATIONAL_B_SPLINE_SURFACE(((1.,1.),(1.,1.),(1.,1.),(1.,1.),(1.,1.),(1.,
1.),(1.,1.),(1.,1.),(1.,1.),(1.,1.),(1.,1.),(1.,1.),(1.,1.),(1.,1.),(1.,
1.),(1.,1.),(1.,1.),(1.,1.),(1.,1.),(1.,1.),(1.,1.),(1.,1.),(1.,1.),(1.,
1.),(1.,1.),(1.,1.),(1.,1.),(1.,1.),(1.,1.),(1.,1.),(1.,1.),(1.,1.),(1.,
1.),(1.,1.),(1.,1.),(1.,1.),(1.,1.),(1.,1.),(1.,1.),(1.,1.),(1.,1.),(1.,
1.),(1.,1.),(1.,1.),(1.,1.),(1.,1.),(1.,1.),(1.,1.),(1.,1.),(1.,1.),(1.,
1.),(1.,1.),(1.,1.),(1.,1.),(1.,1.),(1.,1.),(1.,1.),(1.,1.),(1.,1.),(1.,
1.),(1.,1.),(1.,1.),(1.,1.),(1.,1.),(1.,1.),(1.,1.),(1.,1.),(1.,1.),(1.,
1.),(1.,1.)))
REPRESENTATION_ITEM('')
SURFACE()
);
#47=(
BOUNDED_SURFACE()
B_SPLINE_SURFACE(5,1,((#32093,#32094),(#32095,#32096),(#32097,#32098),(#32099,
#32100),(#32101,#32102),(#32103,#32104),(#32105,#32106),(#32107,#32108),
(#32109,#32110),(#32111,#32112),(#32113,#32114),(#32115,#32116),(#32117,
#32118),(#32119,#32120),(#32121,#32122),(#32123,#32124),(#32125,#32126),
(#32127,#32128),(#32129,#32130),(#32131,#32132),(#32133,#32134),(#32135,
#32136),(#32137,#32138),(#32139,#32140),(#32141,#32142),(#32143,#32144),
(#32145,#32146),(#32147,#32148),(#32149,#32150),(#32151,#32152),(#32153,
#32154),(#32155,#32156),(#32157,#32158),(#32159,#32160),(#32161,#32162),
(#32163,#32164),(#32165,#32166),(#32167,#32168),(#32169,#32170),(#32171,
#32172),(#32173,#32174),(#32175,#32176),(#32177,#32178),(#32179,#32180),
(#32181,#32182),(#32183,#32184),(#32185,#32186),(#32187,#32188),(#32189,
#32190),(#32191,#32192),(#32193,#32194),(#32195,#32196),(#32197,#32198),
(#32199,#32200),(#32201,#32202),(#32203,#32204),(#32205,#32206),(#32207,
#32208),(#32209,#32210),(#32211,#32212),(#32213,#32214),(#32215,#32216),
(#32217,#32218),(#32219,#32220),(#32221,#32222),(#32223,#32224),(#32225,
#32226),(#32227,#32228),(#32229,#32230),(#32231,#32232)),.UNSPECIFIED.,
 .F.,.F.,.F.)
B_SPLINE_SURFACE_WITH_KNOTS((6,1,1,1,1,1,1,1,1,1,1,1,1,1,1,1,1,1,1,1,1,
1,1,1,1,1,1,1,1,1,1,1,1,1,1,1,1,1,1,1,1,1,1,1,1,1,1,1,1,1,1,1,1,1,1,1,1,
1,1,1,1,1,1,1,1,6),(2,2),(-1.,-0.984615384615383,-0.969230769230768,-0.953846153846152,
-0.938461538461537,-0.923076923076922,-0.907692307692306,-0.892307692307691,
-0.876923076923076,-0.86153846153846,-0.846153846153845,-0.83076923076923,
-0.815384615384614,-0.799999999999999,-0.784615384615384,-0.769230769230768,
-0.753846153846153,-0.738461538461538,-0.723076923076922,-0.707692307692307,
-0.692307692307692,-0.676923076923076,-0.661538461538461,-0.646153846153846,
-0.63076923076923,-0.615384615384615,-0.6,-0.584615384615384,-0.569230769230769,
-0.553846153846154,-0.538461538461538,-0.523076923076923,-0.507692307692308,
-0.492307692307692,-0.476923076923077,-0.461538461538462,-0.446153846153846,
-0.430769230769231,-0.415384615384615,-0.4,-0.384615384615385,-0.369230769230769,
-0.353846153846154,-0.338461538461538,-0.323076923076923,-0.307692307692308,
-0.292307692307692,-0.276923076923077,-0.261538461538462,-0.246153846153846,
-0.230769230769231,-0.215384615384615,-0.2,-0.184615384615385,-0.169230769230769,
-0.153846153846154,-0.138461538461538,-0.123076923076923,-0.107692307692308,
-0.0923076923076923,-0.0769230769230769,-0.0615384615384615,-0.0461538461538462,
-0.0307692307692308,-0.0153846153846154,0.),(-1.,1.),.UNSPECIFIED.)
GEOMETRIC_REPRESENTATION_ITEM()
RATIONAL_B_SPLINE_SURFACE(((1.,1.),(1.,1.),(1.,1.),(1.,1.),(1.,1.),(1.,
1.),(1.,1.),(1.,1.),(1.,1.),(1.,1.),(1.,1.),(1.,1.),(1.,1.),(1.,1.),(1.,
1.),(1.,1.),(1.,1.),(1.,1.),(1.,1.),(1.,1.),(1.,1.),(1.,1.),(1.,1.),(1.,
1.),(1.,1.),(1.,1.),(1.,1.),(1.,1.),(1.,1.),(1.,1.),(1.,1.),(1.,1.),(1.,
1.),(1.,1.),(1.,1.),(1.,1.),(1.,1.),(1.,1.),(1.,1.),(1.,1.),(1.,1.),(1.,
1.),(1.,1.),(1.,1.),(1.,1.),(1.,1.),(1.,1.),(1.,1.),(1.,1.),(1.,1.),(1.,
1.),(1.,1.),(1.,1.),(1.,1.),(1.,1.),(1.,1.),(1.,1.),(1.,1.),(1.,1.),(1.,
1.),(1.,1.),(1.,1.),(1.,1.),(1.,1.),(1.,1.),(1.,1.),(1.,1.),(1.,1.),(1.,
1.),(1.,1.)))
REPRESENTATION_ITEM('')
SURFACE()
);
#48=(
BOUNDED_SURFACE()
B_SPLINE_SURFACE(5,1,((#32309,#32310),(#32311,#32312),(#32313,#32314),(#32315,
#32316),(#32317,#32318),(#32319,#32320),(#32321,#32322),(#32323,#32324),
(#32325,#32326),(#32327,#32328),(#32329,#32330),(#32331,#32332),(#32333,
#32334),(#32335,#32336),(#32337,#32338),(#32339,#32340),(#32341,#32342),
(#32343,#32344),(#32345,#32346),(#32347,#32348),(#32349,#32350),(#32351,
#32352),(#32353,#32354),(#32355,#32356),(#32357,#32358),(#32359,#32360),
(#32361,#32362),(#32363,#32364),(#32365,#32366),(#32367,#32368),(#32369,
#32370),(#32371,#32372),(#32373,#32374),(#32375,#32376),(#32377,#32378),
(#32379,#32380),(#32381,#32382),(#32383,#32384),(#32385,#32386),(#32387,
#32388),(#32389,#32390),(#32391,#32392),(#32393,#32394),(#32395,#32396),
(#32397,#32398),(#32399,#32400),(#32401,#32402),(#32403,#32404),(#32405,
#32406),(#32407,#32408),(#32409,#32410),(#32411,#32412),(#32413,#32414),
(#32415,#32416),(#32417,#32418),(#32419,#32420),(#32421,#32422),(#32423,
#32424),(#32425,#32426),(#32427,#32428),(#32429,#32430),(#32431,#32432),
(#32433,#32434),(#32435,#32436),(#32437,#32438),(#32439,#32440),(#32441,
#32442),(#32443,#32444),(#32445,#32446),(#32447,#32448)),.UNSPECIFIED.,
 .F.,.F.,.F.)
B_SPLINE_SURFACE_WITH_KNOTS((6,1,1,1,1,1,1,1,1,1,1,1,1,1,1,1,1,1,1,1,1,
1,1,1,1,1,1,1,1,1,1,1,1,1,1,1,1,1,1,1,1,1,1,1,1,1,1,1,1,1,1,1,1,1,1,1,1,
1,1,1,1,1,1,1,1,6),(2,2),(-1.,-0.984615384615383,-0.969230769230768,-0.953846153846152,
-0.938461538461537,-0.923076923076922,-0.907692307692306,-0.892307692307691,
-0.876923076923076,-0.86153846153846,-0.846153846153845,-0.83076923076923,
-0.815384615384614,-0.799999999999999,-0.784615384615384,-0.769230769230768,
-0.753846153846153,-0.738461538461538,-0.723076923076922,-0.707692307692307,
-0.692307692307692,-0.676923076923076,-0.661538461538461,-0.646153846153846,
-0.63076923076923,-0.615384615384615,-0.6,-0.584615384615384,-0.569230769230769,
-0.553846153846154,-0.538461538461538,-0.523076923076923,-0.507692307692308,
-0.492307692307692,-0.476923076923077,-0.461538461538462,-0.446153846153846,
-0.430769230769231,-0.415384615384615,-0.4,-0.384615384615385,-0.369230769230769,
-0.353846153846154,-0.338461538461538,-0.323076923076923,-0.307692307692308,
-0.292307692307692,-0.276923076923077,-0.261538461538462,-0.246153846153846,
-0.230769230769231,-0.215384615384615,-0.2,-0.184615384615385,-0.169230769230769,
-0.153846153846154,-0.138461538461538,-0.123076923076923,-0.107692307692308,
-0.0923076923076923,-0.0769230769230769,-0.0615384615384615,-0.0461538461538462,
-0.0307692307692308,-0.0153846153846154,0.),(-1.,1.),.UNSPECIFIED.)
GEOMETRIC_REPRESENTATION_ITEM()
RATIONAL_B_SPLINE_SURFACE(((1.,1.),(1.,1.),(1.,1.),(1.,1.),(1.,1.),(1.,
1.),(1.,1.),(1.,1.),(1.,1.),(1.,1.),(1.,1.),(1.,1.),(1.,1.),(1.,1.),(1.,
1.),(1.,1.),(1.,1.),(1.,1.),(1.,1.),(1.,1.),(1.,1.),(1.,1.),(1.,1.),(1.,
1.),(1.,1.),(1.,1.),(1.,1.),(1.,1.),(1.,1.),(1.,1.),(1.,1.),(1.,1.),(1.,
1.),(1.,1.),(1.,1.),(1.,1.),(1.,1.),(1.,1.),(1.,1.),(1.,1.),(1.,1.),(1.,
1.),(1.,1.),(1.,1.),(1.,1.),(1.,1.),(1.,1.),(1.,1.),(1.,1.),(1.,1.),(1.,
1.),(1.,1.),(1.,1.),(1.,1.),(1.,1.),(1.,1.),(1.,1.),(1.,1.),(1.,1.),(1.,
1.),(1.,1.),(1.,1.),(1.,1.),(1.,1.),(1.,1.),(1.,1.),(1.,1.),(1.,1.),(1.,
1.),(1.,1.)))
REPRESENTATION_ITEM('')
SURFACE()
);
#49=(
BOUNDED_SURFACE()
B_SPLINE_SURFACE(5,1,((#32525,#32526),(#32527,#32528),(#32529,#32530),(#32531,
#32532),(#32533,#32534),(#32535,#32536),(#32537,#32538),(#32539,#32540),
(#32541,#32542),(#32543,#32544),(#32545,#32546),(#32547,#32548),(#32549,
#32550),(#32551,#32552),(#32553,#32554),(#32555,#32556),(#32557,#32558),
(#32559,#32560),(#32561,#32562),(#32563,#32564),(#32565,#32566),(#32567,
#32568),(#32569,#32570),(#32571,#32572),(#32573,#32574),(#32575,#32576),
(#32577,#32578),(#32579,#32580),(#32581,#32582),(#32583,#32584),(#32585,
#32586),(#32587,#32588),(#32589,#32590),(#32591,#32592),(#32593,#32594),
(#32595,#32596),(#32597,#32598),(#32599,#32600),(#32601,#32602),(#32603,
#32604),(#32605,#32606),(#32607,#32608),(#32609,#32610),(#32611,#32612),
(#32613,#32614),(#32615,#32616),(#32617,#32618),(#32619,#32620),(#32621,
#32622),(#32623,#32624),(#32625,#32626),(#32627,#32628),(#32629,#32630),
(#32631,#32632),(#32633,#32634),(#32635,#32636),(#32637,#32638),(#32639,
#32640),(#32641,#32642),(#32643,#32644),(#32645,#32646),(#32647,#32648),
(#32649,#32650),(#32651,#32652),(#32653,#32654),(#32655,#32656),(#32657,
#32658),(#32659,#32660),(#32661,#32662),(#32663,#32664)),.UNSPECIFIED.,
 .F.,.F.,.F.)
B_SPLINE_SURFACE_WITH_KNOTS((6,1,1,1,1,1,1,1,1,1,1,1,1,1,1,1,1,1,1,1,1,
1,1,1,1,1,1,1,1,1,1,1,1,1,1,1,1,1,1,1,1,1,1,1,1,1,1,1,1,1,1,1,1,1,1,1,1,
1,1,1,1,1,1,1,1,6),(2,2),(-1.,-0.984615384615383,-0.969230769230768,-0.953846153846152,
-0.938461538461537,-0.923076923076922,-0.907692307692306,-0.892307692307691,
-0.876923076923076,-0.86153846153846,-0.846153846153845,-0.83076923076923,
-0.815384615384614,-0.799999999999999,-0.784615384615384,-0.769230769230768,
-0.753846153846153,-0.738461538461538,-0.723076923076922,-0.707692307692307,
-0.692307692307692,-0.676923076923076,-0.661538461538461,-0.646153846153846,
-0.63076923076923,-0.615384615384615,-0.6,-0.584615384615384,-0.569230769230769,
-0.553846153846154,-0.538461538461538,-0.523076923076923,-0.507692307692308,
-0.492307692307692,-0.476923076923077,-0.461538461538462,-0.446153846153846,
-0.430769230769231,-0.415384615384615,-0.4,-0.384615384615385,-0.369230769230769,
-0.353846153846154,-0.338461538461538,-0.323076923076923,-0.307692307692308,
-0.292307692307692,-0.276923076923077,-0.261538461538462,-0.246153846153846,
-0.230769230769231,-0.215384615384615,-0.2,-0.184615384615385,-0.169230769230769,
-0.153846153846154,-0.138461538461538,-0.123076923076923,-0.107692307692308,
-0.0923076923076923,-0.0769230769230769,-0.0615384615384615,-0.0461538461538462,
-0.0307692307692308,-0.0153846153846154,0.),(-1.,1.),.UNSPECIFIED.)
GEOMETRIC_REPRESENTATION_ITEM()
RATIONAL_B_SPLINE_SURFACE(((1.,1.),(1.,1.),(1.,1.),(1.,1.),(1.,1.),(1.,
1.),(1.,1.),(1.,1.),(1.,1.),(1.,1.),(1.,1.),(1.,1.),(1.,1.),(1.,1.),(1.,
1.),(1.,1.),(1.,1.),(1.,1.),(1.,1.),(1.,1.),(1.,1.),(1.,1.),(1.,1.),(1.,
1.),(1.,1.),(1.,1.),(1.,1.),(1.,1.),(1.,1.),(1.,1.),(1.,1.),(1.,1.),(1.,
1.),(1.,1.),(1.,1.),(1.,1.),(1.,1.),(1.,1.),(1.,1.),(1.,1.),(1.,1.),(1.,
1.),(1.,1.),(1.,1.),(1.,1.),(1.,1.),(1.,1.),(1.,1.),(1.,1.),(1.,1.),(1.,
1.),(1.,1.),(1.,1.),(1.,1.),(1.,1.),(1.,1.),(1.,1.),(1.,1.),(1.,1.),(1.,
1.),(1.,1.),(1.,1.),(1.,1.),(1.,1.),(1.,1.),(1.,1.),(1.,1.),(1.,1.),(1.,
1.),(1.,1.)))
REPRESENTATION_ITEM('')
SURFACE()
);
#50=(
BOUNDED_SURFACE()
B_SPLINE_SURFACE(5,1,((#32741,#32742),(#32743,#32744),(#32745,#32746),(#32747,
#32748),(#32749,#32750),(#32751,#32752),(#32753,#32754),(#32755,#32756),
(#32757,#32758),(#32759,#32760),(#32761,#32762),(#32763,#32764),(#32765,
#32766),(#32767,#32768),(#32769,#32770),(#32771,#32772),(#32773,#32774),
(#32775,#32776),(#32777,#32778),(#32779,#32780),(#32781,#32782),(#32783,
#32784),(#32785,#32786),(#32787,#32788),(#32789,#32790),(#32791,#32792),
(#32793,#32794),(#32795,#32796),(#32797,#32798),(#32799,#32800),(#32801,
#32802),(#32803,#32804),(#32805,#32806),(#32807,#32808),(#32809,#32810),
(#32811,#32812),(#32813,#32814),(#32815,#32816),(#32817,#32818),(#32819,
#32820),(#32821,#32822),(#32823,#32824),(#32825,#32826),(#32827,#32828),
(#32829,#32830),(#32831,#32832),(#32833,#32834),(#32835,#32836),(#32837,
#32838),(#32839,#32840),(#32841,#32842),(#32843,#32844),(#32845,#32846),
(#32847,#32848),(#32849,#32850),(#32851,#32852),(#32853,#32854),(#32855,
#32856),(#32857,#32858),(#32859,#32860),(#32861,#32862),(#32863,#32864),
(#32865,#32866),(#32867,#32868),(#32869,#32870),(#32871,#32872),(#32873,
#32874),(#32875,#32876),(#32877,#32878),(#32879,#32880)),.UNSPECIFIED.,
 .F.,.F.,.F.)
B_SPLINE_SURFACE_WITH_KNOTS((6,1,1,1,1,1,1,1,1,1,1,1,1,1,1,1,1,1,1,1,1,
1,1,1,1,1,1,1,1,1,1,1,1,1,1,1,1,1,1,1,1,1,1,1,1,1,1,1,1,1,1,1,1,1,1,1,1,
1,1,1,1,1,1,1,1,6),(2,2),(-1.,-0.984615384615383,-0.969230769230768,-0.953846153846152,
-0.938461538461537,-0.923076923076922,-0.907692307692306,-0.892307692307691,
-0.876923076923076,-0.86153846153846,-0.846153846153845,-0.83076923076923,
-0.815384615384614,-0.799999999999999,-0.784615384615384,-0.769230769230768,
-0.753846153846153,-0.738461538461538,-0.723076923076922,-0.707692307692307,
-0.692307692307692,-0.676923076923076,-0.661538461538461,-0.646153846153846,
-0.63076923076923,-0.615384615384615,-0.6,-0.584615384615384,-0.569230769230769,
-0.553846153846154,-0.538461538461538,-0.523076923076923,-0.507692307692308,
-0.492307692307692,-0.476923076923077,-0.461538461538462,-0.446153846153846,
-0.430769230769231,-0.415384615384615,-0.4,-0.384615384615385,-0.369230769230769,
-0.353846153846154,-0.338461538461538,-0.323076923076923,-0.307692307692308,
-0.292307692307692,-0.276923076923077,-0.261538461538462,-0.246153846153846,
-0.230769230769231,-0.215384615384615,-0.2,-0.184615384615385,-0.169230769230769,
-0.153846153846154,-0.138461538461538,-0.123076923076923,-0.107692307692308,
-0.0923076923076923,-0.0769230769230769,-0.0615384615384615,-0.0461538461538462,
-0.0307692307692308,-0.0153846153846154,0.),(-1.,1.),.UNSPECIFIED.)
GEOMETRIC_REPRESENTATION_ITEM()
RATIONAL_B_SPLINE_SURFACE(((1.,1.),(1.,1.),(1.,1.),(1.,1.),(1.,1.),(1.,
1.),(1.,1.),(1.,1.),(1.,1.),(1.,1.),(1.,1.),(1.,1.),(1.,1.),(1.,1.),(1.,
1.),(1.,1.),(1.,1.),(1.,1.),(1.,1.),(1.,1.),(1.,1.),(1.,1.),(1.,1.),(1.,
1.),(1.,1.),(1.,1.),(1.,1.),(1.,1.),(1.,1.),(1.,1.),(1.,1.),(1.,1.),(1.,
1.),(1.,1.),(1.,1.),(1.,1.),(1.,1.),(1.,1.),(1.,1.),(1.,1.),(1.,1.),(1.,
1.),(1.,1.),(1.,1.),(1.,1.),(1.,1.),(1.,1.),(1.,1.),(1.,1.),(1.,1.),(1.,
1.),(1.,1.),(1.,1.),(1.,1.),(1.,1.),(1.,1.),(1.,1.),(1.,1.),(1.,1.),(1.,
1.),(1.,1.),(1.,1.),(1.,1.),(1.,1.),(1.,1.),(1.,1.),(1.,1.),(1.,1.),(1.,
1.),(1.,1.)))
REPRESENTATION_ITEM('')
SURFACE()
);
#51=(
BOUNDED_CURVE()
B_SPLINE_CURVE(5,(#21389,#21390,#21391,#21392,#21393,#21394,#21395,#21396,
#21397,#21398,#21399,#21400,#21401,#21402,#21403,#21404,#21405,#21406,#21407,
#21408,#21409,#21410,#21411,#21412,#21413,#21414,#21415,#21416,#21417,#21418,
#21419,#21420,#21421,#21422,#21423,#21424,#21425,#21426,#21427,#21428,#21429,
#21430,#21431,#21432,#21433,#21434,#21435,#21436,#21437,#21438,#21439,#21440,
#21441,#21442,#21443,#21444,#21445,#21446,#21447,#21448,#21449,#21450,#21451,
#21452,#21453,#21454,#21455,#21456,#21457,#21458),.UNSPECIFIED.,.F.,.F.)
B_SPLINE_CURVE_WITH_KNOTS((6,1,1,1,1,1,1,1,1,1,1,1,1,1,1,1,1,1,1,1,1,1,
1,1,1,1,1,1,1,1,1,1,1,1,1,1,1,1,1,1,1,1,1,1,1,1,1,1,1,1,1,1,1,1,1,1,1,1,
1,1,1,1,1,1,1,6),(0.,0.0153846153846154,0.0307692307692308,0.0461538461538462,
0.0615384615384615,0.0769230769230769,0.0923076923076923,0.107692307692308,
0.123076923076923,0.138461538461538,0.153846153846154,0.169230769230769,
0.184615384615385,0.2,0.215384615384615,0.230769230769231,0.246153846153846,
0.261538461538462,0.276923076923077,0.292307692307692,0.307692307692308,
0.323076923076923,0.338461538461538,0.353846153846154,0.369230769230769,
0.384615384615385,0.4,0.415384615384615,0.430769230769231,0.446153846153846,
0.461538461538462,0.476923076923077,0.492307692307692,0.507692307692308,
0.523076923076923,0.538461538461538,0.553846153846154,0.569230769230769,
0.584615384615384,0.6,0.615384615384615,0.63076923076923,0.646153846153846,
0.661538461538461,0.676923076923076,0.692307692307692,0.707692307692307,
0.723076923076922,0.738461538461538,0.753846153846153,0.769230769230768,
0.784615384615384,0.799999999999999,0.815384615384614,0.83076923076923,
0.846153846153845,0.86153846153846,0.876923076923076,0.892307692307691,
0.907692307692306,0.923076923076922,0.938461538461537,0.953846153846152,
0.969230769230768,0.984615384615383,1.),.UNSPECIFIED.)
CURVE()
GEOMETRIC_REPRESENTATION_ITEM()
RATIONAL_B_SPLINE_CURVE((1.,1.,1.,1.,1.,1.,1.,1.,1.,1.,1.,1.,1.,1.,1.,1.,
1.,1.,1.,1.,1.,1.,1.,1.,1.,1.,1.,1.,1.,1.,1.,1.,1.,1.,1.,1.,1.,1.,1.,1.,
1.,1.,1.,1.,1.,1.,1.,1.,1.,1.,1.,1.,1.,1.,1.,1.,1.,1.,1.,1.,1.,1.,1.,1.,
1.,1.,1.,1.,1.,1.))
REPRESENTATION_ITEM('')
);
#52=(
BOUNDED_CURVE()
B_SPLINE_CURVE(5,(#21462,#21463,#21464,#21465,#21466,#21467,#21468,#21469,
#21470,#21471,#21472,#21473,#21474,#21475,#21476,#21477,#21478,#21479,#21480,
#21481,#21482,#21483,#21484,#21485,#21486,#21487,#21488,#21489,#21490,#21491,
#21492,#21493,#21494,#21495,#21496,#21497,#21498,#21499,#21500,#21501,#21502,
#21503,#21504,#21505,#21506,#21507,#21508,#21509,#21510,#21511,#21512,#21513,
#21514,#21515,#21516,#21517,#21518,#21519,#21520,#21521,#21522,#21523,#21524,
#21525,#21526,#21527,#21528,#21529,#21530,#21531),.UNSPECIFIED.,.F.,.F.)
B_SPLINE_CURVE_WITH_KNOTS((6,1,1,1,1,1,1,1,1,1,1,1,1,1,1,1,1,1,1,1,1,1,
1,1,1,1,1,1,1,1,1,1,1,1,1,1,1,1,1,1,1,1,1,1,1,1,1,1,1,1,1,1,1,1,1,1,1,1,
1,1,1,1,1,1,1,6),(0.,0.0153846153846154,0.0307692307692308,0.0461538461538462,
0.0615384615384615,0.0769230769230769,0.0923076923076923,0.107692307692308,
0.123076923076923,0.138461538461538,0.153846153846154,0.169230769230769,
0.184615384615385,0.2,0.215384615384615,0.230769230769231,0.246153846153846,
0.261538461538462,0.276923076923077,0.292307692307692,0.307692307692308,
0.323076923076923,0.338461538461538,0.353846153846154,0.369230769230769,
0.384615384615385,0.4,0.415384615384615,0.430769230769231,0.446153846153846,
0.461538461538462,0.476923076923077,0.492307692307692,0.507692307692308,
0.523076923076923,0.538461538461538,0.553846153846154,0.569230769230769,
0.584615384615384,0.6,0.615384615384615,0.63076923076923,0.646153846153846,
0.661538461538461,0.676923076923076,0.692307692307692,0.707692307692307,
0.723076923076922,0.738461538461538,0.753846153846153,0.769230769230768,
0.784615384615384,0.799999999999999,0.815384615384614,0.83076923076923,
0.846153846153845,0.86153846153846,0.876923076923076,0.892307692307691,
0.907692307692306,0.923076923076922,0.938461538461537,0.953846153846152,
0.969230769230768,0.984615384615383,1.),.UNSPECIFIED.)
CURVE()
GEOMETRIC_REPRESENTATION_ITEM()
RATIONAL_B_SPLINE_CURVE((1.,1.,1.,1.,1.,1.,1.,1.,1.,1.,1.,1.,1.,1.,1.,1.,
1.,1.,1.,1.,1.,1.,1.,1.,1.,1.,1.,1.,1.,1.,1.,1.,1.,1.,1.,1.,1.,1.,1.,1.,
1.,1.,1.,1.,1.,1.,1.,1.,1.,1.,1.,1.,1.,1.,1.,1.,1.,1.,1.,1.,1.,1.,1.,1.,
1.,1.,1.,1.,1.,1.))
REPRESENTATION_ITEM('')
);
#53=(
BOUNDED_CURVE()
B_SPLINE_CURVE(5,(#21535,#21536,#21537,#21538,#21539,#21540,#21541,#21542,
#21543,#21544,#21545,#21546,#21547,#21548,#21549,#21550,#21551,#21552,#21553,
#21554,#21555,#21556,#21557,#21558,#21559,#21560,#21561,#21562,#21563,#21564,
#21565,#21566,#21567,#21568,#21569,#21570,#21571,#21572,#21573,#21574,#21575,
#21576,#21577,#21578,#21579,#21580,#21581,#21582,#21583,#21584,#21585,#21586,
#21587,#21588,#21589,#21590,#21591,#21592,#21593,#21594,#21595,#21596,#21597,
#21598,#21599,#21600,#21601,#21602,#21603,#21604),.UNSPECIFIED.,.F.,.F.)
B_SPLINE_CURVE_WITH_KNOTS((6,1,1,1,1,1,1,1,1,1,1,1,1,1,1,1,1,1,1,1,1,1,
1,1,1,1,1,1,1,1,1,1,1,1,1,1,1,1,1,1,1,1,1,1,1,1,1,1,1,1,1,1,1,1,1,1,1,1,
1,1,1,1,1,1,1,6),(0.,0.0153846153846154,0.0307692307692308,0.0461538461538462,
0.0615384615384615,0.0769230769230769,0.0923076923076923,0.107692307692308,
0.123076923076923,0.138461538461538,0.153846153846154,0.169230769230769,
0.184615384615385,0.2,0.215384615384615,0.230769230769231,0.246153846153846,
0.261538461538462,0.276923076923077,0.292307692307692,0.307692307692308,
0.323076923076923,0.338461538461538,0.353846153846154,0.369230769230769,
0.384615384615385,0.4,0.415384615384615,0.430769230769231,0.446153846153846,
0.461538461538462,0.476923076923077,0.492307692307692,0.507692307692308,
0.523076923076923,0.538461538461538,0.553846153846154,0.569230769230769,
0.584615384615384,0.6,0.615384615384615,0.63076923076923,0.646153846153846,
0.661538461538461,0.676923076923076,0.692307692307692,0.707692307692307,
0.723076923076922,0.738461538461538,0.753846153846153,0.769230769230768,
0.784615384615384,0.799999999999999,0.815384615384614,0.83076923076923,
0.846153846153845,0.86153846153846,0.876923076923076,0.892307692307691,
0.907692307692306,0.923076923076922,0.938461538461537,0.953846153846152,
0.969230769230768,0.984615384615383,1.),.UNSPECIFIED.)
CURVE()
GEOMETRIC_REPRESENTATION_ITEM()
RATIONAL_B_SPLINE_CURVE((1.,1.,1.,1.,1.,1.,1.,1.,1.,1.,1.,1.,1.,1.,1.,1.,
1.,1.,1.,1.,1.,1.,1.,1.,1.,1.,1.,1.,1.,1.,1.,1.,1.,1.,1.,1.,1.,1.,1.,1.,
1.,1.,1.,1.,1.,1.,1.,1.,1.,1.,1.,1.,1.,1.,1.,1.,1.,1.,1.,1.,1.,1.,1.,1.,
1.,1.,1.,1.,1.,1.))
REPRESENTATION_ITEM('')
);
#54=(
BOUNDED_CURVE()
B_SPLINE_CURVE(5,(#21608,#21609,#21610,#21611,#21612,#21613,#21614,#21615,
#21616,#21617,#21618,#21619,#21620,#21621,#21622,#21623,#21624,#21625,#21626,
#21627,#21628,#21629,#21630,#21631,#21632,#21633,#21634,#21635,#21636,#21637,
#21638,#21639,#21640,#21641,#21642,#21643,#21644,#21645,#21646,#21647,#21648,
#21649,#21650,#21651,#21652,#21653,#21654,#21655,#21656,#21657,#21658,#21659,
#21660,#21661,#21662,#21663,#21664,#21665,#21666,#21667,#21668,#21669,#21670,
#21671,#21672,#21673,#21674,#21675,#21676,#21677),.UNSPECIFIED.,.F.,.F.)
B_SPLINE_CURVE_WITH_KNOTS((6,1,1,1,1,1,1,1,1,1,1,1,1,1,1,1,1,1,1,1,1,1,
1,1,1,1,1,1,1,1,1,1,1,1,1,1,1,1,1,1,1,1,1,1,1,1,1,1,1,1,1,1,1,1,1,1,1,1,
1,1,1,1,1,1,1,6),(0.,0.0153846153846154,0.0307692307692308,0.0461538461538462,
0.0615384615384615,0.0769230769230769,0.0923076923076923,0.107692307692308,
0.123076923076923,0.138461538461538,0.153846153846154,0.169230769230769,
0.184615384615385,0.2,0.215384615384615,0.230769230769231,0.246153846153846,
0.261538461538462,0.276923076923077,0.292307692307692,0.307692307692308,
0.323076923076923,0.338461538461538,0.353846153846154,0.369230769230769,
0.384615384615385,0.4,0.415384615384615,0.430769230769231,0.446153846153846,
0.461538461538462,0.476923076923077,0.492307692307692,0.507692307692308,
0.523076923076923,0.538461538461538,0.553846153846154,0.569230769230769,
0.584615384615384,0.6,0.615384615384615,0.63076923076923,0.646153846153846,
0.661538461538461,0.676923076923076,0.692307692307692,0.707692307692307,
0.723076923076922,0.738461538461538,0.753846153846153,0.769230769230768,
0.784615384615384,0.799999999999999,0.815384615384614,0.83076923076923,
0.846153846153845,0.86153846153846,0.876923076923076,0.892307692307691,
0.907692307692306,0.923076923076922,0.938461538461537,0.953846153846152,
0.969230769230768,0.984615384615383,1.),.UNSPECIFIED.)
CURVE()
GEOMETRIC_REPRESENTATION_ITEM()
RATIONAL_B_SPLINE_CURVE((1.,1.,1.,1.,1.,1.,1.,1.,1.,1.,1.,1.,1.,1.,1.,1.,
1.,1.,1.,1.,1.,1.,1.,1.,1.,1.,1.,1.,1.,1.,1.,1.,1.,1.,1.,1.,1.,1.,1.,1.,
1.,1.,1.,1.,1.,1.,1.,1.,1.,1.,1.,1.,1.,1.,1.,1.,1.,1.,1.,1.,1.,1.,1.,1.,
1.,1.,1.,1.,1.,1.))
REPRESENTATION_ITEM('')
);
#55=(
BOUNDED_CURVE()
B_SPLINE_CURVE(5,(#21681,#21682,#21683,#21684,#21685,#21686,#21687,#21688,
#21689,#21690,#21691,#21692,#21693,#21694,#21695,#21696,#21697,#21698,#21699,
#21700,#21701,#21702,#21703,#21704,#21705,#21706,#21707,#21708,#21709,#21710,
#21711,#21712,#21713,#21714,#21715,#21716,#21717,#21718,#21719,#21720,#21721,
#21722,#21723,#21724,#21725,#21726,#21727,#21728,#21729,#21730,#21731,#21732,
#21733,#21734,#21735,#21736,#21737,#21738,#21739,#21740,#21741,#21742,#21743,
#21744,#21745,#21746,#21747,#21748,#21749,#21750),.UNSPECIFIED.,.F.,.F.)
B_SPLINE_CURVE_WITH_KNOTS((6,1,1,1,1,1,1,1,1,1,1,1,1,1,1,1,1,1,1,1,1,1,
1,1,1,1,1,1,1,1,1,1,1,1,1,1,1,1,1,1,1,1,1,1,1,1,1,1,1,1,1,1,1,1,1,1,1,1,
1,1,1,1,1,1,1,6),(0.,0.0153846153846154,0.0307692307692308,0.0461538461538462,
0.0615384615384615,0.0769230769230769,0.0923076923076923,0.107692307692308,
0.123076923076923,0.138461538461538,0.153846153846154,0.169230769230769,
0.184615384615385,0.2,0.215384615384615,0.230769230769231,0.246153846153846,
0.261538461538462,0.276923076923077,0.292307692307692,0.307692307692308,
0.323076923076923,0.338461538461538,0.353846153846154,0.369230769230769,
0.384615384615385,0.4,0.415384615384615,0.430769230769231,0.446153846153846,
0.461538461538462,0.476923076923077,0.492307692307692,0.507692307692308,
0.523076923076923,0.538461538461538,0.553846153846154,0.569230769230769,
0.584615384615384,0.6,0.615384615384615,0.63076923076923,0.646153846153846,
0.661538461538461,0.676923076923076,0.692307692307692,0.707692307692307,
0.723076923076922,0.738461538461538,0.753846153846153,0.769230769230768,
0.784615384615384,0.799999999999999,0.815384615384614,0.83076923076923,
0.846153846153845,0.86153846153846,0.876923076923076,0.892307692307691,
0.907692307692306,0.923076923076922,0.938461538461537,0.953846153846152,
0.969230769230768,0.984615384615383,1.),.UNSPECIFIED.)
CURVE()
GEOMETRIC_REPRESENTATION_ITEM()
RATIONAL_B_SPLINE_CURVE((1.,1.,1.,1.,1.,1.,1.,1.,1.,1.,1.,1.,1.,1.,1.,1.,
1.,1.,1.,1.,1.,1.,1.,1.,1.,1.,1.,1.,1.,1.,1.,1.,1.,1.,1.,1.,1.,1.,1.,1.,
1.,1.,1.,1.,1.,1.,1.,1.,1.,1.,1.,1.,1.,1.,1.,1.,1.,1.,1.,1.,1.,1.,1.,1.,
1.,1.,1.,1.,1.,1.))
REPRESENTATION_ITEM('')
);
#56=(
BOUNDED_CURVE()
B_SPLINE_CURVE(5,(#21754,#21755,#21756,#21757,#21758,#21759,#21760,#21761,
#21762,#21763,#21764,#21765,#21766,#21767,#21768,#21769,#21770,#21771,#21772,
#21773,#21774,#21775,#21776,#21777,#21778,#21779,#21780,#21781,#21782,#21783,
#21784,#21785,#21786,#21787,#21788,#21789,#21790,#21791,#21792,#21793,#21794,
#21795,#21796,#21797,#21798,#21799,#21800,#21801,#21802,#21803,#21804,#21805,
#21806,#21807,#21808,#21809,#21810,#21811,#21812,#21813,#21814,#21815,#21816,
#21817,#21818,#21819,#21820,#21821,#21822,#21823),.UNSPECIFIED.,.F.,.F.)
B_SPLINE_CURVE_WITH_KNOTS((6,1,1,1,1,1,1,1,1,1,1,1,1,1,1,1,1,1,1,1,1,1,
1,1,1,1,1,1,1,1,1,1,1,1,1,1,1,1,1,1,1,1,1,1,1,1,1,1,1,1,1,1,1,1,1,1,1,1,
1,1,1,1,1,1,1,6),(0.,0.0153846153846154,0.0307692307692308,0.0461538461538462,
0.0615384615384615,0.0769230769230769,0.0923076923076923,0.107692307692308,
0.123076923076923,0.138461538461538,0.153846153846154,0.169230769230769,
0.184615384615385,0.2,0.215384615384615,0.230769230769231,0.246153846153846,
0.261538461538462,0.276923076923077,0.292307692307692,0.307692307692308,
0.323076923076923,0.338461538461538,0.353846153846154,0.369230769230769,
0.384615384615385,0.4,0.415384615384615,0.430769230769231,0.446153846153846,
0.461538461538462,0.476923076923077,0.492307692307692,0.507692307692308,
0.523076923076923,0.538461538461538,0.553846153846154,0.569230769230769,
0.584615384615384,0.6,0.615384615384615,0.63076923076923,0.646153846153846,
0.661538461538461,0.676923076923076,0.692307692307692,0.707692307692307,
0.723076923076922,0.738461538461538,0.753846153846153,0.769230769230768,
0.784615384615384,0.799999999999999,0.815384615384614,0.83076923076923,
0.846153846153845,0.86153846153846,0.876923076923076,0.892307692307691,
0.907692307692306,0.923076923076922,0.938461538461537,0.953846153846152,
0.969230769230768,0.984615384615383,1.),.UNSPECIFIED.)
CURVE()
GEOMETRIC_REPRESENTATION_ITEM()
RATIONAL_B_SPLINE_CURVE((1.,1.,1.,1.,1.,1.,1.,1.,1.,1.,1.,1.,1.,1.,1.,1.,
1.,1.,1.,1.,1.,1.,1.,1.,1.,1.,1.,1.,1.,1.,1.,1.,1.,1.,1.,1.,1.,1.,1.,1.,
1.,1.,1.,1.,1.,1.,1.,1.,1.,1.,1.,1.,1.,1.,1.,1.,1.,1.,1.,1.,1.,1.,1.,1.,
1.,1.,1.,1.,1.,1.))
REPRESENTATION_ITEM('')
);
#57=(
BOUNDED_CURVE()
B_SPLINE_CURVE(5,(#21827,#21828,#21829,#21830,#21831,#21832,#21833,#21834,
#21835,#21836,#21837,#21838,#21839,#21840,#21841,#21842,#21843,#21844,#21845,
#21846,#21847,#21848,#21849,#21850,#21851,#21852,#21853,#21854,#21855,#21856,
#21857,#21858,#21859,#21860,#21861,#21862,#21863,#21864,#21865,#21866,#21867,
#21868,#21869,#21870,#21871,#21872,#21873,#21874,#21875,#21876,#21877,#21878,
#21879,#21880,#21881,#21882,#21883,#21884,#21885,#21886,#21887,#21888,#21889,
#21890,#21891,#21892,#21893,#21894,#21895,#21896),.UNSPECIFIED.,.F.,.F.)
B_SPLINE_CURVE_WITH_KNOTS((6,1,1,1,1,1,1,1,1,1,1,1,1,1,1,1,1,1,1,1,1,1,
1,1,1,1,1,1,1,1,1,1,1,1,1,1,1,1,1,1,1,1,1,1,1,1,1,1,1,1,1,1,1,1,1,1,1,1,
1,1,1,1,1,1,1,6),(0.,0.0153846153846154,0.0307692307692308,0.0461538461538462,
0.0615384615384615,0.0769230769230769,0.0923076923076923,0.107692307692308,
0.123076923076923,0.138461538461538,0.153846153846154,0.169230769230769,
0.184615384615385,0.2,0.215384615384615,0.230769230769231,0.246153846153846,
0.261538461538462,0.276923076923077,0.292307692307692,0.307692307692308,
0.323076923076923,0.338461538461538,0.353846153846154,0.369230769230769,
0.384615384615385,0.4,0.415384615384615,0.430769230769231,0.446153846153846,
0.461538461538462,0.476923076923077,0.492307692307692,0.507692307692308,
0.523076923076923,0.538461538461538,0.553846153846154,0.569230769230769,
0.584615384615384,0.6,0.615384615384615,0.63076923076923,0.646153846153846,
0.661538461538461,0.676923076923076,0.692307692307692,0.707692307692307,
0.723076923076922,0.738461538461538,0.753846153846153,0.769230769230768,
0.784615384615384,0.799999999999999,0.815384615384614,0.83076923076923,
0.846153846153845,0.86153846153846,0.876923076923076,0.892307692307691,
0.907692307692306,0.923076923076922,0.938461538461537,0.953846153846152,
0.969230769230768,0.984615384615383,1.),.UNSPECIFIED.)
CURVE()
GEOMETRIC_REPRESENTATION_ITEM()
RATIONAL_B_SPLINE_CURVE((1.,1.,1.,1.,1.,1.,1.,1.,1.,1.,1.,1.,1.,1.,1.,1.,
1.,1.,1.,1.,1.,1.,1.,1.,1.,1.,1.,1.,1.,1.,1.,1.,1.,1.,1.,1.,1.,1.,1.,1.,
1.,1.,1.,1.,1.,1.,1.,1.,1.,1.,1.,1.,1.,1.,1.,1.,1.,1.,1.,1.,1.,1.,1.,1.,
1.,1.,1.,1.,1.,1.))
REPRESENTATION_ITEM('')
);
#58=(
BOUNDED_CURVE()
B_SPLINE_CURVE(5,(#21900,#21901,#21902,#21903,#21904,#21905,#21906,#21907,
#21908,#21909,#21910,#21911,#21912,#21913,#21914,#21915,#21916,#21917,#21918,
#21919,#21920,#21921,#21922,#21923,#21924,#21925,#21926,#21927,#21928,#21929,
#21930,#21931,#21932,#21933,#21934,#21935,#21936,#21937,#21938,#21939,#21940,
#21941,#21942,#21943,#21944,#21945,#21946,#21947,#21948,#21949,#21950,#21951,
#21952,#21953,#21954,#21955,#21956,#21957,#21958,#21959,#21960,#21961,#21962,
#21963,#21964,#21965,#21966,#21967,#21968,#21969),.UNSPECIFIED.,.F.,.F.)
B_SPLINE_CURVE_WITH_KNOTS((6,1,1,1,1,1,1,1,1,1,1,1,1,1,1,1,1,1,1,1,1,1,
1,1,1,1,1,1,1,1,1,1,1,1,1,1,1,1,1,1,1,1,1,1,1,1,1,1,1,1,1,1,1,1,1,1,1,1,
1,1,1,1,1,1,1,6),(0.,0.0153846153846154,0.0307692307692308,0.0461538461538462,
0.0615384615384615,0.0769230769230769,0.0923076923076923,0.107692307692308,
0.123076923076923,0.138461538461538,0.153846153846154,0.169230769230769,
0.184615384615385,0.2,0.215384615384615,0.230769230769231,0.246153846153846,
0.261538461538462,0.276923076923077,0.292307692307692,0.307692307692308,
0.323076923076923,0.338461538461538,0.353846153846154,0.369230769230769,
0.384615384615385,0.4,0.415384615384615,0.430769230769231,0.446153846153846,
0.461538461538462,0.476923076923077,0.492307692307692,0.507692307692308,
0.523076923076923,0.538461538461538,0.553846153846154,0.569230769230769,
0.584615384615384,0.6,0.615384615384615,0.63076923076923,0.646153846153846,
0.661538461538461,0.676923076923076,0.692307692307692,0.707692307692307,
0.723076923076922,0.738461538461538,0.753846153846153,0.769230769230768,
0.784615384615384,0.799999999999999,0.815384615384614,0.83076923076923,
0.846153846153845,0.86153846153846,0.876923076923076,0.892307692307691,
0.907692307692306,0.923076923076922,0.938461538461537,0.953846153846152,
0.969230769230768,0.984615384615383,1.),.UNSPECIFIED.)
CURVE()
GEOMETRIC_REPRESENTATION_ITEM()
RATIONAL_B_SPLINE_CURVE((1.,1.,1.,1.,1.,1.,1.,1.,1.,1.,1.,1.,1.,1.,1.,1.,
1.,1.,1.,1.,1.,1.,1.,1.,1.,1.,1.,1.,1.,1.,1.,1.,1.,1.,1.,1.,1.,1.,1.,1.,
1.,1.,1.,1.,1.,1.,1.,1.,1.,1.,1.,1.,1.,1.,1.,1.,1.,1.,1.,1.,1.,1.,1.,1.,
1.,1.,1.,1.,1.,1.))
REPRESENTATION_ITEM('')
);
#59=(
BOUNDED_CURVE()
B_SPLINE_CURVE(5,(#21973,#21974,#21975,#21976,#21977,#21978,#21979,#21980,
#21981,#21982,#21983,#21984,#21985,#21986,#21987,#21988,#21989,#21990,#21991,
#21992,#21993,#21994,#21995,#21996,#21997,#21998,#21999,#22000,#22001,#22002,
#22003,#22004,#22005,#22006,#22007,#22008,#22009,#22010,#22011,#22012,#22013,
#22014,#22015,#22016,#22017,#22018,#22019,#22020,#22021,#22022,#22023,#22024,
#22025,#22026,#22027,#22028,#22029,#22030,#22031,#22032,#22033,#22034,#22035,
#22036,#22037,#22038,#22039,#22040,#22041,#22042),.UNSPECIFIED.,.F.,.F.)
B_SPLINE_CURVE_WITH_KNOTS((6,1,1,1,1,1,1,1,1,1,1,1,1,1,1,1,1,1,1,1,1,1,
1,1,1,1,1,1,1,1,1,1,1,1,1,1,1,1,1,1,1,1,1,1,1,1,1,1,1,1,1,1,1,1,1,1,1,1,
1,1,1,1,1,1,1,6),(0.,0.0153846153846154,0.0307692307692308,0.0461538461538462,
0.0615384615384615,0.0769230769230769,0.0923076923076923,0.107692307692308,
0.123076923076923,0.138461538461538,0.153846153846154,0.169230769230769,
0.184615384615385,0.2,0.215384615384615,0.230769230769231,0.246153846153846,
0.261538461538462,0.276923076923077,0.292307692307692,0.307692307692308,
0.323076923076923,0.338461538461538,0.353846153846154,0.369230769230769,
0.384615384615385,0.4,0.415384615384615,0.430769230769231,0.446153846153846,
0.461538461538462,0.476923076923077,0.492307692307692,0.507692307692308,
0.523076923076923,0.538461538461538,0.553846153846154,0.569230769230769,
0.584615384615384,0.6,0.615384615384615,0.63076923076923,0.646153846153846,
0.661538461538461,0.676923076923076,0.692307692307692,0.707692307692307,
0.723076923076922,0.738461538461538,0.753846153846153,0.769230769230768,
0.784615384615384,0.799999999999999,0.815384615384614,0.83076923076923,
0.846153846153845,0.86153846153846,0.876923076923076,0.892307692307691,
0.907692307692306,0.923076923076922,0.938461538461537,0.953846153846152,
0.969230769230768,0.984615384615383,1.),.UNSPECIFIED.)
CURVE()
GEOMETRIC_REPRESENTATION_ITEM()
RATIONAL_B_SPLINE_CURVE((1.,1.,1.,1.,1.,1.,1.,1.,1.,1.,1.,1.,1.,1.,1.,1.,
1.,1.,1.,1.,1.,1.,1.,1.,1.,1.,1.,1.,1.,1.,1.,1.,1.,1.,1.,1.,1.,1.,1.,1.,
1.,1.,1.,1.,1.,1.,1.,1.,1.,1.,1.,1.,1.,1.,1.,1.,1.,1.,1.,1.,1.,1.,1.,1.,
1.,1.,1.,1.,1.,1.))
REPRESENTATION_ITEM('')
);
#60=(
BOUNDED_CURVE()
B_SPLINE_CURVE(5,(#22046,#22047,#22048,#22049,#22050,#22051,#22052,#22053,
#22054,#22055,#22056,#22057,#22058,#22059,#22060,#22061,#22062,#22063,#22064,
#22065,#22066,#22067,#22068,#22069,#22070,#22071,#22072,#22073,#22074,#22075,
#22076,#22077,#22078,#22079,#22080,#22081,#22082,#22083,#22084,#22085,#22086,
#22087,#22088,#22089,#22090,#22091,#22092,#22093,#22094,#22095,#22096,#22097,
#22098,#22099,#22100,#22101,#22102,#22103,#22104,#22105,#22106,#22107,#22108,
#22109,#22110,#22111,#22112,#22113,#22114,#22115),.UNSPECIFIED.,.F.,.F.)
B_SPLINE_CURVE_WITH_KNOTS((6,1,1,1,1,1,1,1,1,1,1,1,1,1,1,1,1,1,1,1,1,1,
1,1,1,1,1,1,1,1,1,1,1,1,1,1,1,1,1,1,1,1,1,1,1,1,1,1,1,1,1,1,1,1,1,1,1,1,
1,1,1,1,1,1,1,6),(0.,0.0153846153846154,0.0307692307692308,0.0461538461538462,
0.0615384615384615,0.0769230769230769,0.0923076923076923,0.107692307692308,
0.123076923076923,0.138461538461538,0.153846153846154,0.169230769230769,
0.184615384615385,0.2,0.215384615384615,0.230769230769231,0.246153846153846,
0.261538461538462,0.276923076923077,0.292307692307692,0.307692307692308,
0.323076923076923,0.338461538461538,0.353846153846154,0.369230769230769,
0.384615384615385,0.4,0.415384615384615,0.430769230769231,0.446153846153846,
0.461538461538462,0.476923076923077,0.492307692307692,0.507692307692308,
0.523076923076923,0.538461538461538,0.553846153846154,0.569230769230769,
0.584615384615384,0.6,0.615384615384615,0.63076923076923,0.646153846153846,
0.661538461538461,0.676923076923076,0.692307692307692,0.707692307692307,
0.723076923076922,0.738461538461538,0.753846153846153,0.769230769230768,
0.784615384615384,0.799999999999999,0.815384615384614,0.83076923076923,
0.846153846153845,0.86153846153846,0.876923076923076,0.892307692307691,
0.907692307692306,0.923076923076922,0.938461538461537,0.953846153846152,
0.969230769230768,0.984615384615383,1.),.UNSPECIFIED.)
CURVE()
GEOMETRIC_REPRESENTATION_ITEM()
RATIONAL_B_SPLINE_CURVE((1.,1.,1.,1.,1.,1.,1.,1.,1.,1.,1.,1.,1.,1.,1.,1.,
1.,1.,1.,1.,1.,1.,1.,1.,1.,1.,1.,1.,1.,1.,1.,1.,1.,1.,1.,1.,1.,1.,1.,1.,
1.,1.,1.,1.,1.,1.,1.,1.,1.,1.,1.,1.,1.,1.,1.,1.,1.,1.,1.,1.,1.,1.,1.,1.,
1.,1.,1.,1.,1.,1.))
REPRESENTATION_ITEM('')
);
#61=(
BOUNDED_CURVE()
B_SPLINE_CURVE(5,(#22119,#22120,#22121,#22122,#22123,#22124,#22125,#22126,
#22127,#22128,#22129,#22130,#22131,#22132,#22133,#22134,#22135,#22136,#22137,
#22138,#22139,#22140,#22141,#22142,#22143,#22144,#22145,#22146,#22147,#22148,
#22149,#22150,#22151,#22152,#22153,#22154,#22155,#22156,#22157,#22158,#22159,
#22160,#22161,#22162,#22163,#22164,#22165,#22166,#22167,#22168,#22169,#22170,
#22171,#22172,#22173,#22174,#22175,#22176,#22177,#22178,#22179,#22180,#22181,
#22182,#22183,#22184,#22185,#22186,#22187,#22188),.UNSPECIFIED.,.F.,.F.)
B_SPLINE_CURVE_WITH_KNOTS((6,1,1,1,1,1,1,1,1,1,1,1,1,1,1,1,1,1,1,1,1,1,
1,1,1,1,1,1,1,1,1,1,1,1,1,1,1,1,1,1,1,1,1,1,1,1,1,1,1,1,1,1,1,1,1,1,1,1,
1,1,1,1,1,1,1,6),(0.,0.0153846153846154,0.0307692307692308,0.0461538461538462,
0.0615384615384615,0.0769230769230769,0.0923076923076923,0.107692307692308,
0.123076923076923,0.138461538461538,0.153846153846154,0.169230769230769,
0.184615384615385,0.2,0.215384615384615,0.230769230769231,0.246153846153846,
0.261538461538462,0.276923076923077,0.292307692307692,0.307692307692308,
0.323076923076923,0.338461538461538,0.353846153846154,0.369230769230769,
0.384615384615385,0.4,0.415384615384615,0.430769230769231,0.446153846153846,
0.461538461538462,0.476923076923077,0.492307692307692,0.507692307692308,
0.523076923076923,0.538461538461538,0.553846153846154,0.569230769230769,
0.584615384615384,0.6,0.615384615384615,0.63076923076923,0.646153846153846,
0.661538461538461,0.676923076923076,0.692307692307692,0.707692307692307,
0.723076923076922,0.738461538461538,0.753846153846153,0.769230769230768,
0.784615384615384,0.799999999999999,0.815384615384614,0.83076923076923,
0.846153846153845,0.86153846153846,0.876923076923076,0.892307692307691,
0.907692307692306,0.923076923076922,0.938461538461537,0.953846153846152,
0.969230769230768,0.984615384615383,1.),.UNSPECIFIED.)
CURVE()
GEOMETRIC_REPRESENTATION_ITEM()
RATIONAL_B_SPLINE_CURVE((1.,1.,1.,1.,1.,1.,1.,1.,1.,1.,1.,1.,1.,1.,1.,1.,
1.,1.,1.,1.,1.,1.,1.,1.,1.,1.,1.,1.,1.,1.,1.,1.,1.,1.,1.,1.,1.,1.,1.,1.,
1.,1.,1.,1.,1.,1.,1.,1.,1.,1.,1.,1.,1.,1.,1.,1.,1.,1.,1.,1.,1.,1.,1.,1.,
1.,1.,1.,1.,1.,1.))
REPRESENTATION_ITEM('')
);
#62=(
BOUNDED_CURVE()
B_SPLINE_CURVE(5,(#22192,#22193,#22194,#22195,#22196,#22197,#22198,#22199,
#22200,#22201,#22202,#22203,#22204,#22205,#22206,#22207,#22208,#22209,#22210,
#22211,#22212,#22213,#22214,#22215,#22216,#22217,#22218,#22219,#22220,#22221,
#22222,#22223,#22224,#22225,#22226,#22227,#22228,#22229,#22230,#22231,#22232,
#22233,#22234,#22235,#22236,#22237,#22238,#22239,#22240,#22241,#22242,#22243,
#22244,#22245,#22246,#22247,#22248,#22249,#22250,#22251,#22252,#22253,#22254,
#22255,#22256,#22257,#22258,#22259,#22260,#22261),.UNSPECIFIED.,.F.,.F.)
B_SPLINE_CURVE_WITH_KNOTS((6,1,1,1,1,1,1,1,1,1,1,1,1,1,1,1,1,1,1,1,1,1,
1,1,1,1,1,1,1,1,1,1,1,1,1,1,1,1,1,1,1,1,1,1,1,1,1,1,1,1,1,1,1,1,1,1,1,1,
1,1,1,1,1,1,1,6),(0.,0.0153846153846154,0.0307692307692308,0.0461538461538462,
0.0615384615384615,0.0769230769230769,0.0923076923076923,0.107692307692308,
0.123076923076923,0.138461538461538,0.153846153846154,0.169230769230769,
0.184615384615385,0.2,0.215384615384615,0.230769230769231,0.246153846153846,
0.261538461538462,0.276923076923077,0.292307692307692,0.307692307692308,
0.323076923076923,0.338461538461538,0.353846153846154,0.369230769230769,
0.384615384615385,0.4,0.415384615384615,0.430769230769231,0.446153846153846,
0.461538461538462,0.476923076923077,0.492307692307692,0.507692307692308,
0.523076923076923,0.538461538461538,0.553846153846154,0.569230769230769,
0.584615384615384,0.6,0.615384615384615,0.63076923076923,0.646153846153846,
0.661538461538461,0.676923076923076,0.692307692307692,0.707692307692307,
0.723076923076922,0.738461538461538,0.753846153846153,0.769230769230768,
0.784615384615384,0.799999999999999,0.815384615384614,0.83076923076923,
0.846153846153845,0.86153846153846,0.876923076923076,0.892307692307691,
0.907692307692306,0.923076923076922,0.938461538461537,0.953846153846152,
0.969230769230768,0.984615384615383,1.),.UNSPECIFIED.)
CURVE()
GEOMETRIC_REPRESENTATION_ITEM()
RATIONAL_B_SPLINE_CURVE((1.,1.,1.,1.,1.,1.,1.,1.,1.,1.,1.,1.,1.,1.,1.,1.,
1.,1.,1.,1.,1.,1.,1.,1.,1.,1.,1.,1.,1.,1.,1.,1.,1.,1.,1.,1.,1.,1.,1.,1.,
1.,1.,1.,1.,1.,1.,1.,1.,1.,1.,1.,1.,1.,1.,1.,1.,1.,1.,1.,1.,1.,1.,1.,1.,
1.,1.,1.,1.,1.,1.))
REPRESENTATION_ITEM('')
);
#63=(
BOUNDED_CURVE()
B_SPLINE_CURVE(5,(#22265,#22266,#22267,#22268,#22269,#22270,#22271,#22272,
#22273,#22274,#22275,#22276,#22277,#22278,#22279,#22280,#22281,#22282,#22283,
#22284,#22285,#22286,#22287,#22288,#22289,#22290,#22291,#22292,#22293,#22294,
#22295,#22296,#22297,#22298,#22299,#22300,#22301,#22302,#22303,#22304,#22305,
#22306,#22307,#22308,#22309,#22310,#22311,#22312,#22313,#22314,#22315,#22316,
#22317,#22318,#22319,#22320,#22321,#22322,#22323,#22324,#22325,#22326,#22327,
#22328,#22329,#22330,#22331,#22332,#22333,#22334),.UNSPECIFIED.,.F.,.F.)
B_SPLINE_CURVE_WITH_KNOTS((6,1,1,1,1,1,1,1,1,1,1,1,1,1,1,1,1,1,1,1,1,1,
1,1,1,1,1,1,1,1,1,1,1,1,1,1,1,1,1,1,1,1,1,1,1,1,1,1,1,1,1,1,1,1,1,1,1,1,
1,1,1,1,1,1,1,6),(0.,0.0153846153846154,0.0307692307692308,0.0461538461538462,
0.0615384615384615,0.0769230769230769,0.0923076923076923,0.107692307692308,
0.123076923076923,0.138461538461538,0.153846153846154,0.169230769230769,
0.184615384615385,0.2,0.215384615384615,0.230769230769231,0.246153846153846,
0.261538461538462,0.276923076923077,0.292307692307692,0.307692307692308,
0.323076923076923,0.338461538461538,0.353846153846154,0.369230769230769,
0.384615384615385,0.4,0.415384615384615,0.430769230769231,0.446153846153846,
0.461538461538462,0.476923076923077,0.492307692307692,0.507692307692308,
0.523076923076923,0.538461538461538,0.553846153846154,0.569230769230769,
0.584615384615384,0.6,0.615384615384615,0.63076923076923,0.646153846153846,
0.661538461538461,0.676923076923076,0.692307692307692,0.707692307692307,
0.723076923076922,0.738461538461538,0.753846153846153,0.769230769230768,
0.784615384615384,0.799999999999999,0.815384615384614,0.83076923076923,
0.846153846153845,0.86153846153846,0.876923076923076,0.892307692307691,
0.907692307692306,0.923076923076922,0.938461538461537,0.953846153846152,
0.969230769230768,0.984615384615383,1.),.UNSPECIFIED.)
CURVE()
GEOMETRIC_REPRESENTATION_ITEM()
RATIONAL_B_SPLINE_CURVE((1.,1.,1.,1.,1.,1.,1.,1.,1.,1.,1.,1.,1.,1.,1.,1.,
1.,1.,1.,1.,1.,1.,1.,1.,1.,1.,1.,1.,1.,1.,1.,1.,1.,1.,1.,1.,1.,1.,1.,1.,
1.,1.,1.,1.,1.,1.,1.,1.,1.,1.,1.,1.,1.,1.,1.,1.,1.,1.,1.,1.,1.,1.,1.,1.,
1.,1.,1.,1.,1.,1.))
REPRESENTATION_ITEM('')
);
#64=(
BOUNDED_CURVE()
B_SPLINE_CURVE(5,(#22338,#22339,#22340,#22341,#22342,#22343,#22344,#22345,
#22346,#22347,#22348,#22349,#22350,#22351,#22352,#22353,#22354,#22355,#22356,
#22357,#22358,#22359,#22360,#22361,#22362,#22363,#22364,#22365,#22366,#22367,
#22368,#22369,#22370,#22371,#22372,#22373,#22374,#22375,#22376,#22377,#22378,
#22379,#22380,#22381,#22382,#22383,#22384,#22385,#22386,#22387,#22388,#22389,
#22390,#22391,#22392,#22393,#22394,#22395,#22396,#22397,#22398,#22399,#22400,
#22401,#22402,#22403,#22404,#22405,#22406,#22407),.UNSPECIFIED.,.F.,.F.)
B_SPLINE_CURVE_WITH_KNOTS((6,1,1,1,1,1,1,1,1,1,1,1,1,1,1,1,1,1,1,1,1,1,
1,1,1,1,1,1,1,1,1,1,1,1,1,1,1,1,1,1,1,1,1,1,1,1,1,1,1,1,1,1,1,1,1,1,1,1,
1,1,1,1,1,1,1,6),(0.,0.0153846153846154,0.0307692307692308,0.0461538461538462,
0.0615384615384615,0.0769230769230769,0.0923076923076923,0.107692307692308,
0.123076923076923,0.138461538461538,0.153846153846154,0.169230769230769,
0.184615384615385,0.2,0.215384615384615,0.230769230769231,0.246153846153846,
0.261538461538462,0.276923076923077,0.292307692307692,0.307692307692308,
0.323076923076923,0.338461538461538,0.353846153846154,0.369230769230769,
0.384615384615385,0.4,0.415384615384615,0.430769230769231,0.446153846153846,
0.461538461538462,0.476923076923077,0.492307692307692,0.507692307692308,
0.523076923076923,0.538461538461538,0.553846153846154,0.569230769230769,
0.584615384615384,0.6,0.615384615384615,0.63076923076923,0.646153846153846,
0.661538461538461,0.676923076923076,0.692307692307692,0.707692307692307,
0.723076923076922,0.738461538461538,0.753846153846153,0.769230769230768,
0.784615384615384,0.799999999999999,0.815384615384614,0.83076923076923,
0.846153846153845,0.86153846153846,0.876923076923076,0.892307692307691,
0.907692307692306,0.923076923076922,0.938461538461537,0.953846153846152,
0.969230769230768,0.984615384615383,1.),.UNSPECIFIED.)
CURVE()
GEOMETRIC_REPRESENTATION_ITEM()
RATIONAL_B_SPLINE_CURVE((1.,1.,1.,1.,1.,1.,1.,1.,1.,1.,1.,1.,1.,1.,1.,1.,
1.,1.,1.,1.,1.,1.,1.,1.,1.,1.,1.,1.,1.,1.,1.,1.,1.,1.,1.,1.,1.,1.,1.,1.,
1.,1.,1.,1.,1.,1.,1.,1.,1.,1.,1.,1.,1.,1.,1.,1.,1.,1.,1.,1.,1.,1.,1.,1.,
1.,1.,1.,1.,1.,1.))
REPRESENTATION_ITEM('')
);
#65=(
BOUNDED_CURVE()
B_SPLINE_CURVE(5,(#22411,#22412,#22413,#22414,#22415,#22416,#22417,#22418,
#22419,#22420,#22421,#22422,#22423,#22424,#22425,#22426,#22427,#22428,#22429,
#22430,#22431,#22432,#22433,#22434,#22435,#22436,#22437,#22438,#22439,#22440,
#22441,#22442,#22443,#22444,#22445,#22446,#22447,#22448,#22449,#22450,#22451,
#22452,#22453,#22454,#22455,#22456,#22457,#22458,#22459,#22460,#22461,#22462,
#22463,#22464,#22465,#22466,#22467,#22468,#22469,#22470,#22471,#22472,#22473,
#22474,#22475,#22476,#22477,#22478,#22479,#22480),.UNSPECIFIED.,.F.,.F.)
B_SPLINE_CURVE_WITH_KNOTS((6,1,1,1,1,1,1,1,1,1,1,1,1,1,1,1,1,1,1,1,1,1,
1,1,1,1,1,1,1,1,1,1,1,1,1,1,1,1,1,1,1,1,1,1,1,1,1,1,1,1,1,1,1,1,1,1,1,1,
1,1,1,1,1,1,1,6),(0.,0.0153846153846154,0.0307692307692308,0.0461538461538462,
0.0615384615384615,0.0769230769230769,0.0923076923076923,0.107692307692308,
0.123076923076923,0.138461538461538,0.153846153846154,0.169230769230769,
0.184615384615385,0.2,0.215384615384615,0.230769230769231,0.246153846153846,
0.261538461538462,0.276923076923077,0.292307692307692,0.307692307692308,
0.323076923076923,0.338461538461538,0.353846153846154,0.369230769230769,
0.384615384615385,0.4,0.415384615384615,0.430769230769231,0.446153846153846,
0.461538461538462,0.476923076923077,0.492307692307692,0.507692307692308,
0.523076923076923,0.538461538461538,0.553846153846154,0.569230769230769,
0.584615384615384,0.6,0.615384615384615,0.63076923076923,0.646153846153846,
0.661538461538461,0.676923076923076,0.692307692307692,0.707692307692307,
0.723076923076922,0.738461538461538,0.753846153846153,0.769230769230768,
0.784615384615384,0.799999999999999,0.815384615384614,0.83076923076923,
0.846153846153845,0.86153846153846,0.876923076923076,0.892307692307691,
0.907692307692306,0.923076923076922,0.938461538461537,0.953846153846152,
0.969230769230768,0.984615384615383,1.),.UNSPECIFIED.)
CURVE()
GEOMETRIC_REPRESENTATION_ITEM()
RATIONAL_B_SPLINE_CURVE((1.,1.,1.,1.,1.,1.,1.,1.,1.,1.,1.,1.,1.,1.,1.,1.,
1.,1.,1.,1.,1.,1.,1.,1.,1.,1.,1.,1.,1.,1.,1.,1.,1.,1.,1.,1.,1.,1.,1.,1.,
1.,1.,1.,1.,1.,1.,1.,1.,1.,1.,1.,1.,1.,1.,1.,1.,1.,1.,1.,1.,1.,1.,1.,1.,
1.,1.,1.,1.,1.,1.))
REPRESENTATION_ITEM('')
);
#66=(
BOUNDED_CURVE()
B_SPLINE_CURVE(5,(#22484,#22485,#22486,#22487,#22488,#22489,#22490,#22491,
#22492,#22493,#22494,#22495,#22496,#22497,#22498,#22499,#22500,#22501,#22502,
#22503,#22504,#22505,#22506,#22507,#22508,#22509,#22510,#22511,#22512,#22513,
#22514,#22515,#22516,#22517,#22518,#22519,#22520,#22521,#22522,#22523,#22524,
#22525,#22526,#22527,#22528,#22529,#22530,#22531,#22532,#22533,#22534,#22535,
#22536,#22537,#22538,#22539,#22540,#22541,#22542,#22543,#22544,#22545,#22546,
#22547,#22548,#22549,#22550,#22551,#22552,#22553),.UNSPECIFIED.,.F.,.F.)
B_SPLINE_CURVE_WITH_KNOTS((6,1,1,1,1,1,1,1,1,1,1,1,1,1,1,1,1,1,1,1,1,1,
1,1,1,1,1,1,1,1,1,1,1,1,1,1,1,1,1,1,1,1,1,1,1,1,1,1,1,1,1,1,1,1,1,1,1,1,
1,1,1,1,1,1,1,6),(0.,0.0153846153846154,0.0307692307692308,0.0461538461538462,
0.0615384615384615,0.0769230769230769,0.0923076923076923,0.107692307692308,
0.123076923076923,0.138461538461538,0.153846153846154,0.169230769230769,
0.184615384615385,0.2,0.215384615384615,0.230769230769231,0.246153846153846,
0.261538461538462,0.276923076923077,0.292307692307692,0.307692307692308,
0.323076923076923,0.338461538461538,0.353846153846154,0.369230769230769,
0.384615384615385,0.4,0.415384615384615,0.430769230769231,0.446153846153846,
0.461538461538462,0.476923076923077,0.492307692307692,0.507692307692308,
0.523076923076923,0.538461538461538,0.553846153846154,0.569230769230769,
0.584615384615384,0.6,0.615384615384615,0.63076923076923,0.646153846153846,
0.661538461538461,0.676923076923076,0.692307692307692,0.707692307692307,
0.723076923076922,0.738461538461538,0.753846153846153,0.769230769230768,
0.784615384615384,0.799999999999999,0.815384615384614,0.83076923076923,
0.846153846153845,0.86153846153846,0.876923076923076,0.892307692307691,
0.907692307692306,0.923076923076922,0.938461538461537,0.953846153846152,
0.969230769230768,0.984615384615383,1.),.UNSPECIFIED.)
CURVE()
GEOMETRIC_REPRESENTATION_ITEM()
RATIONAL_B_SPLINE_CURVE((1.,1.,1.,1.,1.,1.,1.,1.,1.,1.,1.,1.,1.,1.,1.,1.,
1.,1.,1.,1.,1.,1.,1.,1.,1.,1.,1.,1.,1.,1.,1.,1.,1.,1.,1.,1.,1.,1.,1.,1.,
1.,1.,1.,1.,1.,1.,1.,1.,1.,1.,1.,1.,1.,1.,1.,1.,1.,1.,1.,1.,1.,1.,1.,1.,
1.,1.,1.,1.,1.,1.))
REPRESENTATION_ITEM('')
);
#67=(
BOUNDED_CURVE()
B_SPLINE_CURVE(5,(#22557,#22558,#22559,#22560,#22561,#22562,#22563,#22564,
#22565,#22566,#22567,#22568,#22569,#22570,#22571,#22572,#22573,#22574,#22575,
#22576,#22577,#22578,#22579,#22580,#22581,#22582,#22583,#22584,#22585,#22586,
#22587,#22588,#22589,#22590,#22591,#22592,#22593,#22594,#22595,#22596,#22597,
#22598,#22599,#22600,#22601,#22602,#22603,#22604,#22605,#22606,#22607,#22608,
#22609,#22610,#22611,#22612,#22613,#22614,#22615,#22616,#22617,#22618,#22619,
#22620,#22621,#22622,#22623,#22624,#22625,#22626),.UNSPECIFIED.,.F.,.F.)
B_SPLINE_CURVE_WITH_KNOTS((6,1,1,1,1,1,1,1,1,1,1,1,1,1,1,1,1,1,1,1,1,1,
1,1,1,1,1,1,1,1,1,1,1,1,1,1,1,1,1,1,1,1,1,1,1,1,1,1,1,1,1,1,1,1,1,1,1,1,
1,1,1,1,1,1,1,6),(0.,0.0153846153846154,0.0307692307692308,0.0461538461538462,
0.0615384615384615,0.0769230769230769,0.0923076923076923,0.107692307692308,
0.123076923076923,0.138461538461538,0.153846153846154,0.169230769230769,
0.184615384615385,0.2,0.215384615384615,0.230769230769231,0.246153846153846,
0.261538461538462,0.276923076923077,0.292307692307692,0.307692307692308,
0.323076923076923,0.338461538461538,0.353846153846154,0.369230769230769,
0.384615384615385,0.4,0.415384615384615,0.430769230769231,0.446153846153846,
0.461538461538462,0.476923076923077,0.492307692307692,0.507692307692308,
0.523076923076923,0.538461538461538,0.553846153846154,0.569230769230769,
0.584615384615384,0.6,0.615384615384615,0.63076923076923,0.646153846153846,
0.661538461538461,0.676923076923076,0.692307692307692,0.707692307692307,
0.723076923076922,0.738461538461538,0.753846153846153,0.769230769230768,
0.784615384615384,0.799999999999999,0.815384615384614,0.83076923076923,
0.846153846153845,0.86153846153846,0.876923076923076,0.892307692307691,
0.907692307692306,0.923076923076922,0.938461538461537,0.953846153846152,
0.969230769230768,0.984615384615383,1.),.UNSPECIFIED.)
CURVE()
GEOMETRIC_REPRESENTATION_ITEM()
RATIONAL_B_SPLINE_CURVE((1.,1.,1.,1.,1.,1.,1.,1.,1.,1.,1.,1.,1.,1.,1.,1.,
1.,1.,1.,1.,1.,1.,1.,1.,1.,1.,1.,1.,1.,1.,1.,1.,1.,1.,1.,1.,1.,1.,1.,1.,
1.,1.,1.,1.,1.,1.,1.,1.,1.,1.,1.,1.,1.,1.,1.,1.,1.,1.,1.,1.,1.,1.,1.,1.,
1.,1.,1.,1.,1.,1.))
REPRESENTATION_ITEM('')
);
#68=(
BOUNDED_CURVE()
B_SPLINE_CURVE(5,(#22630,#22631,#22632,#22633,#22634,#22635,#22636,#22637,
#22638,#22639,#22640,#22641,#22642,#22643,#22644,#22645,#22646,#22647,#22648,
#22649,#22650,#22651,#22652,#22653,#22654,#22655,#22656,#22657,#22658,#22659,
#22660,#22661,#22662,#22663,#22664,#22665,#22666,#22667,#22668,#22669,#22670,
#22671,#22672,#22673,#22674,#22675,#22676,#22677,#22678,#22679,#22680,#22681,
#22682,#22683,#22684,#22685,#22686,#22687,#22688,#22689,#22690,#22691,#22692,
#22693,#22694,#22695,#22696,#22697,#22698,#22699),.UNSPECIFIED.,.F.,.F.)
B_SPLINE_CURVE_WITH_KNOTS((6,1,1,1,1,1,1,1,1,1,1,1,1,1,1,1,1,1,1,1,1,1,
1,1,1,1,1,1,1,1,1,1,1,1,1,1,1,1,1,1,1,1,1,1,1,1,1,1,1,1,1,1,1,1,1,1,1,1,
1,1,1,1,1,1,1,6),(0.,0.0153846153846154,0.0307692307692308,0.0461538461538462,
0.0615384615384615,0.0769230769230769,0.0923076923076923,0.107692307692308,
0.123076923076923,0.138461538461538,0.153846153846154,0.169230769230769,
0.184615384615385,0.2,0.215384615384615,0.230769230769231,0.246153846153846,
0.261538461538462,0.276923076923077,0.292307692307692,0.307692307692308,
0.323076923076923,0.338461538461538,0.353846153846154,0.369230769230769,
0.384615384615385,0.4,0.415384615384615,0.430769230769231,0.446153846153846,
0.461538461538462,0.476923076923077,0.492307692307692,0.507692307692308,
0.523076923076923,0.538461538461538,0.553846153846154,0.569230769230769,
0.584615384615384,0.6,0.615384615384615,0.63076923076923,0.646153846153846,
0.661538461538461,0.676923076923076,0.692307692307692,0.707692307692307,
0.723076923076922,0.738461538461538,0.753846153846153,0.769230769230768,
0.784615384615384,0.799999999999999,0.815384615384614,0.83076923076923,
0.846153846153845,0.86153846153846,0.876923076923076,0.892307692307691,
0.907692307692306,0.923076923076922,0.938461538461537,0.953846153846152,
0.969230769230768,0.984615384615383,1.),.UNSPECIFIED.)
CURVE()
GEOMETRIC_REPRESENTATION_ITEM()
RATIONAL_B_SPLINE_CURVE((1.,1.,1.,1.,1.,1.,1.,1.,1.,1.,1.,1.,1.,1.,1.,1.,
1.,1.,1.,1.,1.,1.,1.,1.,1.,1.,1.,1.,1.,1.,1.,1.,1.,1.,1.,1.,1.,1.,1.,1.,
1.,1.,1.,1.,1.,1.,1.,1.,1.,1.,1.,1.,1.,1.,1.,1.,1.,1.,1.,1.,1.,1.,1.,1.,
1.,1.,1.,1.,1.,1.))
REPRESENTATION_ITEM('')
);
#69=(
BOUNDED_CURVE()
B_SPLINE_CURVE(5,(#22703,#22704,#22705,#22706,#22707,#22708,#22709,#22710,
#22711,#22712,#22713,#22714,#22715,#22716,#22717,#22718,#22719,#22720,#22721,
#22722,#22723,#22724,#22725,#22726,#22727,#22728,#22729,#22730,#22731,#22732,
#22733,#22734,#22735,#22736,#22737,#22738,#22739,#22740,#22741,#22742,#22743,
#22744,#22745,#22746,#22747,#22748,#22749,#22750,#22751,#22752,#22753,#22754,
#22755,#22756,#22757,#22758,#22759,#22760,#22761,#22762,#22763,#22764,#22765,
#22766,#22767,#22768,#22769,#22770,#22771,#22772),.UNSPECIFIED.,.F.,.F.)
B_SPLINE_CURVE_WITH_KNOTS((6,1,1,1,1,1,1,1,1,1,1,1,1,1,1,1,1,1,1,1,1,1,
1,1,1,1,1,1,1,1,1,1,1,1,1,1,1,1,1,1,1,1,1,1,1,1,1,1,1,1,1,1,1,1,1,1,1,1,
1,1,1,1,1,1,1,6),(0.,0.0153846153846154,0.0307692307692308,0.0461538461538462,
0.0615384615384615,0.0769230769230769,0.0923076923076923,0.107692307692308,
0.123076923076923,0.138461538461538,0.153846153846154,0.169230769230769,
0.184615384615385,0.2,0.215384615384615,0.230769230769231,0.246153846153846,
0.261538461538462,0.276923076923077,0.292307692307692,0.307692307692308,
0.323076923076923,0.338461538461538,0.353846153846154,0.369230769230769,
0.384615384615385,0.4,0.415384615384615,0.430769230769231,0.446153846153846,
0.461538461538462,0.476923076923077,0.492307692307692,0.507692307692308,
0.523076923076923,0.538461538461538,0.553846153846154,0.569230769230769,
0.584615384615384,0.6,0.615384615384615,0.63076923076923,0.646153846153846,
0.661538461538461,0.676923076923076,0.692307692307692,0.707692307692307,
0.723076923076922,0.738461538461538,0.753846153846153,0.769230769230768,
0.784615384615384,0.799999999999999,0.815384615384614,0.83076923076923,
0.846153846153845,0.86153846153846,0.876923076923076,0.892307692307691,
0.907692307692306,0.923076923076922,0.938461538461537,0.953846153846152,
0.969230769230768,0.984615384615383,1.),.UNSPECIFIED.)
CURVE()
GEOMETRIC_REPRESENTATION_ITEM()
RATIONAL_B_SPLINE_CURVE((1.,1.,1.,1.,1.,1.,1.,1.,1.,1.,1.,1.,1.,1.,1.,1.,
1.,1.,1.,1.,1.,1.,1.,1.,1.,1.,1.,1.,1.,1.,1.,1.,1.,1.,1.,1.,1.,1.,1.,1.,
1.,1.,1.,1.,1.,1.,1.,1.,1.,1.,1.,1.,1.,1.,1.,1.,1.,1.,1.,1.,1.,1.,1.,1.,
1.,1.,1.,1.,1.,1.))
REPRESENTATION_ITEM('')
);
#70=(
BOUNDED_CURVE()
B_SPLINE_CURVE(5,(#22776,#22777,#22778,#22779,#22780,#22781,#22782,#22783,
#22784,#22785,#22786,#22787,#22788,#22789,#22790,#22791,#22792,#22793,#22794,
#22795,#22796,#22797,#22798,#22799,#22800,#22801,#22802,#22803,#22804,#22805,
#22806,#22807,#22808,#22809,#22810,#22811,#22812,#22813,#22814,#22815,#22816,
#22817,#22818,#22819,#22820,#22821,#22822,#22823,#22824,#22825,#22826,#22827,
#22828,#22829,#22830,#22831,#22832,#22833,#22834,#22835,#22836,#22837,#22838,
#22839,#22840,#22841,#22842,#22843,#22844,#22845),.UNSPECIFIED.,.F.,.F.)
B_SPLINE_CURVE_WITH_KNOTS((6,1,1,1,1,1,1,1,1,1,1,1,1,1,1,1,1,1,1,1,1,1,
1,1,1,1,1,1,1,1,1,1,1,1,1,1,1,1,1,1,1,1,1,1,1,1,1,1,1,1,1,1,1,1,1,1,1,1,
1,1,1,1,1,1,1,6),(0.,0.0153846153846154,0.0307692307692308,0.0461538461538462,
0.0615384615384615,0.0769230769230769,0.0923076923076923,0.107692307692308,
0.123076923076923,0.138461538461538,0.153846153846154,0.169230769230769,
0.184615384615385,0.2,0.215384615384615,0.230769230769231,0.246153846153846,
0.261538461538462,0.276923076923077,0.292307692307692,0.307692307692308,
0.323076923076923,0.338461538461538,0.353846153846154,0.369230769230769,
0.384615384615385,0.4,0.415384615384615,0.430769230769231,0.446153846153846,
0.461538461538462,0.476923076923077,0.492307692307692,0.507692307692308,
0.523076923076923,0.538461538461538,0.553846153846154,0.569230769230769,
0.584615384615384,0.6,0.615384615384615,0.63076923076923,0.646153846153846,
0.661538461538461,0.676923076923076,0.692307692307692,0.707692307692307,
0.723076923076922,0.738461538461538,0.753846153846153,0.769230769230768,
0.784615384615384,0.799999999999999,0.815384615384614,0.83076923076923,
0.846153846153845,0.86153846153846,0.876923076923076,0.892307692307691,
0.907692307692306,0.923076923076922,0.938461538461537,0.953846153846152,
0.969230769230768,0.984615384615383,1.),.UNSPECIFIED.)
CURVE()
GEOMETRIC_REPRESENTATION_ITEM()
RATIONAL_B_SPLINE_CURVE((1.,1.,1.,1.,1.,1.,1.,1.,1.,1.,1.,1.,1.,1.,1.,1.,
1.,1.,1.,1.,1.,1.,1.,1.,1.,1.,1.,1.,1.,1.,1.,1.,1.,1.,1.,1.,1.,1.,1.,1.,
1.,1.,1.,1.,1.,1.,1.,1.,1.,1.,1.,1.,1.,1.,1.,1.,1.,1.,1.,1.,1.,1.,1.,1.,
1.,1.,1.,1.,1.,1.))
REPRESENTATION_ITEM('')
);
#71=(
BOUNDED_CURVE()
B_SPLINE_CURVE(5,(#22849,#22850,#22851,#22852,#22853,#22854,#22855,#22856,
#22857,#22858,#22859,#22860,#22861,#22862,#22863,#22864,#22865,#22866,#22867,
#22868,#22869,#22870,#22871,#22872,#22873,#22874,#22875,#22876,#22877,#22878,
#22879,#22880,#22881,#22882,#22883,#22884,#22885,#22886,#22887,#22888,#22889,
#22890,#22891,#22892,#22893,#22894,#22895,#22896,#22897,#22898,#22899,#22900,
#22901,#22902,#22903,#22904,#22905,#22906,#22907,#22908,#22909,#22910,#22911,
#22912,#22913,#22914,#22915,#22916,#22917,#22918),.UNSPECIFIED.,.F.,.F.)
B_SPLINE_CURVE_WITH_KNOTS((6,1,1,1,1,1,1,1,1,1,1,1,1,1,1,1,1,1,1,1,1,1,
1,1,1,1,1,1,1,1,1,1,1,1,1,1,1,1,1,1,1,1,1,1,1,1,1,1,1,1,1,1,1,1,1,1,1,1,
1,1,1,1,1,1,1,6),(0.,0.0153846153846154,0.0307692307692308,0.0461538461538462,
0.0615384615384615,0.0769230769230769,0.0923076923076923,0.107692307692308,
0.123076923076923,0.138461538461538,0.153846153846154,0.169230769230769,
0.184615384615385,0.2,0.215384615384615,0.230769230769231,0.246153846153846,
0.261538461538462,0.276923076923077,0.292307692307692,0.307692307692308,
0.323076923076923,0.338461538461538,0.353846153846154,0.369230769230769,
0.384615384615385,0.4,0.415384615384615,0.430769230769231,0.446153846153846,
0.461538461538462,0.476923076923077,0.492307692307692,0.507692307692308,
0.523076923076923,0.538461538461538,0.553846153846154,0.569230769230769,
0.584615384615384,0.6,0.615384615384615,0.63076923076923,0.646153846153846,
0.661538461538461,0.676923076923076,0.692307692307692,0.707692307692307,
0.723076923076922,0.738461538461538,0.753846153846153,0.769230769230768,
0.784615384615384,0.799999999999999,0.815384615384614,0.83076923076923,
0.846153846153845,0.86153846153846,0.876923076923076,0.892307692307691,
0.907692307692306,0.923076923076922,0.938461538461537,0.953846153846152,
0.969230769230768,0.984615384615383,1.),.UNSPECIFIED.)
CURVE()
GEOMETRIC_REPRESENTATION_ITEM()
RATIONAL_B_SPLINE_CURVE((1.,1.,1.,1.,1.,1.,1.,1.,1.,1.,1.,1.,1.,1.,1.,1.,
1.,1.,1.,1.,1.,1.,1.,1.,1.,1.,1.,1.,1.,1.,1.,1.,1.,1.,1.,1.,1.,1.,1.,1.,
1.,1.,1.,1.,1.,1.,1.,1.,1.,1.,1.,1.,1.,1.,1.,1.,1.,1.,1.,1.,1.,1.,1.,1.,
1.,1.,1.,1.,1.,1.))
REPRESENTATION_ITEM('')
);
#72=(
BOUNDED_CURVE()
B_SPLINE_CURVE(5,(#22922,#22923,#22924,#22925,#22926,#22927,#22928,#22929,
#22930,#22931,#22932,#22933,#22934,#22935,#22936,#22937,#22938,#22939,#22940,
#22941,#22942,#22943,#22944,#22945,#22946,#22947,#22948,#22949,#22950,#22951,
#22952,#22953,#22954,#22955,#22956,#22957,#22958,#22959,#22960,#22961,#22962,
#22963,#22964,#22965,#22966,#22967,#22968,#22969,#22970,#22971,#22972,#22973,
#22974,#22975,#22976,#22977,#22978,#22979,#22980,#22981,#22982,#22983,#22984,
#22985,#22986,#22987,#22988,#22989,#22990,#22991),.UNSPECIFIED.,.F.,.F.)
B_SPLINE_CURVE_WITH_KNOTS((6,1,1,1,1,1,1,1,1,1,1,1,1,1,1,1,1,1,1,1,1,1,
1,1,1,1,1,1,1,1,1,1,1,1,1,1,1,1,1,1,1,1,1,1,1,1,1,1,1,1,1,1,1,1,1,1,1,1,
1,1,1,1,1,1,1,6),(0.,0.0153846153846154,0.0307692307692308,0.0461538461538462,
0.0615384615384615,0.0769230769230769,0.0923076923076923,0.107692307692308,
0.123076923076923,0.138461538461538,0.153846153846154,0.169230769230769,
0.184615384615385,0.2,0.215384615384615,0.230769230769231,0.246153846153846,
0.261538461538462,0.276923076923077,0.292307692307692,0.307692307692308,
0.323076923076923,0.338461538461538,0.353846153846154,0.369230769230769,
0.384615384615385,0.4,0.415384615384615,0.430769230769231,0.446153846153846,
0.461538461538462,0.476923076923077,0.492307692307692,0.507692307692308,
0.523076923076923,0.538461538461538,0.553846153846154,0.569230769230769,
0.584615384615384,0.6,0.615384615384615,0.63076923076923,0.646153846153846,
0.661538461538461,0.676923076923076,0.692307692307692,0.707692307692307,
0.723076923076922,0.738461538461538,0.753846153846153,0.769230769230768,
0.784615384615384,0.799999999999999,0.815384615384614,0.83076923076923,
0.846153846153845,0.86153846153846,0.876923076923076,0.892307692307691,
0.907692307692306,0.923076923076922,0.938461538461537,0.953846153846152,
0.969230769230768,0.984615384615383,1.),.UNSPECIFIED.)
CURVE()
GEOMETRIC_REPRESENTATION_ITEM()
RATIONAL_B_SPLINE_CURVE((1.,1.,1.,1.,1.,1.,1.,1.,1.,1.,1.,1.,1.,1.,1.,1.,
1.,1.,1.,1.,1.,1.,1.,1.,1.,1.,1.,1.,1.,1.,1.,1.,1.,1.,1.,1.,1.,1.,1.,1.,
1.,1.,1.,1.,1.,1.,1.,1.,1.,1.,1.,1.,1.,1.,1.,1.,1.,1.,1.,1.,1.,1.,1.,1.,
1.,1.,1.,1.,1.,1.))
REPRESENTATION_ITEM('')
);
#73=(
BOUNDED_CURVE()
B_SPLINE_CURVE(5,(#22995,#22996,#22997,#22998,#22999,#23000,#23001,#23002,
#23003,#23004,#23005,#23006,#23007,#23008,#23009,#23010,#23011,#23012,#23013,
#23014,#23015,#23016,#23017,#23018,#23019,#23020,#23021,#23022,#23023,#23024,
#23025,#23026,#23027,#23028,#23029,#23030,#23031,#23032,#23033,#23034,#23035,
#23036,#23037,#23038,#23039,#23040,#23041,#23042,#23043,#23044,#23045,#23046,
#23047,#23048,#23049,#23050,#23051,#23052,#23053,#23054,#23055,#23056,#23057,
#23058,#23059,#23060,#23061,#23062,#23063,#23064),.UNSPECIFIED.,.F.,.F.)
B_SPLINE_CURVE_WITH_KNOTS((6,1,1,1,1,1,1,1,1,1,1,1,1,1,1,1,1,1,1,1,1,1,
1,1,1,1,1,1,1,1,1,1,1,1,1,1,1,1,1,1,1,1,1,1,1,1,1,1,1,1,1,1,1,1,1,1,1,1,
1,1,1,1,1,1,1,6),(0.,0.0153846153846154,0.0307692307692308,0.0461538461538462,
0.0615384615384615,0.0769230769230769,0.0923076923076923,0.107692307692308,
0.123076923076923,0.138461538461538,0.153846153846154,0.169230769230769,
0.184615384615385,0.2,0.215384615384615,0.230769230769231,0.246153846153846,
0.261538461538462,0.276923076923077,0.292307692307692,0.307692307692308,
0.323076923076923,0.338461538461538,0.353846153846154,0.369230769230769,
0.384615384615385,0.4,0.415384615384615,0.430769230769231,0.446153846153846,
0.461538461538462,0.476923076923077,0.492307692307692,0.507692307692308,
0.523076923076923,0.538461538461538,0.553846153846154,0.569230769230769,
0.584615384615384,0.6,0.615384615384615,0.63076923076923,0.646153846153846,
0.661538461538461,0.676923076923076,0.692307692307692,0.707692307692307,
0.723076923076922,0.738461538461538,0.753846153846153,0.769230769230768,
0.784615384615384,0.799999999999999,0.815384615384614,0.83076923076923,
0.846153846153845,0.86153846153846,0.876923076923076,0.892307692307691,
0.907692307692306,0.923076923076922,0.938461538461537,0.953846153846152,
0.969230769230768,0.984615384615383,1.),.UNSPECIFIED.)
CURVE()
GEOMETRIC_REPRESENTATION_ITEM()
RATIONAL_B_SPLINE_CURVE((1.,1.,1.,1.,1.,1.,1.,1.,1.,1.,1.,1.,1.,1.,1.,1.,
1.,1.,1.,1.,1.,1.,1.,1.,1.,1.,1.,1.,1.,1.,1.,1.,1.,1.,1.,1.,1.,1.,1.,1.,
1.,1.,1.,1.,1.,1.,1.,1.,1.,1.,1.,1.,1.,1.,1.,1.,1.,1.,1.,1.,1.,1.,1.,1.,
1.,1.,1.,1.,1.,1.))
REPRESENTATION_ITEM('')
);
#74=(
BOUNDED_CURVE()
B_SPLINE_CURVE(5,(#23068,#23069,#23070,#23071,#23072,#23073,#23074,#23075,
#23076,#23077,#23078,#23079,#23080,#23081,#23082,#23083,#23084,#23085,#23086,
#23087,#23088,#23089,#23090,#23091,#23092,#23093,#23094,#23095,#23096,#23097,
#23098,#23099,#23100,#23101,#23102,#23103,#23104,#23105,#23106,#23107,#23108,
#23109,#23110,#23111,#23112,#23113,#23114,#23115,#23116,#23117,#23118,#23119,
#23120,#23121,#23122,#23123,#23124,#23125,#23126,#23127,#23128,#23129,#23130,
#23131,#23132,#23133,#23134,#23135,#23136,#23137),.UNSPECIFIED.,.F.,.F.)
B_SPLINE_CURVE_WITH_KNOTS((6,1,1,1,1,1,1,1,1,1,1,1,1,1,1,1,1,1,1,1,1,1,
1,1,1,1,1,1,1,1,1,1,1,1,1,1,1,1,1,1,1,1,1,1,1,1,1,1,1,1,1,1,1,1,1,1,1,1,
1,1,1,1,1,1,1,6),(0.,0.0153846153846154,0.0307692307692308,0.0461538461538462,
0.0615384615384615,0.0769230769230769,0.0923076923076923,0.107692307692308,
0.123076923076923,0.138461538461538,0.153846153846154,0.169230769230769,
0.184615384615385,0.2,0.215384615384615,0.230769230769231,0.246153846153846,
0.261538461538462,0.276923076923077,0.292307692307692,0.307692307692308,
0.323076923076923,0.338461538461538,0.353846153846154,0.369230769230769,
0.384615384615385,0.4,0.415384615384615,0.430769230769231,0.446153846153846,
0.461538461538462,0.476923076923077,0.492307692307692,0.507692307692308,
0.523076923076923,0.538461538461538,0.553846153846154,0.569230769230769,
0.584615384615384,0.6,0.615384615384615,0.63076923076923,0.646153846153846,
0.661538461538461,0.676923076923076,0.692307692307692,0.707692307692307,
0.723076923076922,0.738461538461538,0.753846153846153,0.769230769230768,
0.784615384615384,0.799999999999999,0.815384615384614,0.83076923076923,
0.846153846153845,0.86153846153846,0.876923076923076,0.892307692307691,
0.907692307692306,0.923076923076922,0.938461538461537,0.953846153846152,
0.969230769230768,0.984615384615383,1.),.UNSPECIFIED.)
CURVE()
GEOMETRIC_REPRESENTATION_ITEM()
RATIONAL_B_SPLINE_CURVE((1.,1.,1.,1.,1.,1.,1.,1.,1.,1.,1.,1.,1.,1.,1.,1.,
1.,1.,1.,1.,1.,1.,1.,1.,1.,1.,1.,1.,1.,1.,1.,1.,1.,1.,1.,1.,1.,1.,1.,1.,
1.,1.,1.,1.,1.,1.,1.,1.,1.,1.,1.,1.,1.,1.,1.,1.,1.,1.,1.,1.,1.,1.,1.,1.,
1.,1.,1.,1.,1.,1.))
REPRESENTATION_ITEM('')
);
#75=(
BOUNDED_CURVE()
B_SPLINE_CURVE(5,(#23141,#23142,#23143,#23144,#23145,#23146,#23147,#23148,
#23149,#23150,#23151,#23152,#23153,#23154,#23155,#23156,#23157,#23158,#23159,
#23160,#23161,#23162,#23163,#23164,#23165,#23166,#23167,#23168,#23169,#23170,
#23171,#23172,#23173,#23174,#23175,#23176,#23177,#23178,#23179,#23180,#23181,
#23182,#23183,#23184,#23185,#23186,#23187,#23188,#23189,#23190,#23191,#23192,
#23193,#23194,#23195,#23196,#23197,#23198,#23199,#23200,#23201,#23202,#23203,
#23204,#23205,#23206,#23207,#23208,#23209,#23210),.UNSPECIFIED.,.F.,.F.)
B_SPLINE_CURVE_WITH_KNOTS((6,1,1,1,1,1,1,1,1,1,1,1,1,1,1,1,1,1,1,1,1,1,
1,1,1,1,1,1,1,1,1,1,1,1,1,1,1,1,1,1,1,1,1,1,1,1,1,1,1,1,1,1,1,1,1,1,1,1,
1,1,1,1,1,1,1,6),(0.,0.0153846153846154,0.0307692307692308,0.0461538461538462,
0.0615384615384615,0.0769230769230769,0.0923076923076923,0.107692307692308,
0.123076923076923,0.138461538461538,0.153846153846154,0.169230769230769,
0.184615384615385,0.2,0.215384615384615,0.230769230769231,0.246153846153846,
0.261538461538462,0.276923076923077,0.292307692307692,0.307692307692308,
0.323076923076923,0.338461538461538,0.353846153846154,0.369230769230769,
0.384615384615385,0.4,0.415384615384615,0.430769230769231,0.446153846153846,
0.461538461538462,0.476923076923077,0.492307692307692,0.507692307692308,
0.523076923076923,0.538461538461538,0.553846153846154,0.569230769230769,
0.584615384615384,0.6,0.615384615384615,0.63076923076923,0.646153846153846,
0.661538461538461,0.676923076923076,0.692307692307692,0.707692307692307,
0.723076923076922,0.738461538461538,0.753846153846153,0.769230769230768,
0.784615384615384,0.799999999999999,0.815384615384614,0.83076923076923,
0.846153846153845,0.86153846153846,0.876923076923076,0.892307692307691,
0.907692307692306,0.923076923076922,0.938461538461537,0.953846153846152,
0.969230769230768,0.984615384615383,1.),.UNSPECIFIED.)
CURVE()
GEOMETRIC_REPRESENTATION_ITEM()
RATIONAL_B_SPLINE_CURVE((1.,1.,1.,1.,1.,1.,1.,1.,1.,1.,1.,1.,1.,1.,1.,1.,
1.,1.,1.,1.,1.,1.,1.,1.,1.,1.,1.,1.,1.,1.,1.,1.,1.,1.,1.,1.,1.,1.,1.,1.,
1.,1.,1.,1.,1.,1.,1.,1.,1.,1.,1.,1.,1.,1.,1.,1.,1.,1.,1.,1.,1.,1.,1.,1.,
1.,1.,1.,1.,1.,1.))
REPRESENTATION_ITEM('')
);
#76=(
BOUNDED_CURVE()
B_SPLINE_CURVE(5,(#23214,#23215,#23216,#23217,#23218,#23219,#23220,#23221,
#23222,#23223,#23224,#23225,#23226,#23227,#23228,#23229,#23230,#23231,#23232,
#23233,#23234,#23235,#23236,#23237,#23238,#23239,#23240,#23241,#23242,#23243,
#23244,#23245,#23246,#23247,#23248,#23249,#23250,#23251,#23252,#23253,#23254,
#23255,#23256,#23257,#23258,#23259,#23260,#23261,#23262,#23263,#23264,#23265,
#23266,#23267,#23268,#23269,#23270,#23271,#23272,#23273,#23274,#23275,#23276,
#23277,#23278,#23279,#23280,#23281,#23282,#23283),.UNSPECIFIED.,.F.,.F.)
B_SPLINE_CURVE_WITH_KNOTS((6,1,1,1,1,1,1,1,1,1,1,1,1,1,1,1,1,1,1,1,1,1,
1,1,1,1,1,1,1,1,1,1,1,1,1,1,1,1,1,1,1,1,1,1,1,1,1,1,1,1,1,1,1,1,1,1,1,1,
1,1,1,1,1,1,1,6),(0.,0.0153846153846154,0.0307692307692308,0.0461538461538462,
0.0615384615384615,0.0769230769230769,0.0923076923076923,0.107692307692308,
0.123076923076923,0.138461538461538,0.153846153846154,0.169230769230769,
0.184615384615385,0.2,0.215384615384615,0.230769230769231,0.246153846153846,
0.261538461538462,0.276923076923077,0.292307692307692,0.307692307692308,
0.323076923076923,0.338461538461538,0.353846153846154,0.369230769230769,
0.384615384615385,0.4,0.415384615384615,0.430769230769231,0.446153846153846,
0.461538461538462,0.476923076923077,0.492307692307692,0.507692307692308,
0.523076923076923,0.538461538461538,0.553846153846154,0.569230769230769,
0.584615384615384,0.6,0.615384615384615,0.63076923076923,0.646153846153846,
0.661538461538461,0.676923076923076,0.692307692307692,0.707692307692307,
0.723076923076922,0.738461538461538,0.753846153846153,0.769230769230768,
0.784615384615384,0.799999999999999,0.815384615384614,0.83076923076923,
0.846153846153845,0.86153846153846,0.876923076923076,0.892307692307691,
0.907692307692306,0.923076923076922,0.938461538461537,0.953846153846152,
0.969230769230768,0.984615384615383,1.),.UNSPECIFIED.)
CURVE()
GEOMETRIC_REPRESENTATION_ITEM()
RATIONAL_B_SPLINE_CURVE((1.,1.,1.,1.,1.,1.,1.,1.,1.,1.,1.,1.,1.,1.,1.,1.,
1.,1.,1.,1.,1.,1.,1.,1.,1.,1.,1.,1.,1.,1.,1.,1.,1.,1.,1.,1.,1.,1.,1.,1.,
1.,1.,1.,1.,1.,1.,1.,1.,1.,1.,1.,1.,1.,1.,1.,1.,1.,1.,1.,1.,1.,1.,1.,1.,
1.,1.,1.,1.,1.,1.))
REPRESENTATION_ITEM('')
);
#77=(
BOUNDED_CURVE()
B_SPLINE_CURVE(5,(#23287,#23288,#23289,#23290,#23291,#23292,#23293,#23294,
#23295,#23296,#23297,#23298,#23299,#23300,#23301,#23302,#23303,#23304,#23305,
#23306,#23307,#23308,#23309,#23310,#23311,#23312,#23313,#23314,#23315,#23316,
#23317,#23318,#23319,#23320,#23321,#23322,#23323,#23324,#23325,#23326,#23327,
#23328,#23329,#23330,#23331,#23332,#23333,#23334,#23335,#23336,#23337,#23338,
#23339,#23340,#23341,#23342,#23343,#23344,#23345,#23346,#23347,#23348,#23349,
#23350,#23351,#23352,#23353,#23354,#23355,#23356),.UNSPECIFIED.,.F.,.F.)
B_SPLINE_CURVE_WITH_KNOTS((6,1,1,1,1,1,1,1,1,1,1,1,1,1,1,1,1,1,1,1,1,1,
1,1,1,1,1,1,1,1,1,1,1,1,1,1,1,1,1,1,1,1,1,1,1,1,1,1,1,1,1,1,1,1,1,1,1,1,
1,1,1,1,1,1,1,6),(0.,0.0153846153846154,0.0307692307692308,0.0461538461538462,
0.0615384615384615,0.0769230769230769,0.0923076923076923,0.107692307692308,
0.123076923076923,0.138461538461538,0.153846153846154,0.169230769230769,
0.184615384615385,0.2,0.215384615384615,0.230769230769231,0.246153846153846,
0.261538461538462,0.276923076923077,0.292307692307692,0.307692307692308,
0.323076923076923,0.338461538461538,0.353846153846154,0.369230769230769,
0.384615384615385,0.4,0.415384615384615,0.430769230769231,0.446153846153846,
0.461538461538462,0.476923076923077,0.492307692307692,0.507692307692308,
0.523076923076923,0.538461538461538,0.553846153846154,0.569230769230769,
0.584615384615384,0.6,0.615384615384615,0.63076923076923,0.646153846153846,
0.661538461538461,0.676923076923076,0.692307692307692,0.707692307692307,
0.723076923076922,0.738461538461538,0.753846153846153,0.769230769230768,
0.784615384615384,0.799999999999999,0.815384615384614,0.83076923076923,
0.846153846153845,0.86153846153846,0.876923076923076,0.892307692307691,
0.907692307692306,0.923076923076922,0.938461538461537,0.953846153846152,
0.969230769230768,0.984615384615383,1.),.UNSPECIFIED.)
CURVE()
GEOMETRIC_REPRESENTATION_ITEM()
RATIONAL_B_SPLINE_CURVE((1.,1.,1.,1.,1.,1.,1.,1.,1.,1.,1.,1.,1.,1.,1.,1.,
1.,1.,1.,1.,1.,1.,1.,1.,1.,1.,1.,1.,1.,1.,1.,1.,1.,1.,1.,1.,1.,1.,1.,1.,
1.,1.,1.,1.,1.,1.,1.,1.,1.,1.,1.,1.,1.,1.,1.,1.,1.,1.,1.,1.,1.,1.,1.,1.,
1.,1.,1.,1.,1.,1.))
REPRESENTATION_ITEM('')
);
#78=(
BOUNDED_CURVE()
B_SPLINE_CURVE(5,(#23360,#23361,#23362,#23363,#23364,#23365,#23366,#23367,
#23368,#23369,#23370,#23371,#23372,#23373,#23374,#23375,#23376,#23377,#23378,
#23379,#23380,#23381,#23382,#23383,#23384,#23385,#23386,#23387,#23388,#23389,
#23390,#23391,#23392,#23393,#23394,#23395,#23396,#23397,#23398,#23399,#23400,
#23401,#23402,#23403,#23404,#23405,#23406,#23407,#23408,#23409,#23410,#23411,
#23412,#23413,#23414,#23415,#23416,#23417,#23418,#23419,#23420,#23421,#23422,
#23423,#23424,#23425,#23426,#23427,#23428,#23429),.UNSPECIFIED.,.F.,.F.)
B_SPLINE_CURVE_WITH_KNOTS((6,1,1,1,1,1,1,1,1,1,1,1,1,1,1,1,1,1,1,1,1,1,
1,1,1,1,1,1,1,1,1,1,1,1,1,1,1,1,1,1,1,1,1,1,1,1,1,1,1,1,1,1,1,1,1,1,1,1,
1,1,1,1,1,1,1,6),(0.,0.0153846153846154,0.0307692307692308,0.0461538461538462,
0.0615384615384615,0.0769230769230769,0.0923076923076923,0.107692307692308,
0.123076923076923,0.138461538461538,0.153846153846154,0.169230769230769,
0.184615384615385,0.2,0.215384615384615,0.230769230769231,0.246153846153846,
0.261538461538462,0.276923076923077,0.292307692307692,0.307692307692308,
0.323076923076923,0.338461538461538,0.353846153846154,0.369230769230769,
0.384615384615385,0.4,0.415384615384615,0.430769230769231,0.446153846153846,
0.461538461538462,0.476923076923077,0.492307692307692,0.507692307692308,
0.523076923076923,0.538461538461538,0.553846153846154,0.569230769230769,
0.584615384615384,0.6,0.615384615384615,0.63076923076923,0.646153846153846,
0.661538461538461,0.676923076923076,0.692307692307692,0.707692307692307,
0.723076923076922,0.738461538461538,0.753846153846153,0.769230769230768,
0.784615384615384,0.799999999999999,0.815384615384614,0.83076923076923,
0.846153846153845,0.86153846153846,0.876923076923076,0.892307692307691,
0.907692307692306,0.923076923076922,0.938461538461537,0.953846153846152,
0.969230769230768,0.984615384615383,1.),.UNSPECIFIED.)
CURVE()
GEOMETRIC_REPRESENTATION_ITEM()
RATIONAL_B_SPLINE_CURVE((1.,1.,1.,1.,1.,1.,1.,1.,1.,1.,1.,1.,1.,1.,1.,1.,
1.,1.,1.,1.,1.,1.,1.,1.,1.,1.,1.,1.,1.,1.,1.,1.,1.,1.,1.,1.,1.,1.,1.,1.,
1.,1.,1.,1.,1.,1.,1.,1.,1.,1.,1.,1.,1.,1.,1.,1.,1.,1.,1.,1.,1.,1.,1.,1.,
1.,1.,1.,1.,1.,1.))
REPRESENTATION_ITEM('')
);
#79=(
BOUNDED_CURVE()
B_SPLINE_CURVE(5,(#23433,#23434,#23435,#23436,#23437,#23438,#23439,#23440,
#23441,#23442,#23443,#23444,#23445,#23446,#23447,#23448,#23449,#23450,#23451,
#23452,#23453,#23454,#23455,#23456,#23457,#23458,#23459,#23460,#23461,#23462,
#23463,#23464,#23465,#23466,#23467,#23468,#23469,#23470,#23471,#23472,#23473,
#23474,#23475,#23476,#23477,#23478,#23479,#23480,#23481,#23482,#23483,#23484,
#23485,#23486,#23487,#23488,#23489,#23490,#23491,#23492,#23493,#23494,#23495,
#23496,#23497,#23498,#23499,#23500,#23501,#23502),.UNSPECIFIED.,.F.,.F.)
B_SPLINE_CURVE_WITH_KNOTS((6,1,1,1,1,1,1,1,1,1,1,1,1,1,1,1,1,1,1,1,1,1,
1,1,1,1,1,1,1,1,1,1,1,1,1,1,1,1,1,1,1,1,1,1,1,1,1,1,1,1,1,1,1,1,1,1,1,1,
1,1,1,1,1,1,1,6),(0.,0.0153846153846154,0.0307692307692308,0.0461538461538462,
0.0615384615384615,0.0769230769230769,0.0923076923076923,0.107692307692308,
0.123076923076923,0.138461538461538,0.153846153846154,0.169230769230769,
0.184615384615385,0.2,0.215384615384615,0.230769230769231,0.246153846153846,
0.261538461538462,0.276923076923077,0.292307692307692,0.307692307692308,
0.323076923076923,0.338461538461538,0.353846153846154,0.369230769230769,
0.384615384615385,0.4,0.415384615384615,0.430769230769231,0.446153846153846,
0.461538461538462,0.476923076923077,0.492307692307692,0.507692307692308,
0.523076923076923,0.538461538461538,0.553846153846154,0.569230769230769,
0.584615384615384,0.6,0.615384615384615,0.63076923076923,0.646153846153846,
0.661538461538461,0.676923076923076,0.692307692307692,0.707692307692307,
0.723076923076922,0.738461538461538,0.753846153846153,0.769230769230768,
0.784615384615384,0.799999999999999,0.815384615384614,0.83076923076923,
0.846153846153845,0.86153846153846,0.876923076923076,0.892307692307691,
0.907692307692306,0.923076923076922,0.938461538461537,0.953846153846152,
0.969230769230768,0.984615384615383,1.),.UNSPECIFIED.)
CURVE()
GEOMETRIC_REPRESENTATION_ITEM()
RATIONAL_B_SPLINE_CURVE((1.,1.,1.,1.,1.,1.,1.,1.,1.,1.,1.,1.,1.,1.,1.,1.,
1.,1.,1.,1.,1.,1.,1.,1.,1.,1.,1.,1.,1.,1.,1.,1.,1.,1.,1.,1.,1.,1.,1.,1.,
1.,1.,1.,1.,1.,1.,1.,1.,1.,1.,1.,1.,1.,1.,1.,1.,1.,1.,1.,1.,1.,1.,1.,1.,
1.,1.,1.,1.,1.,1.))
REPRESENTATION_ITEM('')
);
#80=(
BOUNDED_CURVE()
B_SPLINE_CURVE(5,(#23506,#23507,#23508,#23509,#23510,#23511,#23512,#23513,
#23514,#23515,#23516,#23517,#23518,#23519,#23520,#23521,#23522,#23523,#23524,
#23525,#23526,#23527,#23528,#23529,#23530,#23531,#23532,#23533,#23534,#23535,
#23536,#23537,#23538,#23539,#23540,#23541,#23542,#23543,#23544,#23545,#23546,
#23547,#23548,#23549,#23550,#23551,#23552,#23553,#23554,#23555,#23556,#23557,
#23558,#23559,#23560,#23561,#23562,#23563,#23564,#23565,#23566,#23567,#23568,
#23569,#23570,#23571,#23572,#23573,#23574,#23575),.UNSPECIFIED.,.F.,.F.)
B_SPLINE_CURVE_WITH_KNOTS((6,1,1,1,1,1,1,1,1,1,1,1,1,1,1,1,1,1,1,1,1,1,
1,1,1,1,1,1,1,1,1,1,1,1,1,1,1,1,1,1,1,1,1,1,1,1,1,1,1,1,1,1,1,1,1,1,1,1,
1,1,1,1,1,1,1,6),(0.,0.0153846153846154,0.0307692307692308,0.0461538461538462,
0.0615384615384615,0.0769230769230769,0.0923076923076923,0.107692307692308,
0.123076923076923,0.138461538461538,0.153846153846154,0.169230769230769,
0.184615384615385,0.2,0.215384615384615,0.230769230769231,0.246153846153846,
0.261538461538462,0.276923076923077,0.292307692307692,0.307692307692308,
0.323076923076923,0.338461538461538,0.353846153846154,0.369230769230769,
0.384615384615385,0.4,0.415384615384615,0.430769230769231,0.446153846153846,
0.461538461538462,0.476923076923077,0.492307692307692,0.507692307692308,
0.523076923076923,0.538461538461538,0.553846153846154,0.569230769230769,
0.584615384615384,0.6,0.615384615384615,0.63076923076923,0.646153846153846,
0.661538461538461,0.676923076923076,0.692307692307692,0.707692307692307,
0.723076923076922,0.738461538461538,0.753846153846153,0.769230769230768,
0.784615384615384,0.799999999999999,0.815384615384614,0.83076923076923,
0.846153846153845,0.86153846153846,0.876923076923076,0.892307692307691,
0.907692307692306,0.923076923076922,0.938461538461537,0.953846153846152,
0.969230769230768,0.984615384615383,1.),.UNSPECIFIED.)
CURVE()
GEOMETRIC_REPRESENTATION_ITEM()
RATIONAL_B_SPLINE_CURVE((1.,1.,1.,1.,1.,1.,1.,1.,1.,1.,1.,1.,1.,1.,1.,1.,
1.,1.,1.,1.,1.,1.,1.,1.,1.,1.,1.,1.,1.,1.,1.,1.,1.,1.,1.,1.,1.,1.,1.,1.,
1.,1.,1.,1.,1.,1.,1.,1.,1.,1.,1.,1.,1.,1.,1.,1.,1.,1.,1.,1.,1.,1.,1.,1.,
1.,1.,1.,1.,1.,1.))
REPRESENTATION_ITEM('')
);
#81=(
BOUNDED_CURVE()
B_SPLINE_CURVE(5,(#23579,#23580,#23581,#23582,#23583,#23584,#23585,#23586,
#23587,#23588,#23589,#23590,#23591,#23592,#23593,#23594,#23595,#23596,#23597,
#23598,#23599,#23600,#23601,#23602,#23603,#23604,#23605,#23606,#23607,#23608,
#23609,#23610,#23611,#23612,#23613,#23614,#23615,#23616,#23617,#23618,#23619,
#23620,#23621,#23622,#23623,#23624,#23625,#23626,#23627,#23628,#23629,#23630,
#23631,#23632,#23633,#23634,#23635,#23636,#23637,#23638,#23639,#23640,#23641,
#23642,#23643,#23644,#23645,#23646,#23647,#23648),.UNSPECIFIED.,.F.,.F.)
B_SPLINE_CURVE_WITH_KNOTS((6,1,1,1,1,1,1,1,1,1,1,1,1,1,1,1,1,1,1,1,1,1,
1,1,1,1,1,1,1,1,1,1,1,1,1,1,1,1,1,1,1,1,1,1,1,1,1,1,1,1,1,1,1,1,1,1,1,1,
1,1,1,1,1,1,1,6),(0.,0.0153846153846154,0.0307692307692308,0.0461538461538462,
0.0615384615384615,0.0769230769230769,0.0923076923076923,0.107692307692308,
0.123076923076923,0.138461538461538,0.153846153846154,0.169230769230769,
0.184615384615385,0.2,0.215384615384615,0.230769230769231,0.246153846153846,
0.261538461538462,0.276923076923077,0.292307692307692,0.307692307692308,
0.323076923076923,0.338461538461538,0.353846153846154,0.369230769230769,
0.384615384615385,0.4,0.415384615384615,0.430769230769231,0.446153846153846,
0.461538461538462,0.476923076923077,0.492307692307692,0.507692307692308,
0.523076923076923,0.538461538461538,0.553846153846154,0.569230769230769,
0.584615384615384,0.6,0.615384615384615,0.63076923076923,0.646153846153846,
0.661538461538461,0.676923076923076,0.692307692307692,0.707692307692307,
0.723076923076922,0.738461538461538,0.753846153846153,0.769230769230768,
0.784615384615384,0.799999999999999,0.815384615384614,0.83076923076923,
0.846153846153845,0.86153846153846,0.876923076923076,0.892307692307691,
0.907692307692306,0.923076923076922,0.938461538461537,0.953846153846152,
0.969230769230768,0.984615384615383,1.),.UNSPECIFIED.)
CURVE()
GEOMETRIC_REPRESENTATION_ITEM()
RATIONAL_B_SPLINE_CURVE((1.,1.,1.,1.,1.,1.,1.,1.,1.,1.,1.,1.,1.,1.,1.,1.,
1.,1.,1.,1.,1.,1.,1.,1.,1.,1.,1.,1.,1.,1.,1.,1.,1.,1.,1.,1.,1.,1.,1.,1.,
1.,1.,1.,1.,1.,1.,1.,1.,1.,1.,1.,1.,1.,1.,1.,1.,1.,1.,1.,1.,1.,1.,1.,1.,
1.,1.,1.,1.,1.,1.))
REPRESENTATION_ITEM('')
);
#82=(
BOUNDED_CURVE()
B_SPLINE_CURVE(5,(#23652,#23653,#23654,#23655,#23656,#23657,#23658,#23659,
#23660,#23661,#23662,#23663,#23664,#23665,#23666,#23667,#23668,#23669,#23670,
#23671,#23672,#23673,#23674,#23675,#23676,#23677,#23678,#23679,#23680,#23681,
#23682,#23683,#23684,#23685,#23686,#23687,#23688,#23689,#23690,#23691,#23692,
#23693,#23694,#23695,#23696,#23697,#23698,#23699,#23700,#23701,#23702,#23703,
#23704,#23705,#23706,#23707,#23708,#23709,#23710,#23711,#23712,#23713,#23714,
#23715,#23716,#23717,#23718,#23719,#23720,#23721),.UNSPECIFIED.,.F.,.F.)
B_SPLINE_CURVE_WITH_KNOTS((6,1,1,1,1,1,1,1,1,1,1,1,1,1,1,1,1,1,1,1,1,1,
1,1,1,1,1,1,1,1,1,1,1,1,1,1,1,1,1,1,1,1,1,1,1,1,1,1,1,1,1,1,1,1,1,1,1,1,
1,1,1,1,1,1,1,6),(0.,0.0153846153846154,0.0307692307692308,0.0461538461538462,
0.0615384615384615,0.0769230769230769,0.0923076923076923,0.107692307692308,
0.123076923076923,0.138461538461538,0.153846153846154,0.169230769230769,
0.184615384615385,0.2,0.215384615384615,0.230769230769231,0.246153846153846,
0.261538461538462,0.276923076923077,0.292307692307692,0.307692307692308,
0.323076923076923,0.338461538461538,0.353846153846154,0.369230769230769,
0.384615384615385,0.4,0.415384615384615,0.430769230769231,0.446153846153846,
0.461538461538462,0.476923076923077,0.492307692307692,0.507692307692308,
0.523076923076923,0.538461538461538,0.553846153846154,0.569230769230769,
0.584615384615384,0.6,0.615384615384615,0.63076923076923,0.646153846153846,
0.661538461538461,0.676923076923076,0.692307692307692,0.707692307692307,
0.723076923076922,0.738461538461538,0.753846153846153,0.769230769230768,
0.784615384615384,0.799999999999999,0.815384615384614,0.83076923076923,
0.846153846153845,0.86153846153846,0.876923076923076,0.892307692307691,
0.907692307692306,0.923076923076922,0.938461538461537,0.953846153846152,
0.969230769230768,0.984615384615383,1.),.UNSPECIFIED.)
CURVE()
GEOMETRIC_REPRESENTATION_ITEM()
RATIONAL_B_SPLINE_CURVE((1.,1.,1.,1.,1.,1.,1.,1.,1.,1.,1.,1.,1.,1.,1.,1.,
1.,1.,1.,1.,1.,1.,1.,1.,1.,1.,1.,1.,1.,1.,1.,1.,1.,1.,1.,1.,1.,1.,1.,1.,
1.,1.,1.,1.,1.,1.,1.,1.,1.,1.,1.,1.,1.,1.,1.,1.,1.,1.,1.,1.,1.,1.,1.,1.,
1.,1.,1.,1.,1.,1.))
REPRESENTATION_ITEM('')
);
#83=(
BOUNDED_CURVE()
B_SPLINE_CURVE(5,(#23725,#23726,#23727,#23728,#23729,#23730,#23731,#23732,
#23733,#23734,#23735,#23736,#23737,#23738,#23739,#23740,#23741,#23742,#23743,
#23744,#23745,#23746,#23747,#23748,#23749,#23750,#23751,#23752,#23753,#23754,
#23755,#23756,#23757,#23758,#23759,#23760,#23761,#23762,#23763,#23764,#23765,
#23766,#23767,#23768,#23769,#23770,#23771,#23772,#23773,#23774,#23775,#23776,
#23777,#23778,#23779,#23780,#23781,#23782,#23783,#23784,#23785,#23786,#23787,
#23788,#23789,#23790,#23791,#23792,#23793,#23794),.UNSPECIFIED.,.F.,.F.)
B_SPLINE_CURVE_WITH_KNOTS((6,1,1,1,1,1,1,1,1,1,1,1,1,1,1,1,1,1,1,1,1,1,
1,1,1,1,1,1,1,1,1,1,1,1,1,1,1,1,1,1,1,1,1,1,1,1,1,1,1,1,1,1,1,1,1,1,1,1,
1,1,1,1,1,1,1,6),(0.,0.0153846153846154,0.0307692307692308,0.0461538461538462,
0.0615384615384615,0.0769230769230769,0.0923076923076923,0.107692307692308,
0.123076923076923,0.138461538461538,0.153846153846154,0.169230769230769,
0.184615384615385,0.2,0.215384615384615,0.230769230769231,0.246153846153846,
0.261538461538462,0.276923076923077,0.292307692307692,0.307692307692308,
0.323076923076923,0.338461538461538,0.353846153846154,0.369230769230769,
0.384615384615385,0.4,0.415384615384615,0.430769230769231,0.446153846153846,
0.461538461538462,0.476923076923077,0.492307692307692,0.507692307692308,
0.523076923076923,0.538461538461538,0.553846153846154,0.569230769230769,
0.584615384615384,0.6,0.615384615384615,0.63076923076923,0.646153846153846,
0.661538461538461,0.676923076923076,0.692307692307692,0.707692307692307,
0.723076923076922,0.738461538461538,0.753846153846153,0.769230769230768,
0.784615384615384,0.799999999999999,0.815384615384614,0.83076923076923,
0.846153846153845,0.86153846153846,0.876923076923076,0.892307692307691,
0.907692307692306,0.923076923076922,0.938461538461537,0.953846153846152,
0.969230769230768,0.984615384615383,1.),.UNSPECIFIED.)
CURVE()
GEOMETRIC_REPRESENTATION_ITEM()
RATIONAL_B_SPLINE_CURVE((1.,1.,1.,1.,1.,1.,1.,1.,1.,1.,1.,1.,1.,1.,1.,1.,
1.,1.,1.,1.,1.,1.,1.,1.,1.,1.,1.,1.,1.,1.,1.,1.,1.,1.,1.,1.,1.,1.,1.,1.,
1.,1.,1.,1.,1.,1.,1.,1.,1.,1.,1.,1.,1.,1.,1.,1.,1.,1.,1.,1.,1.,1.,1.,1.,
1.,1.,1.,1.,1.,1.))
REPRESENTATION_ITEM('')
);
#84=(
BOUNDED_CURVE()
B_SPLINE_CURVE(5,(#23798,#23799,#23800,#23801,#23802,#23803,#23804,#23805,
#23806,#23807,#23808,#23809,#23810,#23811,#23812,#23813,#23814,#23815,#23816,
#23817,#23818,#23819,#23820,#23821,#23822,#23823,#23824,#23825,#23826,#23827,
#23828,#23829,#23830,#23831,#23832,#23833,#23834,#23835,#23836,#23837,#23838,
#23839,#23840,#23841,#23842,#23843,#23844,#23845,#23846,#23847,#23848,#23849,
#23850,#23851,#23852,#23853,#23854,#23855,#23856,#23857,#23858,#23859,#23860,
#23861,#23862,#23863,#23864,#23865,#23866,#23867),.UNSPECIFIED.,.F.,.F.)
B_SPLINE_CURVE_WITH_KNOTS((6,1,1,1,1,1,1,1,1,1,1,1,1,1,1,1,1,1,1,1,1,1,
1,1,1,1,1,1,1,1,1,1,1,1,1,1,1,1,1,1,1,1,1,1,1,1,1,1,1,1,1,1,1,1,1,1,1,1,
1,1,1,1,1,1,1,6),(0.,0.0153846153846154,0.0307692307692308,0.0461538461538462,
0.0615384615384615,0.0769230769230769,0.0923076923076923,0.107692307692308,
0.123076923076923,0.138461538461538,0.153846153846154,0.169230769230769,
0.184615384615385,0.2,0.215384615384615,0.230769230769231,0.246153846153846,
0.261538461538462,0.276923076923077,0.292307692307692,0.307692307692308,
0.323076923076923,0.338461538461538,0.353846153846154,0.369230769230769,
0.384615384615385,0.4,0.415384615384615,0.430769230769231,0.446153846153846,
0.461538461538462,0.476923076923077,0.492307692307692,0.507692307692308,
0.523076923076923,0.538461538461538,0.553846153846154,0.569230769230769,
0.584615384615384,0.6,0.615384615384615,0.63076923076923,0.646153846153846,
0.661538461538461,0.676923076923076,0.692307692307692,0.707692307692307,
0.723076923076922,0.738461538461538,0.753846153846153,0.769230769230768,
0.784615384615384,0.799999999999999,0.815384615384614,0.83076923076923,
0.846153846153845,0.86153846153846,0.876923076923076,0.892307692307691,
0.907692307692306,0.923076923076922,0.938461538461537,0.953846153846152,
0.969230769230768,0.984615384615383,1.),.UNSPECIFIED.)
CURVE()
GEOMETRIC_REPRESENTATION_ITEM()
RATIONAL_B_SPLINE_CURVE((1.,1.,1.,1.,1.,1.,1.,1.,1.,1.,1.,1.,1.,1.,1.,1.,
1.,1.,1.,1.,1.,1.,1.,1.,1.,1.,1.,1.,1.,1.,1.,1.,1.,1.,1.,1.,1.,1.,1.,1.,
1.,1.,1.,1.,1.,1.,1.,1.,1.,1.,1.,1.,1.,1.,1.,1.,1.,1.,1.,1.,1.,1.,1.,1.,
1.,1.,1.,1.,1.,1.))
REPRESENTATION_ITEM('')
);
#85=(
BOUNDED_CURVE()
B_SPLINE_CURVE(5,(#23871,#23872,#23873,#23874,#23875,#23876,#23877,#23878,
#23879,#23880,#23881,#23882,#23883,#23884,#23885,#23886,#23887,#23888,#23889,
#23890,#23891,#23892,#23893,#23894,#23895,#23896,#23897,#23898,#23899,#23900,
#23901,#23902,#23903,#23904,#23905,#23906,#23907,#23908,#23909,#23910,#23911,
#23912,#23913,#23914,#23915,#23916,#23917,#23918,#23919,#23920,#23921,#23922,
#23923,#23924,#23925,#23926,#23927,#23928,#23929,#23930,#23931,#23932,#23933,
#23934,#23935,#23936,#23937,#23938,#23939,#23940),.UNSPECIFIED.,.F.,.F.)
B_SPLINE_CURVE_WITH_KNOTS((6,1,1,1,1,1,1,1,1,1,1,1,1,1,1,1,1,1,1,1,1,1,
1,1,1,1,1,1,1,1,1,1,1,1,1,1,1,1,1,1,1,1,1,1,1,1,1,1,1,1,1,1,1,1,1,1,1,1,
1,1,1,1,1,1,1,6),(0.,0.0153846153846154,0.0307692307692308,0.0461538461538462,
0.0615384615384615,0.0769230769230769,0.0923076923076923,0.107692307692308,
0.123076923076923,0.138461538461538,0.153846153846154,0.169230769230769,
0.184615384615385,0.2,0.215384615384615,0.230769230769231,0.246153846153846,
0.261538461538462,0.276923076923077,0.292307692307692,0.307692307692308,
0.323076923076923,0.338461538461538,0.353846153846154,0.369230769230769,
0.384615384615385,0.4,0.415384615384615,0.430769230769231,0.446153846153846,
0.461538461538462,0.476923076923077,0.492307692307692,0.507692307692308,
0.523076923076923,0.538461538461538,0.553846153846154,0.569230769230769,
0.584615384615384,0.6,0.615384615384615,0.63076923076923,0.646153846153846,
0.661538461538461,0.676923076923076,0.692307692307692,0.707692307692307,
0.723076923076922,0.738461538461538,0.753846153846153,0.769230769230768,
0.784615384615384,0.799999999999999,0.815384615384614,0.83076923076923,
0.846153846153845,0.86153846153846,0.876923076923076,0.892307692307691,
0.907692307692306,0.923076923076922,0.938461538461537,0.953846153846152,
0.969230769230768,0.984615384615383,1.),.UNSPECIFIED.)
CURVE()
GEOMETRIC_REPRESENTATION_ITEM()
RATIONAL_B_SPLINE_CURVE((1.,1.,1.,1.,1.,1.,1.,1.,1.,1.,1.,1.,1.,1.,1.,1.,
1.,1.,1.,1.,1.,1.,1.,1.,1.,1.,1.,1.,1.,1.,1.,1.,1.,1.,1.,1.,1.,1.,1.,1.,
1.,1.,1.,1.,1.,1.,1.,1.,1.,1.,1.,1.,1.,1.,1.,1.,1.,1.,1.,1.,1.,1.,1.,1.,
1.,1.,1.,1.,1.,1.))
REPRESENTATION_ITEM('')
);
#86=(
BOUNDED_CURVE()
B_SPLINE_CURVE(5,(#23944,#23945,#23946,#23947,#23948,#23949,#23950,#23951,
#23952,#23953,#23954,#23955,#23956,#23957,#23958,#23959,#23960,#23961,#23962,
#23963,#23964,#23965,#23966,#23967,#23968,#23969,#23970,#23971,#23972,#23973,
#23974,#23975,#23976,#23977,#23978,#23979,#23980,#23981,#23982,#23983,#23984,
#23985,#23986,#23987,#23988,#23989,#23990,#23991,#23992,#23993,#23994,#23995,
#23996,#23997,#23998,#23999,#24000,#24001,#24002,#24003,#24004,#24005,#24006,
#24007,#24008,#24009,#24010,#24011,#24012,#24013),.UNSPECIFIED.,.F.,.F.)
B_SPLINE_CURVE_WITH_KNOTS((6,1,1,1,1,1,1,1,1,1,1,1,1,1,1,1,1,1,1,1,1,1,
1,1,1,1,1,1,1,1,1,1,1,1,1,1,1,1,1,1,1,1,1,1,1,1,1,1,1,1,1,1,1,1,1,1,1,1,
1,1,1,1,1,1,1,6),(0.,0.0153846153846154,0.0307692307692308,0.0461538461538462,
0.0615384615384615,0.0769230769230769,0.0923076923076923,0.107692307692308,
0.123076923076923,0.138461538461538,0.153846153846154,0.169230769230769,
0.184615384615385,0.2,0.215384615384615,0.230769230769231,0.246153846153846,
0.261538461538462,0.276923076923077,0.292307692307692,0.307692307692308,
0.323076923076923,0.338461538461538,0.353846153846154,0.369230769230769,
0.384615384615385,0.4,0.415384615384615,0.430769230769231,0.446153846153846,
0.461538461538462,0.476923076923077,0.492307692307692,0.507692307692308,
0.523076923076923,0.538461538461538,0.553846153846154,0.569230769230769,
0.584615384615384,0.6,0.615384615384615,0.63076923076923,0.646153846153846,
0.661538461538461,0.676923076923076,0.692307692307692,0.707692307692307,
0.723076923076922,0.738461538461538,0.753846153846153,0.769230769230768,
0.784615384615384,0.799999999999999,0.815384615384614,0.83076923076923,
0.846153846153845,0.86153846153846,0.876923076923076,0.892307692307691,
0.907692307692306,0.923076923076922,0.938461538461537,0.953846153846152,
0.969230769230768,0.984615384615383,1.),.UNSPECIFIED.)
CURVE()
GEOMETRIC_REPRESENTATION_ITEM()
RATIONAL_B_SPLINE_CURVE((1.,1.,1.,1.,1.,1.,1.,1.,1.,1.,1.,1.,1.,1.,1.,1.,
1.,1.,1.,1.,1.,1.,1.,1.,1.,1.,1.,1.,1.,1.,1.,1.,1.,1.,1.,1.,1.,1.,1.,1.,
1.,1.,1.,1.,1.,1.,1.,1.,1.,1.,1.,1.,1.,1.,1.,1.,1.,1.,1.,1.,1.,1.,1.,1.,
1.,1.,1.,1.,1.,1.))
REPRESENTATION_ITEM('')
);
#87=(
BOUNDED_CURVE()
B_SPLINE_CURVE(5,(#24017,#24018,#24019,#24020,#24021,#24022,#24023,#24024,
#24025,#24026,#24027,#24028,#24029,#24030,#24031,#24032,#24033,#24034,#24035,
#24036,#24037,#24038,#24039,#24040,#24041,#24042,#24043,#24044,#24045,#24046,
#24047,#24048,#24049,#24050,#24051,#24052,#24053,#24054,#24055,#24056,#24057,
#24058,#24059,#24060,#24061,#24062,#24063,#24064,#24065,#24066,#24067,#24068,
#24069,#24070,#24071,#24072,#24073,#24074,#24075,#24076,#24077,#24078,#24079,
#24080,#24081,#24082,#24083,#24084,#24085,#24086),.UNSPECIFIED.,.F.,.F.)
B_SPLINE_CURVE_WITH_KNOTS((6,1,1,1,1,1,1,1,1,1,1,1,1,1,1,1,1,1,1,1,1,1,
1,1,1,1,1,1,1,1,1,1,1,1,1,1,1,1,1,1,1,1,1,1,1,1,1,1,1,1,1,1,1,1,1,1,1,1,
1,1,1,1,1,1,1,6),(0.,0.0153846153846154,0.0307692307692308,0.0461538461538462,
0.0615384615384615,0.0769230769230769,0.0923076923076923,0.107692307692308,
0.123076923076923,0.138461538461538,0.153846153846154,0.169230769230769,
0.184615384615385,0.2,0.215384615384615,0.230769230769231,0.246153846153846,
0.261538461538462,0.276923076923077,0.292307692307692,0.307692307692308,
0.323076923076923,0.338461538461538,0.353846153846154,0.369230769230769,
0.384615384615385,0.4,0.415384615384615,0.430769230769231,0.446153846153846,
0.461538461538462,0.476923076923077,0.492307692307692,0.507692307692308,
0.523076923076923,0.538461538461538,0.553846153846154,0.569230769230769,
0.584615384615384,0.6,0.615384615384615,0.63076923076923,0.646153846153846,
0.661538461538461,0.676923076923076,0.692307692307692,0.707692307692307,
0.723076923076922,0.738461538461538,0.753846153846153,0.769230769230768,
0.784615384615384,0.799999999999999,0.815384615384614,0.83076923076923,
0.846153846153845,0.86153846153846,0.876923076923076,0.892307692307691,
0.907692307692306,0.923076923076922,0.938461538461537,0.953846153846152,
0.969230769230768,0.984615384615383,1.),.UNSPECIFIED.)
CURVE()
GEOMETRIC_REPRESENTATION_ITEM()
RATIONAL_B_SPLINE_CURVE((1.,1.,1.,1.,1.,1.,1.,1.,1.,1.,1.,1.,1.,1.,1.,1.,
1.,1.,1.,1.,1.,1.,1.,1.,1.,1.,1.,1.,1.,1.,1.,1.,1.,1.,1.,1.,1.,1.,1.,1.,
1.,1.,1.,1.,1.,1.,1.,1.,1.,1.,1.,1.,1.,1.,1.,1.,1.,1.,1.,1.,1.,1.,1.,1.,
1.,1.,1.,1.,1.,1.))
REPRESENTATION_ITEM('')
);
#88=(
BOUNDED_CURVE()
B_SPLINE_CURVE(5,(#24090,#24091,#24092,#24093,#24094,#24095,#24096,#24097,
#24098,#24099,#24100,#24101,#24102,#24103,#24104,#24105,#24106,#24107,#24108,
#24109,#24110,#24111,#24112,#24113,#24114,#24115,#24116,#24117,#24118,#24119,
#24120,#24121,#24122,#24123,#24124,#24125,#24126,#24127,#24128,#24129,#24130,
#24131,#24132,#24133,#24134,#24135,#24136,#24137,#24138,#24139,#24140,#24141,
#24142,#24143,#24144,#24145,#24146,#24147,#24148,#24149,#24150,#24151,#24152,
#24153,#24154,#24155,#24156,#24157,#24158,#24159),.UNSPECIFIED.,.F.,.F.)
B_SPLINE_CURVE_WITH_KNOTS((6,1,1,1,1,1,1,1,1,1,1,1,1,1,1,1,1,1,1,1,1,1,
1,1,1,1,1,1,1,1,1,1,1,1,1,1,1,1,1,1,1,1,1,1,1,1,1,1,1,1,1,1,1,1,1,1,1,1,
1,1,1,1,1,1,1,6),(0.,0.0153846153846154,0.0307692307692308,0.0461538461538462,
0.0615384615384615,0.0769230769230769,0.0923076923076923,0.107692307692308,
0.123076923076923,0.138461538461538,0.153846153846154,0.169230769230769,
0.184615384615385,0.2,0.215384615384615,0.230769230769231,0.246153846153846,
0.261538461538462,0.276923076923077,0.292307692307692,0.307692307692308,
0.323076923076923,0.338461538461538,0.353846153846154,0.369230769230769,
0.384615384615385,0.4,0.415384615384615,0.430769230769231,0.446153846153846,
0.461538461538462,0.476923076923077,0.492307692307692,0.507692307692308,
0.523076923076923,0.538461538461538,0.553846153846154,0.569230769230769,
0.584615384615384,0.6,0.615384615384615,0.63076923076923,0.646153846153846,
0.661538461538461,0.676923076923076,0.692307692307692,0.707692307692307,
0.723076923076922,0.738461538461538,0.753846153846153,0.769230769230768,
0.784615384615384,0.799999999999999,0.815384615384614,0.83076923076923,
0.846153846153845,0.86153846153846,0.876923076923076,0.892307692307691,
0.907692307692306,0.923076923076922,0.938461538461537,0.953846153846152,
0.969230769230768,0.984615384615383,1.),.UNSPECIFIED.)
CURVE()
GEOMETRIC_REPRESENTATION_ITEM()
RATIONAL_B_SPLINE_CURVE((1.,1.,1.,1.,1.,1.,1.,1.,1.,1.,1.,1.,1.,1.,1.,1.,
1.,1.,1.,1.,1.,1.,1.,1.,1.,1.,1.,1.,1.,1.,1.,1.,1.,1.,1.,1.,1.,1.,1.,1.,
1.,1.,1.,1.,1.,1.,1.,1.,1.,1.,1.,1.,1.,1.,1.,1.,1.,1.,1.,1.,1.,1.,1.,1.,
1.,1.,1.,1.,1.,1.))
REPRESENTATION_ITEM('')
);
#89=(
BOUNDED_CURVE()
B_SPLINE_CURVE(5,(#24163,#24164,#24165,#24166,#24167,#24168,#24169,#24170,
#24171,#24172,#24173,#24174,#24175,#24176,#24177,#24178,#24179,#24180,#24181,
#24182,#24183,#24184,#24185,#24186,#24187,#24188,#24189,#24190,#24191,#24192,
#24193,#24194,#24195,#24196,#24197,#24198,#24199,#24200,#24201,#24202,#24203,
#24204,#24205,#24206,#24207,#24208,#24209,#24210,#24211,#24212,#24213,#24214,
#24215,#24216,#24217,#24218,#24219,#24220,#24221,#24222,#24223,#24224,#24225,
#24226,#24227,#24228,#24229,#24230,#24231,#24232),.UNSPECIFIED.,.F.,.F.)
B_SPLINE_CURVE_WITH_KNOTS((6,1,1,1,1,1,1,1,1,1,1,1,1,1,1,1,1,1,1,1,1,1,
1,1,1,1,1,1,1,1,1,1,1,1,1,1,1,1,1,1,1,1,1,1,1,1,1,1,1,1,1,1,1,1,1,1,1,1,
1,1,1,1,1,1,1,6),(0.,0.0153846153846154,0.0307692307692308,0.0461538461538462,
0.0615384615384615,0.0769230769230769,0.0923076923076923,0.107692307692308,
0.123076923076923,0.138461538461538,0.153846153846154,0.169230769230769,
0.184615384615385,0.2,0.215384615384615,0.230769230769231,0.246153846153846,
0.261538461538462,0.276923076923077,0.292307692307692,0.307692307692308,
0.323076923076923,0.338461538461538,0.353846153846154,0.369230769230769,
0.384615384615385,0.4,0.415384615384615,0.430769230769231,0.446153846153846,
0.461538461538462,0.476923076923077,0.492307692307692,0.507692307692308,
0.523076923076923,0.538461538461538,0.553846153846154,0.569230769230769,
0.584615384615384,0.6,0.615384615384615,0.63076923076923,0.646153846153846,
0.661538461538461,0.676923076923076,0.692307692307692,0.707692307692307,
0.723076923076922,0.738461538461538,0.753846153846153,0.769230769230768,
0.784615384615384,0.799999999999999,0.815384615384614,0.83076923076923,
0.846153846153845,0.86153846153846,0.876923076923076,0.892307692307691,
0.907692307692306,0.923076923076922,0.938461538461537,0.953846153846152,
0.969230769230768,0.984615384615383,1.),.UNSPECIFIED.)
CURVE()
GEOMETRIC_REPRESENTATION_ITEM()
RATIONAL_B_SPLINE_CURVE((1.,1.,1.,1.,1.,1.,1.,1.,1.,1.,1.,1.,1.,1.,1.,1.,
1.,1.,1.,1.,1.,1.,1.,1.,1.,1.,1.,1.,1.,1.,1.,1.,1.,1.,1.,1.,1.,1.,1.,1.,
1.,1.,1.,1.,1.,1.,1.,1.,1.,1.,1.,1.,1.,1.,1.,1.,1.,1.,1.,1.,1.,1.,1.,1.,
1.,1.,1.,1.,1.,1.))
REPRESENTATION_ITEM('')
);
#90=(
BOUNDED_CURVE()
B_SPLINE_CURVE(5,(#24235,#24236,#24237,#24238,#24239,#24240,#24241,#24242,
#24243,#24244,#24245,#24246,#24247,#24248,#24249,#24250,#24251,#24252,#24253,
#24254,#24255,#24256,#24257,#24258,#24259,#24260,#24261,#24262,#24263,#24264,
#24265,#24266,#24267,#24268,#24269,#24270,#24271,#24272,#24273,#24274,#24275,
#24276,#24277,#24278,#24279,#24280,#24281,#24282,#24283,#24284,#24285,#24286,
#24287,#24288,#24289,#24290,#24291,#24292,#24293,#24294,#24295,#24296,#24297,
#24298,#24299,#24300,#24301,#24302,#24303,#24304),.UNSPECIFIED.,.F.,.F.)
B_SPLINE_CURVE_WITH_KNOTS((6,1,1,1,1,1,1,1,1,1,1,1,1,1,1,1,1,1,1,1,1,1,
1,1,1,1,1,1,1,1,1,1,1,1,1,1,1,1,1,1,1,1,1,1,1,1,1,1,1,1,1,1,1,1,1,1,1,1,
1,1,1,1,1,1,1,6),(0.,0.0153846153846154,0.0307692307692308,0.0461538461538462,
0.0615384615384615,0.0769230769230769,0.0923076923076923,0.107692307692308,
0.123076923076923,0.138461538461538,0.153846153846154,0.169230769230769,
0.184615384615385,0.2,0.215384615384615,0.230769230769231,0.246153846153846,
0.261538461538462,0.276923076923077,0.292307692307692,0.307692307692308,
0.323076923076923,0.338461538461538,0.353846153846154,0.369230769230769,
0.384615384615385,0.4,0.415384615384615,0.430769230769231,0.446153846153846,
0.461538461538462,0.476923076923077,0.492307692307692,0.507692307692308,
0.523076923076923,0.538461538461538,0.553846153846154,0.569230769230769,
0.584615384615384,0.6,0.615384615384615,0.63076923076923,0.646153846153846,
0.661538461538461,0.676923076923076,0.692307692307692,0.707692307692307,
0.723076923076922,0.738461538461538,0.753846153846153,0.769230769230768,
0.784615384615384,0.799999999999999,0.815384615384614,0.83076923076923,
0.846153846153845,0.86153846153846,0.876923076923076,0.892307692307691,
0.907692307692306,0.923076923076922,0.938461538461537,0.953846153846152,
0.969230769230768,0.984615384615383,1.),.UNSPECIFIED.)
CURVE()
GEOMETRIC_REPRESENTATION_ITEM()
RATIONAL_B_SPLINE_CURVE((1.,1.,1.,1.,1.,1.,1.,1.,1.,1.,1.,1.,1.,1.,1.,1.,
1.,1.,1.,1.,1.,1.,1.,1.,1.,1.,1.,1.,1.,1.,1.,1.,1.,1.,1.,1.,1.,1.,1.,1.,
1.,1.,1.,1.,1.,1.,1.,1.,1.,1.,1.,1.,1.,1.,1.,1.,1.,1.,1.,1.,1.,1.,1.,1.,
1.,1.,1.,1.,1.,1.))
REPRESENTATION_ITEM('')
);
#91=(
BOUNDED_CURVE()
B_SPLINE_CURVE(5,(#24458,#24459,#24460,#24461,#24462,#24463,#24464,#24465,
#24466,#24467,#24468,#24469,#24470,#24471,#24472,#24473,#24474,#24475,#24476,
#24477,#24478,#24479,#24480,#24481,#24482,#24483,#24484,#24485,#24486,#24487,
#24488,#24489,#24490,#24491,#24492,#24493,#24494,#24495,#24496,#24497,#24498,
#24499,#24500,#24501,#24502,#24503,#24504,#24505,#24506,#24507,#24508,#24509,
#24510,#24511,#24512,#24513,#24514,#24515,#24516,#24517,#24518,#24519,#24520,
#24521,#24522,#24523,#24524,#24525,#24526,#24527),.UNSPECIFIED.,.F.,.F.)
B_SPLINE_CURVE_WITH_KNOTS((6,1,1,1,1,1,1,1,1,1,1,1,1,1,1,1,1,1,1,1,1,1,
1,1,1,1,1,1,1,1,1,1,1,1,1,1,1,1,1,1,1,1,1,1,1,1,1,1,1,1,1,1,1,1,1,1,1,1,
1,1,1,1,1,1,1,6),(-1.,-0.984615384615383,-0.969230769230768,-0.953846153846152,
-0.938461538461537,-0.923076923076922,-0.907692307692306,-0.892307692307691,
-0.876923076923076,-0.86153846153846,-0.846153846153845,-0.83076923076923,
-0.815384615384614,-0.799999999999999,-0.784615384615384,-0.769230769230768,
-0.753846153846153,-0.738461538461538,-0.723076923076922,-0.707692307692307,
-0.692307692307692,-0.676923076923076,-0.661538461538461,-0.646153846153846,
-0.63076923076923,-0.615384615384615,-0.6,-0.584615384615384,-0.569230769230769,
-0.553846153846154,-0.538461538461538,-0.523076923076923,-0.507692307692308,
-0.492307692307692,-0.476923076923077,-0.461538461538462,-0.446153846153846,
-0.430769230769231,-0.415384615384615,-0.4,-0.384615384615385,-0.369230769230769,
-0.353846153846154,-0.338461538461538,-0.323076923076923,-0.307692307692308,
-0.292307692307692,-0.276923076923077,-0.261538461538462,-0.246153846153846,
-0.230769230769231,-0.215384615384615,-0.2,-0.184615384615385,-0.169230769230769,
-0.153846153846154,-0.138461538461538,-0.123076923076923,-0.107692307692308,
-0.0923076923076923,-0.0769230769230769,-0.0615384615384615,-0.0461538461538462,
-0.0307692307692308,-0.0153846153846154,0.),.UNSPECIFIED.)
CURVE()
GEOMETRIC_REPRESENTATION_ITEM()
RATIONAL_B_SPLINE_CURVE((1.,1.,1.,1.,1.,1.,1.,1.,1.,1.,1.,1.,1.,1.,1.,1.,
1.,1.,1.,1.,1.,1.,1.,1.,1.,1.,1.,1.,1.,1.,1.,1.,1.,1.,1.,1.,1.,1.,1.,1.,
1.,1.,1.,1.,1.,1.,1.,1.,1.,1.,1.,1.,1.,1.,1.,1.,1.,1.,1.,1.,1.,1.,1.,1.,
1.,1.,1.,1.,1.,1.))
REPRESENTATION_ITEM('')
);
#92=(
BOUNDED_CURVE()
B_SPLINE_CURVE(5,(#24674,#24675,#24676,#24677,#24678,#24679,#24680,#24681,
#24682,#24683,#24684,#24685,#24686,#24687,#24688,#24689,#24690,#24691,#24692,
#24693,#24694,#24695,#24696,#24697,#24698,#24699,#24700,#24701,#24702,#24703,
#24704,#24705,#24706,#24707,#24708,#24709,#24710,#24711,#24712,#24713,#24714,
#24715,#24716,#24717,#24718,#24719,#24720,#24721,#24722,#24723,#24724,#24725,
#24726,#24727,#24728,#24729,#24730,#24731,#24732,#24733,#24734,#24735,#24736,
#24737,#24738,#24739,#24740,#24741,#24742,#24743),.UNSPECIFIED.,.F.,.F.)
B_SPLINE_CURVE_WITH_KNOTS((6,1,1,1,1,1,1,1,1,1,1,1,1,1,1,1,1,1,1,1,1,1,
1,1,1,1,1,1,1,1,1,1,1,1,1,1,1,1,1,1,1,1,1,1,1,1,1,1,1,1,1,1,1,1,1,1,1,1,
1,1,1,1,1,1,1,6),(-1.,-0.984615384615383,-0.969230769230768,-0.953846153846152,
-0.938461538461537,-0.923076923076922,-0.907692307692306,-0.892307692307691,
-0.876923076923076,-0.86153846153846,-0.846153846153845,-0.83076923076923,
-0.815384615384614,-0.799999999999999,-0.784615384615384,-0.769230769230768,
-0.753846153846153,-0.738461538461538,-0.723076923076922,-0.707692307692307,
-0.692307692307692,-0.676923076923076,-0.661538461538461,-0.646153846153846,
-0.63076923076923,-0.615384615384615,-0.6,-0.584615384615384,-0.569230769230769,
-0.553846153846154,-0.538461538461538,-0.523076923076923,-0.507692307692308,
-0.492307692307692,-0.476923076923077,-0.461538461538462,-0.446153846153846,
-0.430769230769231,-0.415384615384615,-0.4,-0.384615384615385,-0.369230769230769,
-0.353846153846154,-0.338461538461538,-0.323076923076923,-0.307692307692308,
-0.292307692307692,-0.276923076923077,-0.261538461538462,-0.246153846153846,
-0.230769230769231,-0.215384615384615,-0.2,-0.184615384615385,-0.169230769230769,
-0.153846153846154,-0.138461538461538,-0.123076923076923,-0.107692307692308,
-0.0923076923076923,-0.0769230769230769,-0.0615384615384615,-0.0461538461538462,
-0.0307692307692308,-0.0153846153846154,0.),.UNSPECIFIED.)
CURVE()
GEOMETRIC_REPRESENTATION_ITEM()
RATIONAL_B_SPLINE_CURVE((1.,1.,1.,1.,1.,1.,1.,1.,1.,1.,1.,1.,1.,1.,1.,1.,
1.,1.,1.,1.,1.,1.,1.,1.,1.,1.,1.,1.,1.,1.,1.,1.,1.,1.,1.,1.,1.,1.,1.,1.,
1.,1.,1.,1.,1.,1.,1.,1.,1.,1.,1.,1.,1.,1.,1.,1.,1.,1.,1.,1.,1.,1.,1.,1.,
1.,1.,1.,1.,1.,1.))
REPRESENTATION_ITEM('')
);
#93=(
BOUNDED_CURVE()
B_SPLINE_CURVE(5,(#24890,#24891,#24892,#24893,#24894,#24895,#24896,#24897,
#24898,#24899,#24900,#24901,#24902,#24903,#24904,#24905,#24906,#24907,#24908,
#24909,#24910,#24911,#24912,#24913,#24914,#24915,#24916,#24917,#24918,#24919,
#24920,#24921,#24922,#24923,#24924,#24925,#24926,#24927,#24928,#24929,#24930,
#24931,#24932,#24933,#24934,#24935,#24936,#24937,#24938,#24939,#24940,#24941,
#24942,#24943,#24944,#24945,#24946,#24947,#24948,#24949,#24950,#24951,#24952,
#24953,#24954,#24955,#24956,#24957,#24958,#24959),.UNSPECIFIED.,.F.,.F.)
B_SPLINE_CURVE_WITH_KNOTS((6,1,1,1,1,1,1,1,1,1,1,1,1,1,1,1,1,1,1,1,1,1,
1,1,1,1,1,1,1,1,1,1,1,1,1,1,1,1,1,1,1,1,1,1,1,1,1,1,1,1,1,1,1,1,1,1,1,1,
1,1,1,1,1,1,1,6),(-1.,-0.984615384615383,-0.969230769230768,-0.953846153846152,
-0.938461538461537,-0.923076923076922,-0.907692307692306,-0.892307692307691,
-0.876923076923076,-0.86153846153846,-0.846153846153845,-0.83076923076923,
-0.815384615384614,-0.799999999999999,-0.784615384615384,-0.769230769230768,
-0.753846153846153,-0.738461538461538,-0.723076923076922,-0.707692307692307,
-0.692307692307692,-0.676923076923076,-0.661538461538461,-0.646153846153846,
-0.63076923076923,-0.615384615384615,-0.6,-0.584615384615384,-0.569230769230769,
-0.553846153846154,-0.538461538461538,-0.523076923076923,-0.507692307692308,
-0.492307692307692,-0.476923076923077,-0.461538461538462,-0.446153846153846,
-0.430769230769231,-0.415384615384615,-0.4,-0.384615384615385,-0.369230769230769,
-0.353846153846154,-0.338461538461538,-0.323076923076923,-0.307692307692308,
-0.292307692307692,-0.276923076923077,-0.261538461538462,-0.246153846153846,
-0.230769230769231,-0.215384615384615,-0.2,-0.184615384615385,-0.169230769230769,
-0.153846153846154,-0.138461538461538,-0.123076923076923,-0.107692307692308,
-0.0923076923076923,-0.0769230769230769,-0.0615384615384615,-0.0461538461538462,
-0.0307692307692308,-0.0153846153846154,0.),.UNSPECIFIED.)
CURVE()
GEOMETRIC_REPRESENTATION_ITEM()
RATIONAL_B_SPLINE_CURVE((1.,1.,1.,1.,1.,1.,1.,1.,1.,1.,1.,1.,1.,1.,1.,1.,
1.,1.,1.,1.,1.,1.,1.,1.,1.,1.,1.,1.,1.,1.,1.,1.,1.,1.,1.,1.,1.,1.,1.,1.,
1.,1.,1.,1.,1.,1.,1.,1.,1.,1.,1.,1.,1.,1.,1.,1.,1.,1.,1.,1.,1.,1.,1.,1.,
1.,1.,1.,1.,1.,1.))
REPRESENTATION_ITEM('')
);
#94=(
BOUNDED_CURVE()
B_SPLINE_CURVE(5,(#25106,#25107,#25108,#25109,#25110,#25111,#25112,#25113,
#25114,#25115,#25116,#25117,#25118,#25119,#25120,#25121,#25122,#25123,#25124,
#25125,#25126,#25127,#25128,#25129,#25130,#25131,#25132,#25133,#25134,#25135,
#25136,#25137,#25138,#25139,#25140,#25141,#25142,#25143,#25144,#25145,#25146,
#25147,#25148,#25149,#25150,#25151,#25152,#25153,#25154,#25155,#25156,#25157,
#25158,#25159,#25160,#25161,#25162,#25163,#25164,#25165,#25166,#25167,#25168,
#25169,#25170,#25171,#25172,#25173,#25174,#25175),.UNSPECIFIED.,.F.,.F.)
B_SPLINE_CURVE_WITH_KNOTS((6,1,1,1,1,1,1,1,1,1,1,1,1,1,1,1,1,1,1,1,1,1,
1,1,1,1,1,1,1,1,1,1,1,1,1,1,1,1,1,1,1,1,1,1,1,1,1,1,1,1,1,1,1,1,1,1,1,1,
1,1,1,1,1,1,1,6),(-1.,-0.984615384615383,-0.969230769230768,-0.953846153846152,
-0.938461538461537,-0.923076923076922,-0.907692307692306,-0.892307692307691,
-0.876923076923076,-0.86153846153846,-0.846153846153845,-0.83076923076923,
-0.815384615384614,-0.799999999999999,-0.784615384615384,-0.769230769230768,
-0.753846153846153,-0.738461538461538,-0.723076923076922,-0.707692307692307,
-0.692307692307692,-0.676923076923076,-0.661538461538461,-0.646153846153846,
-0.63076923076923,-0.615384615384615,-0.6,-0.584615384615384,-0.569230769230769,
-0.553846153846154,-0.538461538461538,-0.523076923076923,-0.507692307692308,
-0.492307692307692,-0.476923076923077,-0.461538461538462,-0.446153846153846,
-0.430769230769231,-0.415384615384615,-0.4,-0.384615384615385,-0.369230769230769,
-0.353846153846154,-0.338461538461538,-0.323076923076923,-0.307692307692308,
-0.292307692307692,-0.276923076923077,-0.261538461538462,-0.246153846153846,
-0.230769230769231,-0.215384615384615,-0.2,-0.184615384615385,-0.169230769230769,
-0.153846153846154,-0.138461538461538,-0.123076923076923,-0.107692307692308,
-0.0923076923076923,-0.0769230769230769,-0.0615384615384615,-0.0461538461538462,
-0.0307692307692308,-0.0153846153846154,0.),.UNSPECIFIED.)
CURVE()
GEOMETRIC_REPRESENTATION_ITEM()
RATIONAL_B_SPLINE_CURVE((1.,1.,1.,1.,1.,1.,1.,1.,1.,1.,1.,1.,1.,1.,1.,1.,
1.,1.,1.,1.,1.,1.,1.,1.,1.,1.,1.,1.,1.,1.,1.,1.,1.,1.,1.,1.,1.,1.,1.,1.,
1.,1.,1.,1.,1.,1.,1.,1.,1.,1.,1.,1.,1.,1.,1.,1.,1.,1.,1.,1.,1.,1.,1.,1.,
1.,1.,1.,1.,1.,1.))
REPRESENTATION_ITEM('')
);
#95=(
BOUNDED_CURVE()
B_SPLINE_CURVE(5,(#25322,#25323,#25324,#25325,#25326,#25327,#25328,#25329,
#25330,#25331,#25332,#25333,#25334,#25335,#25336,#25337,#25338,#25339,#25340,
#25341,#25342,#25343,#25344,#25345,#25346,#25347,#25348,#25349,#25350,#25351,
#25352,#25353,#25354,#25355,#25356,#25357,#25358,#25359,#25360,#25361,#25362,
#25363,#25364,#25365,#25366,#25367,#25368,#25369,#25370,#25371,#25372,#25373,
#25374,#25375,#25376,#25377,#25378,#25379,#25380,#25381,#25382,#25383,#25384,
#25385,#25386,#25387,#25388,#25389,#25390,#25391),.UNSPECIFIED.,.F.,.F.)
B_SPLINE_CURVE_WITH_KNOTS((6,1,1,1,1,1,1,1,1,1,1,1,1,1,1,1,1,1,1,1,1,1,
1,1,1,1,1,1,1,1,1,1,1,1,1,1,1,1,1,1,1,1,1,1,1,1,1,1,1,1,1,1,1,1,1,1,1,1,
1,1,1,1,1,1,1,6),(-1.,-0.984615384615383,-0.969230769230768,-0.953846153846152,
-0.938461538461537,-0.923076923076922,-0.907692307692306,-0.892307692307691,
-0.876923076923076,-0.86153846153846,-0.846153846153845,-0.83076923076923,
-0.815384615384614,-0.799999999999999,-0.784615384615384,-0.769230769230768,
-0.753846153846153,-0.738461538461538,-0.723076923076922,-0.707692307692307,
-0.692307692307692,-0.676923076923076,-0.661538461538461,-0.646153846153846,
-0.63076923076923,-0.615384615384615,-0.6,-0.584615384615384,-0.569230769230769,
-0.553846153846154,-0.538461538461538,-0.523076923076923,-0.507692307692308,
-0.492307692307692,-0.476923076923077,-0.461538461538462,-0.446153846153846,
-0.430769230769231,-0.415384615384615,-0.4,-0.384615384615385,-0.369230769230769,
-0.353846153846154,-0.338461538461538,-0.323076923076923,-0.307692307692308,
-0.292307692307692,-0.276923076923077,-0.261538461538462,-0.246153846153846,
-0.230769230769231,-0.215384615384615,-0.2,-0.184615384615385,-0.169230769230769,
-0.153846153846154,-0.138461538461538,-0.123076923076923,-0.107692307692308,
-0.0923076923076923,-0.0769230769230769,-0.0615384615384615,-0.0461538461538462,
-0.0307692307692308,-0.0153846153846154,0.),.UNSPECIFIED.)
CURVE()
GEOMETRIC_REPRESENTATION_ITEM()
RATIONAL_B_SPLINE_CURVE((1.,1.,1.,1.,1.,1.,1.,1.,1.,1.,1.,1.,1.,1.,1.,1.,
1.,1.,1.,1.,1.,1.,1.,1.,1.,1.,1.,1.,1.,1.,1.,1.,1.,1.,1.,1.,1.,1.,1.,1.,
1.,1.,1.,1.,1.,1.,1.,1.,1.,1.,1.,1.,1.,1.,1.,1.,1.,1.,1.,1.,1.,1.,1.,1.,
1.,1.,1.,1.,1.,1.))
REPRESENTATION_ITEM('')
);
#96=(
BOUNDED_CURVE()
B_SPLINE_CURVE(5,(#25538,#25539,#25540,#25541,#25542,#25543,#25544,#25545,
#25546,#25547,#25548,#25549,#25550,#25551,#25552,#25553,#25554,#25555,#25556,
#25557,#25558,#25559,#25560,#25561,#25562,#25563,#25564,#25565,#25566,#25567,
#25568,#25569,#25570,#25571,#25572,#25573,#25574,#25575,#25576,#25577,#25578,
#25579,#25580,#25581,#25582,#25583,#25584,#25585,#25586,#25587,#25588,#25589,
#25590,#25591,#25592,#25593,#25594,#25595,#25596,#25597,#25598,#25599,#25600,
#25601,#25602,#25603,#25604,#25605,#25606,#25607),.UNSPECIFIED.,.F.,.F.)
B_SPLINE_CURVE_WITH_KNOTS((6,1,1,1,1,1,1,1,1,1,1,1,1,1,1,1,1,1,1,1,1,1,
1,1,1,1,1,1,1,1,1,1,1,1,1,1,1,1,1,1,1,1,1,1,1,1,1,1,1,1,1,1,1,1,1,1,1,1,
1,1,1,1,1,1,1,6),(-1.,-0.984615384615383,-0.969230769230768,-0.953846153846152,
-0.938461538461537,-0.923076923076922,-0.907692307692306,-0.892307692307691,
-0.876923076923076,-0.86153846153846,-0.846153846153845,-0.83076923076923,
-0.815384615384614,-0.799999999999999,-0.784615384615384,-0.769230769230768,
-0.753846153846153,-0.738461538461538,-0.723076923076922,-0.707692307692307,
-0.692307692307692,-0.676923076923076,-0.661538461538461,-0.646153846153846,
-0.63076923076923,-0.615384615384615,-0.6,-0.584615384615384,-0.569230769230769,
-0.553846153846154,-0.538461538461538,-0.523076923076923,-0.507692307692308,
-0.492307692307692,-0.476923076923077,-0.461538461538462,-0.446153846153846,
-0.430769230769231,-0.415384615384615,-0.4,-0.384615384615385,-0.369230769230769,
-0.353846153846154,-0.338461538461538,-0.323076923076923,-0.307692307692308,
-0.292307692307692,-0.276923076923077,-0.261538461538462,-0.246153846153846,
-0.230769230769231,-0.215384615384615,-0.2,-0.184615384615385,-0.169230769230769,
-0.153846153846154,-0.138461538461538,-0.123076923076923,-0.107692307692308,
-0.0923076923076923,-0.0769230769230769,-0.0615384615384615,-0.0461538461538462,
-0.0307692307692308,-0.0153846153846154,0.),.UNSPECIFIED.)
CURVE()
GEOMETRIC_REPRESENTATION_ITEM()
RATIONAL_B_SPLINE_CURVE((1.,1.,1.,1.,1.,1.,1.,1.,1.,1.,1.,1.,1.,1.,1.,1.,
1.,1.,1.,1.,1.,1.,1.,1.,1.,1.,1.,1.,1.,1.,1.,1.,1.,1.,1.,1.,1.,1.,1.,1.,
1.,1.,1.,1.,1.,1.,1.,1.,1.,1.,1.,1.,1.,1.,1.,1.,1.,1.,1.,1.,1.,1.,1.,1.,
1.,1.,1.,1.,1.,1.))
REPRESENTATION_ITEM('')
);
#97=(
BOUNDED_CURVE()
B_SPLINE_CURVE(5,(#25754,#25755,#25756,#25757,#25758,#25759,#25760,#25761,
#25762,#25763,#25764,#25765,#25766,#25767,#25768,#25769,#25770,#25771,#25772,
#25773,#25774,#25775,#25776,#25777,#25778,#25779,#25780,#25781,#25782,#25783,
#25784,#25785,#25786,#25787,#25788,#25789,#25790,#25791,#25792,#25793,#25794,
#25795,#25796,#25797,#25798,#25799,#25800,#25801,#25802,#25803,#25804,#25805,
#25806,#25807,#25808,#25809,#25810,#25811,#25812,#25813,#25814,#25815,#25816,
#25817,#25818,#25819,#25820,#25821,#25822,#25823),.UNSPECIFIED.,.F.,.F.)
B_SPLINE_CURVE_WITH_KNOTS((6,1,1,1,1,1,1,1,1,1,1,1,1,1,1,1,1,1,1,1,1,1,
1,1,1,1,1,1,1,1,1,1,1,1,1,1,1,1,1,1,1,1,1,1,1,1,1,1,1,1,1,1,1,1,1,1,1,1,
1,1,1,1,1,1,1,6),(-1.,-0.984615384615383,-0.969230769230768,-0.953846153846152,
-0.938461538461537,-0.923076923076922,-0.907692307692306,-0.892307692307691,
-0.876923076923076,-0.86153846153846,-0.846153846153845,-0.83076923076923,
-0.815384615384614,-0.799999999999999,-0.784615384615384,-0.769230769230768,
-0.753846153846153,-0.738461538461538,-0.723076923076922,-0.707692307692307,
-0.692307692307692,-0.676923076923076,-0.661538461538461,-0.646153846153846,
-0.63076923076923,-0.615384615384615,-0.6,-0.584615384615384,-0.569230769230769,
-0.553846153846154,-0.538461538461538,-0.523076923076923,-0.507692307692308,
-0.492307692307692,-0.476923076923077,-0.461538461538462,-0.446153846153846,
-0.430769230769231,-0.415384615384615,-0.4,-0.384615384615385,-0.369230769230769,
-0.353846153846154,-0.338461538461538,-0.323076923076923,-0.307692307692308,
-0.292307692307692,-0.276923076923077,-0.261538461538462,-0.246153846153846,
-0.230769230769231,-0.215384615384615,-0.2,-0.184615384615385,-0.169230769230769,
-0.153846153846154,-0.138461538461538,-0.123076923076923,-0.107692307692308,
-0.0923076923076923,-0.0769230769230769,-0.0615384615384615,-0.0461538461538462,
-0.0307692307692308,-0.0153846153846154,0.),.UNSPECIFIED.)
CURVE()
GEOMETRIC_REPRESENTATION_ITEM()
RATIONAL_B_SPLINE_CURVE((1.,1.,1.,1.,1.,1.,1.,1.,1.,1.,1.,1.,1.,1.,1.,1.,
1.,1.,1.,1.,1.,1.,1.,1.,1.,1.,1.,1.,1.,1.,1.,1.,1.,1.,1.,1.,1.,1.,1.,1.,
1.,1.,1.,1.,1.,1.,1.,1.,1.,1.,1.,1.,1.,1.,1.,1.,1.,1.,1.,1.,1.,1.,1.,1.,
1.,1.,1.,1.,1.,1.))
REPRESENTATION_ITEM('')
);
#98=(
BOUNDED_CURVE()
B_SPLINE_CURVE(5,(#25970,#25971,#25972,#25973,#25974,#25975,#25976,#25977,
#25978,#25979,#25980,#25981,#25982,#25983,#25984,#25985,#25986,#25987,#25988,
#25989,#25990,#25991,#25992,#25993,#25994,#25995,#25996,#25997,#25998,#25999,
#26000,#26001,#26002,#26003,#26004,#26005,#26006,#26007,#26008,#26009,#26010,
#26011,#26012,#26013,#26014,#26015,#26016,#26017,#26018,#26019,#26020,#26021,
#26022,#26023,#26024,#26025,#26026,#26027,#26028,#26029,#26030,#26031,#26032,
#26033,#26034,#26035,#26036,#26037,#26038,#26039),.UNSPECIFIED.,.F.,.F.)
B_SPLINE_CURVE_WITH_KNOTS((6,1,1,1,1,1,1,1,1,1,1,1,1,1,1,1,1,1,1,1,1,1,
1,1,1,1,1,1,1,1,1,1,1,1,1,1,1,1,1,1,1,1,1,1,1,1,1,1,1,1,1,1,1,1,1,1,1,1,
1,1,1,1,1,1,1,6),(-1.,-0.984615384615383,-0.969230769230768,-0.953846153846152,
-0.938461538461537,-0.923076923076922,-0.907692307692306,-0.892307692307691,
-0.876923076923076,-0.86153846153846,-0.846153846153845,-0.83076923076923,
-0.815384615384614,-0.799999999999999,-0.784615384615384,-0.769230769230768,
-0.753846153846153,-0.738461538461538,-0.723076923076922,-0.707692307692307,
-0.692307692307692,-0.676923076923076,-0.661538461538461,-0.646153846153846,
-0.63076923076923,-0.615384615384615,-0.6,-0.584615384615384,-0.569230769230769,
-0.553846153846154,-0.538461538461538,-0.523076923076923,-0.507692307692308,
-0.492307692307692,-0.476923076923077,-0.461538461538462,-0.446153846153846,
-0.430769230769231,-0.415384615384615,-0.4,-0.384615384615385,-0.369230769230769,
-0.353846153846154,-0.338461538461538,-0.323076923076923,-0.307692307692308,
-0.292307692307692,-0.276923076923077,-0.261538461538462,-0.246153846153846,
-0.230769230769231,-0.215384615384615,-0.2,-0.184615384615385,-0.169230769230769,
-0.153846153846154,-0.138461538461538,-0.123076923076923,-0.107692307692308,
-0.0923076923076923,-0.0769230769230769,-0.0615384615384615,-0.0461538461538462,
-0.0307692307692308,-0.0153846153846154,0.),.UNSPECIFIED.)
CURVE()
GEOMETRIC_REPRESENTATION_ITEM()
RATIONAL_B_SPLINE_CURVE((1.,1.,1.,1.,1.,1.,1.,1.,1.,1.,1.,1.,1.,1.,1.,1.,
1.,1.,1.,1.,1.,1.,1.,1.,1.,1.,1.,1.,1.,1.,1.,1.,1.,1.,1.,1.,1.,1.,1.,1.,
1.,1.,1.,1.,1.,1.,1.,1.,1.,1.,1.,1.,1.,1.,1.,1.,1.,1.,1.,1.,1.,1.,1.,1.,
1.,1.,1.,1.,1.,1.))
REPRESENTATION_ITEM('')
);
#99=(
BOUNDED_CURVE()
B_SPLINE_CURVE(5,(#26186,#26187,#26188,#26189,#26190,#26191,#26192,#26193,
#26194,#26195,#26196,#26197,#26198,#26199,#26200,#26201,#26202,#26203,#26204,
#26205,#26206,#26207,#26208,#26209,#26210,#26211,#26212,#26213,#26214,#26215,
#26216,#26217,#26218,#26219,#26220,#26221,#26222,#26223,#26224,#26225,#26226,
#26227,#26228,#26229,#26230,#26231,#26232,#26233,#26234,#26235,#26236,#26237,
#26238,#26239,#26240,#26241,#26242,#26243,#26244,#26245,#26246,#26247,#26248,
#26249,#26250,#26251,#26252,#26253,#26254,#26255),.UNSPECIFIED.,.F.,.F.)
B_SPLINE_CURVE_WITH_KNOTS((6,1,1,1,1,1,1,1,1,1,1,1,1,1,1,1,1,1,1,1,1,1,
1,1,1,1,1,1,1,1,1,1,1,1,1,1,1,1,1,1,1,1,1,1,1,1,1,1,1,1,1,1,1,1,1,1,1,1,
1,1,1,1,1,1,1,6),(-1.,-0.984615384615383,-0.969230769230768,-0.953846153846152,
-0.938461538461537,-0.923076923076922,-0.907692307692306,-0.892307692307691,
-0.876923076923076,-0.86153846153846,-0.846153846153845,-0.83076923076923,
-0.815384615384614,-0.799999999999999,-0.784615384615384,-0.769230769230768,
-0.753846153846153,-0.738461538461538,-0.723076923076922,-0.707692307692307,
-0.692307692307692,-0.676923076923076,-0.661538461538461,-0.646153846153846,
-0.63076923076923,-0.615384615384615,-0.6,-0.584615384615384,-0.569230769230769,
-0.553846153846154,-0.538461538461538,-0.523076923076923,-0.507692307692308,
-0.492307692307692,-0.476923076923077,-0.461538461538462,-0.446153846153846,
-0.430769230769231,-0.415384615384615,-0.4,-0.384615384615385,-0.369230769230769,
-0.353846153846154,-0.338461538461538,-0.323076923076923,-0.307692307692308,
-0.292307692307692,-0.276923076923077,-0.261538461538462,-0.246153846153846,
-0.230769230769231,-0.215384615384615,-0.2,-0.184615384615385,-0.169230769230769,
-0.153846153846154,-0.138461538461538,-0.123076923076923,-0.107692307692308,
-0.0923076923076923,-0.0769230769230769,-0.0615384615384615,-0.0461538461538462,
-0.0307692307692308,-0.0153846153846154,0.),.UNSPECIFIED.)
CURVE()
GEOMETRIC_REPRESENTATION_ITEM()
RATIONAL_B_SPLINE_CURVE((1.,1.,1.,1.,1.,1.,1.,1.,1.,1.,1.,1.,1.,1.,1.,1.,
1.,1.,1.,1.,1.,1.,1.,1.,1.,1.,1.,1.,1.,1.,1.,1.,1.,1.,1.,1.,1.,1.,1.,1.,
1.,1.,1.,1.,1.,1.,1.,1.,1.,1.,1.,1.,1.,1.,1.,1.,1.,1.,1.,1.,1.,1.,1.,1.,
1.,1.,1.,1.,1.,1.))
REPRESENTATION_ITEM('')
);
#100=(
BOUNDED_CURVE()
B_SPLINE_CURVE(5,(#26402,#26403,#26404,#26405,#26406,#26407,#26408,#26409,
#26410,#26411,#26412,#26413,#26414,#26415,#26416,#26417,#26418,#26419,#26420,
#26421,#26422,#26423,#26424,#26425,#26426,#26427,#26428,#26429,#26430,#26431,
#26432,#26433,#26434,#26435,#26436,#26437,#26438,#26439,#26440,#26441,#26442,
#26443,#26444,#26445,#26446,#26447,#26448,#26449,#26450,#26451,#26452,#26453,
#26454,#26455,#26456,#26457,#26458,#26459,#26460,#26461,#26462,#26463,#26464,
#26465,#26466,#26467,#26468,#26469,#26470,#26471),.UNSPECIFIED.,.F.,.F.)
B_SPLINE_CURVE_WITH_KNOTS((6,1,1,1,1,1,1,1,1,1,1,1,1,1,1,1,1,1,1,1,1,1,
1,1,1,1,1,1,1,1,1,1,1,1,1,1,1,1,1,1,1,1,1,1,1,1,1,1,1,1,1,1,1,1,1,1,1,1,
1,1,1,1,1,1,1,6),(-1.,-0.984615384615383,-0.969230769230768,-0.953846153846152,
-0.938461538461537,-0.923076923076922,-0.907692307692306,-0.892307692307691,
-0.876923076923076,-0.86153846153846,-0.846153846153845,-0.83076923076923,
-0.815384615384614,-0.799999999999999,-0.784615384615384,-0.769230769230768,
-0.753846153846153,-0.738461538461538,-0.723076923076922,-0.707692307692307,
-0.692307692307692,-0.676923076923076,-0.661538461538461,-0.646153846153846,
-0.63076923076923,-0.615384615384615,-0.6,-0.584615384615384,-0.569230769230769,
-0.553846153846154,-0.538461538461538,-0.523076923076923,-0.507692307692308,
-0.492307692307692,-0.476923076923077,-0.461538461538462,-0.446153846153846,
-0.430769230769231,-0.415384615384615,-0.4,-0.384615384615385,-0.369230769230769,
-0.353846153846154,-0.338461538461538,-0.323076923076923,-0.307692307692308,
-0.292307692307692,-0.276923076923077,-0.261538461538462,-0.246153846153846,
-0.230769230769231,-0.215384615384615,-0.2,-0.184615384615385,-0.169230769230769,
-0.153846153846154,-0.138461538461538,-0.123076923076923,-0.107692307692308,
-0.0923076923076923,-0.0769230769230769,-0.0615384615384615,-0.0461538461538462,
-0.0307692307692308,-0.0153846153846154,0.),.UNSPECIFIED.)
CURVE()
GEOMETRIC_REPRESENTATION_ITEM()
RATIONAL_B_SPLINE_CURVE((1.,1.,1.,1.,1.,1.,1.,1.,1.,1.,1.,1.,1.,1.,1.,1.,
1.,1.,1.,1.,1.,1.,1.,1.,1.,1.,1.,1.,1.,1.,1.,1.,1.,1.,1.,1.,1.,1.,1.,1.,
1.,1.,1.,1.,1.,1.,1.,1.,1.,1.,1.,1.,1.,1.,1.,1.,1.,1.,1.,1.,1.,1.,1.,1.,
1.,1.,1.,1.,1.,1.))
REPRESENTATION_ITEM('')
);
#101=(
BOUNDED_CURVE()
B_SPLINE_CURVE(5,(#26618,#26619,#26620,#26621,#26622,#26623,#26624,#26625,
#26626,#26627,#26628,#26629,#26630,#26631,#26632,#26633,#26634,#26635,#26636,
#26637,#26638,#26639,#26640,#26641,#26642,#26643,#26644,#26645,#26646,#26647,
#26648,#26649,#26650,#26651,#26652,#26653,#26654,#26655,#26656,#26657,#26658,
#26659,#26660,#26661,#26662,#26663,#26664,#26665,#26666,#26667,#26668,#26669,
#26670,#26671,#26672,#26673,#26674,#26675,#26676,#26677,#26678,#26679,#26680,
#26681,#26682,#26683,#26684,#26685,#26686,#26687),.UNSPECIFIED.,.F.,.F.)
B_SPLINE_CURVE_WITH_KNOTS((6,1,1,1,1,1,1,1,1,1,1,1,1,1,1,1,1,1,1,1,1,1,
1,1,1,1,1,1,1,1,1,1,1,1,1,1,1,1,1,1,1,1,1,1,1,1,1,1,1,1,1,1,1,1,1,1,1,1,
1,1,1,1,1,1,1,6),(-1.,-0.984615384615383,-0.969230769230768,-0.953846153846152,
-0.938461538461537,-0.923076923076922,-0.907692307692306,-0.892307692307691,
-0.876923076923076,-0.86153846153846,-0.846153846153845,-0.83076923076923,
-0.815384615384614,-0.799999999999999,-0.784615384615384,-0.769230769230768,
-0.753846153846153,-0.738461538461538,-0.723076923076922,-0.707692307692307,
-0.692307692307692,-0.676923076923076,-0.661538461538461,-0.646153846153846,
-0.63076923076923,-0.615384615384615,-0.6,-0.584615384615384,-0.569230769230769,
-0.553846153846154,-0.538461538461538,-0.523076923076923,-0.507692307692308,
-0.492307692307692,-0.476923076923077,-0.461538461538462,-0.446153846153846,
-0.430769230769231,-0.415384615384615,-0.4,-0.384615384615385,-0.369230769230769,
-0.353846153846154,-0.338461538461538,-0.323076923076923,-0.307692307692308,
-0.292307692307692,-0.276923076923077,-0.261538461538462,-0.246153846153846,
-0.230769230769231,-0.215384615384615,-0.2,-0.184615384615385,-0.169230769230769,
-0.153846153846154,-0.138461538461538,-0.123076923076923,-0.107692307692308,
-0.0923076923076923,-0.0769230769230769,-0.0615384615384615,-0.0461538461538462,
-0.0307692307692308,-0.0153846153846154,0.),.UNSPECIFIED.)
CURVE()
GEOMETRIC_REPRESENTATION_ITEM()
RATIONAL_B_SPLINE_CURVE((1.,1.,1.,1.,1.,1.,1.,1.,1.,1.,1.,1.,1.,1.,1.,1.,
1.,1.,1.,1.,1.,1.,1.,1.,1.,1.,1.,1.,1.,1.,1.,1.,1.,1.,1.,1.,1.,1.,1.,1.,
1.,1.,1.,1.,1.,1.,1.,1.,1.,1.,1.,1.,1.,1.,1.,1.,1.,1.,1.,1.,1.,1.,1.,1.,
1.,1.,1.,1.,1.,1.))
REPRESENTATION_ITEM('')
);
#102=(
BOUNDED_CURVE()
B_SPLINE_CURVE(5,(#26834,#26835,#26836,#26837,#26838,#26839,#26840,#26841,
#26842,#26843,#26844,#26845,#26846,#26847,#26848,#26849,#26850,#26851,#26852,
#26853,#26854,#26855,#26856,#26857,#26858,#26859,#26860,#26861,#26862,#26863,
#26864,#26865,#26866,#26867,#26868,#26869,#26870,#26871,#26872,#26873,#26874,
#26875,#26876,#26877,#26878,#26879,#26880,#26881,#26882,#26883,#26884,#26885,
#26886,#26887,#26888,#26889,#26890,#26891,#26892,#26893,#26894,#26895,#26896,
#26897,#26898,#26899,#26900,#26901,#26902,#26903),.UNSPECIFIED.,.F.,.F.)
B_SPLINE_CURVE_WITH_KNOTS((6,1,1,1,1,1,1,1,1,1,1,1,1,1,1,1,1,1,1,1,1,1,
1,1,1,1,1,1,1,1,1,1,1,1,1,1,1,1,1,1,1,1,1,1,1,1,1,1,1,1,1,1,1,1,1,1,1,1,
1,1,1,1,1,1,1,6),(-1.,-0.984615384615383,-0.969230769230768,-0.953846153846152,
-0.938461538461537,-0.923076923076922,-0.907692307692306,-0.892307692307691,
-0.876923076923076,-0.86153846153846,-0.846153846153845,-0.83076923076923,
-0.815384615384614,-0.799999999999999,-0.784615384615384,-0.769230769230768,
-0.753846153846153,-0.738461538461538,-0.723076923076922,-0.707692307692307,
-0.692307692307692,-0.676923076923076,-0.661538461538461,-0.646153846153846,
-0.63076923076923,-0.615384615384615,-0.6,-0.584615384615384,-0.569230769230769,
-0.553846153846154,-0.538461538461538,-0.523076923076923,-0.507692307692308,
-0.492307692307692,-0.476923076923077,-0.461538461538462,-0.446153846153846,
-0.430769230769231,-0.415384615384615,-0.4,-0.384615384615385,-0.369230769230769,
-0.353846153846154,-0.338461538461538,-0.323076923076923,-0.307692307692308,
-0.292307692307692,-0.276923076923077,-0.261538461538462,-0.246153846153846,
-0.230769230769231,-0.215384615384615,-0.2,-0.184615384615385,-0.169230769230769,
-0.153846153846154,-0.138461538461538,-0.123076923076923,-0.107692307692308,
-0.0923076923076923,-0.0769230769230769,-0.0615384615384615,-0.0461538461538462,
-0.0307692307692308,-0.0153846153846154,0.),.UNSPECIFIED.)
CURVE()
GEOMETRIC_REPRESENTATION_ITEM()
RATIONAL_B_SPLINE_CURVE((1.,1.,1.,1.,1.,1.,1.,1.,1.,1.,1.,1.,1.,1.,1.,1.,
1.,1.,1.,1.,1.,1.,1.,1.,1.,1.,1.,1.,1.,1.,1.,1.,1.,1.,1.,1.,1.,1.,1.,1.,
1.,1.,1.,1.,1.,1.,1.,1.,1.,1.,1.,1.,1.,1.,1.,1.,1.,1.,1.,1.,1.,1.,1.,1.,
1.,1.,1.,1.,1.,1.))
REPRESENTATION_ITEM('')
);
#103=(
BOUNDED_CURVE()
B_SPLINE_CURVE(5,(#27050,#27051,#27052,#27053,#27054,#27055,#27056,#27057,
#27058,#27059,#27060,#27061,#27062,#27063,#27064,#27065,#27066,#27067,#27068,
#27069,#27070,#27071,#27072,#27073,#27074,#27075,#27076,#27077,#27078,#27079,
#27080,#27081,#27082,#27083,#27084,#27085,#27086,#27087,#27088,#27089,#27090,
#27091,#27092,#27093,#27094,#27095,#27096,#27097,#27098,#27099,#27100,#27101,
#27102,#27103,#27104,#27105,#27106,#27107,#27108,#27109,#27110,#27111,#27112,
#27113,#27114,#27115,#27116,#27117,#27118,#27119),.UNSPECIFIED.,.F.,.F.)
B_SPLINE_CURVE_WITH_KNOTS((6,1,1,1,1,1,1,1,1,1,1,1,1,1,1,1,1,1,1,1,1,1,
1,1,1,1,1,1,1,1,1,1,1,1,1,1,1,1,1,1,1,1,1,1,1,1,1,1,1,1,1,1,1,1,1,1,1,1,
1,1,1,1,1,1,1,6),(-1.,-0.984615384615383,-0.969230769230768,-0.953846153846152,
-0.938461538461537,-0.923076923076922,-0.907692307692306,-0.892307692307691,
-0.876923076923076,-0.86153846153846,-0.846153846153845,-0.83076923076923,
-0.815384615384614,-0.799999999999999,-0.784615384615384,-0.769230769230768,
-0.753846153846153,-0.738461538461538,-0.723076923076922,-0.707692307692307,
-0.692307692307692,-0.676923076923076,-0.661538461538461,-0.646153846153846,
-0.63076923076923,-0.615384615384615,-0.6,-0.584615384615384,-0.569230769230769,
-0.553846153846154,-0.538461538461538,-0.523076923076923,-0.507692307692308,
-0.492307692307692,-0.476923076923077,-0.461538461538462,-0.446153846153846,
-0.430769230769231,-0.415384615384615,-0.4,-0.384615384615385,-0.369230769230769,
-0.353846153846154,-0.338461538461538,-0.323076923076923,-0.307692307692308,
-0.292307692307692,-0.276923076923077,-0.261538461538462,-0.246153846153846,
-0.230769230769231,-0.215384615384615,-0.2,-0.184615384615385,-0.169230769230769,
-0.153846153846154,-0.138461538461538,-0.123076923076923,-0.107692307692308,
-0.0923076923076923,-0.0769230769230769,-0.0615384615384615,-0.0461538461538462,
-0.0307692307692308,-0.0153846153846154,0.),.UNSPECIFIED.)
CURVE()
GEOMETRIC_REPRESENTATION_ITEM()
RATIONAL_B_SPLINE_CURVE((1.,1.,1.,1.,1.,1.,1.,1.,1.,1.,1.,1.,1.,1.,1.,1.,
1.,1.,1.,1.,1.,1.,1.,1.,1.,1.,1.,1.,1.,1.,1.,1.,1.,1.,1.,1.,1.,1.,1.,1.,
1.,1.,1.,1.,1.,1.,1.,1.,1.,1.,1.,1.,1.,1.,1.,1.,1.,1.,1.,1.,1.,1.,1.,1.,
1.,1.,1.,1.,1.,1.))
REPRESENTATION_ITEM('')
);
#104=(
BOUNDED_CURVE()
B_SPLINE_CURVE(5,(#27266,#27267,#27268,#27269,#27270,#27271,#27272,#27273,
#27274,#27275,#27276,#27277,#27278,#27279,#27280,#27281,#27282,#27283,#27284,
#27285,#27286,#27287,#27288,#27289,#27290,#27291,#27292,#27293,#27294,#27295,
#27296,#27297,#27298,#27299,#27300,#27301,#27302,#27303,#27304,#27305,#27306,
#27307,#27308,#27309,#27310,#27311,#27312,#27313,#27314,#27315,#27316,#27317,
#27318,#27319,#27320,#27321,#27322,#27323,#27324,#27325,#27326,#27327,#27328,
#27329,#27330,#27331,#27332,#27333,#27334,#27335),.UNSPECIFIED.,.F.,.F.)
B_SPLINE_CURVE_WITH_KNOTS((6,1,1,1,1,1,1,1,1,1,1,1,1,1,1,1,1,1,1,1,1,1,
1,1,1,1,1,1,1,1,1,1,1,1,1,1,1,1,1,1,1,1,1,1,1,1,1,1,1,1,1,1,1,1,1,1,1,1,
1,1,1,1,1,1,1,6),(-1.,-0.984615384615383,-0.969230769230768,-0.953846153846152,
-0.938461538461537,-0.923076923076922,-0.907692307692306,-0.892307692307691,
-0.876923076923076,-0.86153846153846,-0.846153846153845,-0.83076923076923,
-0.815384615384614,-0.799999999999999,-0.784615384615384,-0.769230769230768,
-0.753846153846153,-0.738461538461538,-0.723076923076922,-0.707692307692307,
-0.692307692307692,-0.676923076923076,-0.661538461538461,-0.646153846153846,
-0.63076923076923,-0.615384615384615,-0.6,-0.584615384615384,-0.569230769230769,
-0.553846153846154,-0.538461538461538,-0.523076923076923,-0.507692307692308,
-0.492307692307692,-0.476923076923077,-0.461538461538462,-0.446153846153846,
-0.430769230769231,-0.415384615384615,-0.4,-0.384615384615385,-0.369230769230769,
-0.353846153846154,-0.338461538461538,-0.323076923076923,-0.307692307692308,
-0.292307692307692,-0.276923076923077,-0.261538461538462,-0.246153846153846,
-0.230769230769231,-0.215384615384615,-0.2,-0.184615384615385,-0.169230769230769,
-0.153846153846154,-0.138461538461538,-0.123076923076923,-0.107692307692308,
-0.0923076923076923,-0.0769230769230769,-0.0615384615384615,-0.0461538461538462,
-0.0307692307692308,-0.0153846153846154,0.),.UNSPECIFIED.)
CURVE()
GEOMETRIC_REPRESENTATION_ITEM()
RATIONAL_B_SPLINE_CURVE((1.,1.,1.,1.,1.,1.,1.,1.,1.,1.,1.,1.,1.,1.,1.,1.,
1.,1.,1.,1.,1.,1.,1.,1.,1.,1.,1.,1.,1.,1.,1.,1.,1.,1.,1.,1.,1.,1.,1.,1.,
1.,1.,1.,1.,1.,1.,1.,1.,1.,1.,1.,1.,1.,1.,1.,1.,1.,1.,1.,1.,1.,1.,1.,1.,
1.,1.,1.,1.,1.,1.))
REPRESENTATION_ITEM('')
);
#105=(
BOUNDED_CURVE()
B_SPLINE_CURVE(5,(#27482,#27483,#27484,#27485,#27486,#27487,#27488,#27489,
#27490,#27491,#27492,#27493,#27494,#27495,#27496,#27497,#27498,#27499,#27500,
#27501,#27502,#27503,#27504,#27505,#27506,#27507,#27508,#27509,#27510,#27511,
#27512,#27513,#27514,#27515,#27516,#27517,#27518,#27519,#27520,#27521,#27522,
#27523,#27524,#27525,#27526,#27527,#27528,#27529,#27530,#27531,#27532,#27533,
#27534,#27535,#27536,#27537,#27538,#27539,#27540,#27541,#27542,#27543,#27544,
#27545,#27546,#27547,#27548,#27549,#27550,#27551),.UNSPECIFIED.,.F.,.F.)
B_SPLINE_CURVE_WITH_KNOTS((6,1,1,1,1,1,1,1,1,1,1,1,1,1,1,1,1,1,1,1,1,1,
1,1,1,1,1,1,1,1,1,1,1,1,1,1,1,1,1,1,1,1,1,1,1,1,1,1,1,1,1,1,1,1,1,1,1,1,
1,1,1,1,1,1,1,6),(-1.,-0.984615384615383,-0.969230769230768,-0.953846153846152,
-0.938461538461537,-0.923076923076922,-0.907692307692306,-0.892307692307691,
-0.876923076923076,-0.86153846153846,-0.846153846153845,-0.83076923076923,
-0.815384615384614,-0.799999999999999,-0.784615384615384,-0.769230769230768,
-0.753846153846153,-0.738461538461538,-0.723076923076922,-0.707692307692307,
-0.692307692307692,-0.676923076923076,-0.661538461538461,-0.646153846153846,
-0.63076923076923,-0.615384615384615,-0.6,-0.584615384615384,-0.569230769230769,
-0.553846153846154,-0.538461538461538,-0.523076923076923,-0.507692307692308,
-0.492307692307692,-0.476923076923077,-0.461538461538462,-0.446153846153846,
-0.430769230769231,-0.415384615384615,-0.4,-0.384615384615385,-0.369230769230769,
-0.353846153846154,-0.338461538461538,-0.323076923076923,-0.307692307692308,
-0.292307692307692,-0.276923076923077,-0.261538461538462,-0.246153846153846,
-0.230769230769231,-0.215384615384615,-0.2,-0.184615384615385,-0.169230769230769,
-0.153846153846154,-0.138461538461538,-0.123076923076923,-0.107692307692308,
-0.0923076923076923,-0.0769230769230769,-0.0615384615384615,-0.0461538461538462,
-0.0307692307692308,-0.0153846153846154,0.),.UNSPECIFIED.)
CURVE()
GEOMETRIC_REPRESENTATION_ITEM()
RATIONAL_B_SPLINE_CURVE((1.,1.,1.,1.,1.,1.,1.,1.,1.,1.,1.,1.,1.,1.,1.,1.,
1.,1.,1.,1.,1.,1.,1.,1.,1.,1.,1.,1.,1.,1.,1.,1.,1.,1.,1.,1.,1.,1.,1.,1.,
1.,1.,1.,1.,1.,1.,1.,1.,1.,1.,1.,1.,1.,1.,1.,1.,1.,1.,1.,1.,1.,1.,1.,1.,
1.,1.,1.,1.,1.,1.))
REPRESENTATION_ITEM('')
);
#106=(
BOUNDED_CURVE()
B_SPLINE_CURVE(5,(#27698,#27699,#27700,#27701,#27702,#27703,#27704,#27705,
#27706,#27707,#27708,#27709,#27710,#27711,#27712,#27713,#27714,#27715,#27716,
#27717,#27718,#27719,#27720,#27721,#27722,#27723,#27724,#27725,#27726,#27727,
#27728,#27729,#27730,#27731,#27732,#27733,#27734,#27735,#27736,#27737,#27738,
#27739,#27740,#27741,#27742,#27743,#27744,#27745,#27746,#27747,#27748,#27749,
#27750,#27751,#27752,#27753,#27754,#27755,#27756,#27757,#27758,#27759,#27760,
#27761,#27762,#27763,#27764,#27765,#27766,#27767),.UNSPECIFIED.,.F.,.F.)
B_SPLINE_CURVE_WITH_KNOTS((6,1,1,1,1,1,1,1,1,1,1,1,1,1,1,1,1,1,1,1,1,1,
1,1,1,1,1,1,1,1,1,1,1,1,1,1,1,1,1,1,1,1,1,1,1,1,1,1,1,1,1,1,1,1,1,1,1,1,
1,1,1,1,1,1,1,6),(-1.,-0.984615384615383,-0.969230769230768,-0.953846153846152,
-0.938461538461537,-0.923076923076922,-0.907692307692306,-0.892307692307691,
-0.876923076923076,-0.86153846153846,-0.846153846153845,-0.83076923076923,
-0.815384615384614,-0.799999999999999,-0.784615384615384,-0.769230769230768,
-0.753846153846153,-0.738461538461538,-0.723076923076922,-0.707692307692307,
-0.692307692307692,-0.676923076923076,-0.661538461538461,-0.646153846153846,
-0.63076923076923,-0.615384615384615,-0.6,-0.584615384615384,-0.569230769230769,
-0.553846153846154,-0.538461538461538,-0.523076923076923,-0.507692307692308,
-0.492307692307692,-0.476923076923077,-0.461538461538462,-0.446153846153846,
-0.430769230769231,-0.415384615384615,-0.4,-0.384615384615385,-0.369230769230769,
-0.353846153846154,-0.338461538461538,-0.323076923076923,-0.307692307692308,
-0.292307692307692,-0.276923076923077,-0.261538461538462,-0.246153846153846,
-0.230769230769231,-0.215384615384615,-0.2,-0.184615384615385,-0.169230769230769,
-0.153846153846154,-0.138461538461538,-0.123076923076923,-0.107692307692308,
-0.0923076923076923,-0.0769230769230769,-0.0615384615384615,-0.0461538461538462,
-0.0307692307692308,-0.0153846153846154,0.),.UNSPECIFIED.)
CURVE()
GEOMETRIC_REPRESENTATION_ITEM()
RATIONAL_B_SPLINE_CURVE((1.,1.,1.,1.,1.,1.,1.,1.,1.,1.,1.,1.,1.,1.,1.,1.,
1.,1.,1.,1.,1.,1.,1.,1.,1.,1.,1.,1.,1.,1.,1.,1.,1.,1.,1.,1.,1.,1.,1.,1.,
1.,1.,1.,1.,1.,1.,1.,1.,1.,1.,1.,1.,1.,1.,1.,1.,1.,1.,1.,1.,1.,1.,1.,1.,
1.,1.,1.,1.,1.,1.))
REPRESENTATION_ITEM('')
);
#107=(
BOUNDED_CURVE()
B_SPLINE_CURVE(5,(#27914,#27915,#27916,#27917,#27918,#27919,#27920,#27921,
#27922,#27923,#27924,#27925,#27926,#27927,#27928,#27929,#27930,#27931,#27932,
#27933,#27934,#27935,#27936,#27937,#27938,#27939,#27940,#27941,#27942,#27943,
#27944,#27945,#27946,#27947,#27948,#27949,#27950,#27951,#27952,#27953,#27954,
#27955,#27956,#27957,#27958,#27959,#27960,#27961,#27962,#27963,#27964,#27965,
#27966,#27967,#27968,#27969,#27970,#27971,#27972,#27973,#27974,#27975,#27976,
#27977,#27978,#27979,#27980,#27981,#27982,#27983),.UNSPECIFIED.,.F.,.F.)
B_SPLINE_CURVE_WITH_KNOTS((6,1,1,1,1,1,1,1,1,1,1,1,1,1,1,1,1,1,1,1,1,1,
1,1,1,1,1,1,1,1,1,1,1,1,1,1,1,1,1,1,1,1,1,1,1,1,1,1,1,1,1,1,1,1,1,1,1,1,
1,1,1,1,1,1,1,6),(-1.,-0.984615384615383,-0.969230769230768,-0.953846153846152,
-0.938461538461537,-0.923076923076922,-0.907692307692306,-0.892307692307691,
-0.876923076923076,-0.86153846153846,-0.846153846153845,-0.83076923076923,
-0.815384615384614,-0.799999999999999,-0.784615384615384,-0.769230769230768,
-0.753846153846153,-0.738461538461538,-0.723076923076922,-0.707692307692307,
-0.692307692307692,-0.676923076923076,-0.661538461538461,-0.646153846153846,
-0.63076923076923,-0.615384615384615,-0.6,-0.584615384615384,-0.569230769230769,
-0.553846153846154,-0.538461538461538,-0.523076923076923,-0.507692307692308,
-0.492307692307692,-0.476923076923077,-0.461538461538462,-0.446153846153846,
-0.430769230769231,-0.415384615384615,-0.4,-0.384615384615385,-0.369230769230769,
-0.353846153846154,-0.338461538461538,-0.323076923076923,-0.307692307692308,
-0.292307692307692,-0.276923076923077,-0.261538461538462,-0.246153846153846,
-0.230769230769231,-0.215384615384615,-0.2,-0.184615384615385,-0.169230769230769,
-0.153846153846154,-0.138461538461538,-0.123076923076923,-0.107692307692308,
-0.0923076923076923,-0.0769230769230769,-0.0615384615384615,-0.0461538461538462,
-0.0307692307692308,-0.0153846153846154,0.),.UNSPECIFIED.)
CURVE()
GEOMETRIC_REPRESENTATION_ITEM()
RATIONAL_B_SPLINE_CURVE((1.,1.,1.,1.,1.,1.,1.,1.,1.,1.,1.,1.,1.,1.,1.,1.,
1.,1.,1.,1.,1.,1.,1.,1.,1.,1.,1.,1.,1.,1.,1.,1.,1.,1.,1.,1.,1.,1.,1.,1.,
1.,1.,1.,1.,1.,1.,1.,1.,1.,1.,1.,1.,1.,1.,1.,1.,1.,1.,1.,1.,1.,1.,1.,1.,
1.,1.,1.,1.,1.,1.))
REPRESENTATION_ITEM('')
);
#108=(
BOUNDED_CURVE()
B_SPLINE_CURVE(5,(#28130,#28131,#28132,#28133,#28134,#28135,#28136,#28137,
#28138,#28139,#28140,#28141,#28142,#28143,#28144,#28145,#28146,#28147,#28148,
#28149,#28150,#28151,#28152,#28153,#28154,#28155,#28156,#28157,#28158,#28159,
#28160,#28161,#28162,#28163,#28164,#28165,#28166,#28167,#28168,#28169,#28170,
#28171,#28172,#28173,#28174,#28175,#28176,#28177,#28178,#28179,#28180,#28181,
#28182,#28183,#28184,#28185,#28186,#28187,#28188,#28189,#28190,#28191,#28192,
#28193,#28194,#28195,#28196,#28197,#28198,#28199),.UNSPECIFIED.,.F.,.F.)
B_SPLINE_CURVE_WITH_KNOTS((6,1,1,1,1,1,1,1,1,1,1,1,1,1,1,1,1,1,1,1,1,1,
1,1,1,1,1,1,1,1,1,1,1,1,1,1,1,1,1,1,1,1,1,1,1,1,1,1,1,1,1,1,1,1,1,1,1,1,
1,1,1,1,1,1,1,6),(-1.,-0.984615384615383,-0.969230769230768,-0.953846153846152,
-0.938461538461537,-0.923076923076922,-0.907692307692306,-0.892307692307691,
-0.876923076923076,-0.86153846153846,-0.846153846153845,-0.83076923076923,
-0.815384615384614,-0.799999999999999,-0.784615384615384,-0.769230769230768,
-0.753846153846153,-0.738461538461538,-0.723076923076922,-0.707692307692307,
-0.692307692307692,-0.676923076923076,-0.661538461538461,-0.646153846153846,
-0.63076923076923,-0.615384615384615,-0.6,-0.584615384615384,-0.569230769230769,
-0.553846153846154,-0.538461538461538,-0.523076923076923,-0.507692307692308,
-0.492307692307692,-0.476923076923077,-0.461538461538462,-0.446153846153846,
-0.430769230769231,-0.415384615384615,-0.4,-0.384615384615385,-0.369230769230769,
-0.353846153846154,-0.338461538461538,-0.323076923076923,-0.307692307692308,
-0.292307692307692,-0.276923076923077,-0.261538461538462,-0.246153846153846,
-0.230769230769231,-0.215384615384615,-0.2,-0.184615384615385,-0.169230769230769,
-0.153846153846154,-0.138461538461538,-0.123076923076923,-0.107692307692308,
-0.0923076923076923,-0.0769230769230769,-0.0615384615384615,-0.0461538461538462,
-0.0307692307692308,-0.0153846153846154,0.),.UNSPECIFIED.)
CURVE()
GEOMETRIC_REPRESENTATION_ITEM()
RATIONAL_B_SPLINE_CURVE((1.,1.,1.,1.,1.,1.,1.,1.,1.,1.,1.,1.,1.,1.,1.,1.,
1.,1.,1.,1.,1.,1.,1.,1.,1.,1.,1.,1.,1.,1.,1.,1.,1.,1.,1.,1.,1.,1.,1.,1.,
1.,1.,1.,1.,1.,1.,1.,1.,1.,1.,1.,1.,1.,1.,1.,1.,1.,1.,1.,1.,1.,1.,1.,1.,
1.,1.,1.,1.,1.,1.))
REPRESENTATION_ITEM('')
);
#109=(
BOUNDED_CURVE()
B_SPLINE_CURVE(5,(#28346,#28347,#28348,#28349,#28350,#28351,#28352,#28353,
#28354,#28355,#28356,#28357,#28358,#28359,#28360,#28361,#28362,#28363,#28364,
#28365,#28366,#28367,#28368,#28369,#28370,#28371,#28372,#28373,#28374,#28375,
#28376,#28377,#28378,#28379,#28380,#28381,#28382,#28383,#28384,#28385,#28386,
#28387,#28388,#28389,#28390,#28391,#28392,#28393,#28394,#28395,#28396,#28397,
#28398,#28399,#28400,#28401,#28402,#28403,#28404,#28405,#28406,#28407,#28408,
#28409,#28410,#28411,#28412,#28413,#28414,#28415),.UNSPECIFIED.,.F.,.F.)
B_SPLINE_CURVE_WITH_KNOTS((6,1,1,1,1,1,1,1,1,1,1,1,1,1,1,1,1,1,1,1,1,1,
1,1,1,1,1,1,1,1,1,1,1,1,1,1,1,1,1,1,1,1,1,1,1,1,1,1,1,1,1,1,1,1,1,1,1,1,
1,1,1,1,1,1,1,6),(-1.,-0.984615384615383,-0.969230769230768,-0.953846153846152,
-0.938461538461537,-0.923076923076922,-0.907692307692306,-0.892307692307691,
-0.876923076923076,-0.86153846153846,-0.846153846153845,-0.83076923076923,
-0.815384615384614,-0.799999999999999,-0.784615384615384,-0.769230769230768,
-0.753846153846153,-0.738461538461538,-0.723076923076922,-0.707692307692307,
-0.692307692307692,-0.676923076923076,-0.661538461538461,-0.646153846153846,
-0.63076923076923,-0.615384615384615,-0.6,-0.584615384615384,-0.569230769230769,
-0.553846153846154,-0.538461538461538,-0.523076923076923,-0.507692307692308,
-0.492307692307692,-0.476923076923077,-0.461538461538462,-0.446153846153846,
-0.430769230769231,-0.415384615384615,-0.4,-0.384615384615385,-0.369230769230769,
-0.353846153846154,-0.338461538461538,-0.323076923076923,-0.307692307692308,
-0.292307692307692,-0.276923076923077,-0.261538461538462,-0.246153846153846,
-0.230769230769231,-0.215384615384615,-0.2,-0.184615384615385,-0.169230769230769,
-0.153846153846154,-0.138461538461538,-0.123076923076923,-0.107692307692308,
-0.0923076923076923,-0.0769230769230769,-0.0615384615384615,-0.0461538461538462,
-0.0307692307692308,-0.0153846153846154,0.),.UNSPECIFIED.)
CURVE()
GEOMETRIC_REPRESENTATION_ITEM()
RATIONAL_B_SPLINE_CURVE((1.,1.,1.,1.,1.,1.,1.,1.,1.,1.,1.,1.,1.,1.,1.,1.,
1.,1.,1.,1.,1.,1.,1.,1.,1.,1.,1.,1.,1.,1.,1.,1.,1.,1.,1.,1.,1.,1.,1.,1.,
1.,1.,1.,1.,1.,1.,1.,1.,1.,1.,1.,1.,1.,1.,1.,1.,1.,1.,1.,1.,1.,1.,1.,1.,
1.,1.,1.,1.,1.,1.))
REPRESENTATION_ITEM('')
);
#110=(
BOUNDED_CURVE()
B_SPLINE_CURVE(5,(#28562,#28563,#28564,#28565,#28566,#28567,#28568,#28569,
#28570,#28571,#28572,#28573,#28574,#28575,#28576,#28577,#28578,#28579,#28580,
#28581,#28582,#28583,#28584,#28585,#28586,#28587,#28588,#28589,#28590,#28591,
#28592,#28593,#28594,#28595,#28596,#28597,#28598,#28599,#28600,#28601,#28602,
#28603,#28604,#28605,#28606,#28607,#28608,#28609,#28610,#28611,#28612,#28613,
#28614,#28615,#28616,#28617,#28618,#28619,#28620,#28621,#28622,#28623,#28624,
#28625,#28626,#28627,#28628,#28629,#28630,#28631),.UNSPECIFIED.,.F.,.F.)
B_SPLINE_CURVE_WITH_KNOTS((6,1,1,1,1,1,1,1,1,1,1,1,1,1,1,1,1,1,1,1,1,1,
1,1,1,1,1,1,1,1,1,1,1,1,1,1,1,1,1,1,1,1,1,1,1,1,1,1,1,1,1,1,1,1,1,1,1,1,
1,1,1,1,1,1,1,6),(-1.,-0.984615384615383,-0.969230769230768,-0.953846153846152,
-0.938461538461537,-0.923076923076922,-0.907692307692306,-0.892307692307691,
-0.876923076923076,-0.86153846153846,-0.846153846153845,-0.83076923076923,
-0.815384615384614,-0.799999999999999,-0.784615384615384,-0.769230769230768,
-0.753846153846153,-0.738461538461538,-0.723076923076922,-0.707692307692307,
-0.692307692307692,-0.676923076923076,-0.661538461538461,-0.646153846153846,
-0.63076923076923,-0.615384615384615,-0.6,-0.584615384615384,-0.569230769230769,
-0.553846153846154,-0.538461538461538,-0.523076923076923,-0.507692307692308,
-0.492307692307692,-0.476923076923077,-0.461538461538462,-0.446153846153846,
-0.430769230769231,-0.415384615384615,-0.4,-0.384615384615385,-0.369230769230769,
-0.353846153846154,-0.338461538461538,-0.323076923076923,-0.307692307692308,
-0.292307692307692,-0.276923076923077,-0.261538461538462,-0.246153846153846,
-0.230769230769231,-0.215384615384615,-0.2,-0.184615384615385,-0.169230769230769,
-0.153846153846154,-0.138461538461538,-0.123076923076923,-0.107692307692308,
-0.0923076923076923,-0.0769230769230769,-0.0615384615384615,-0.0461538461538462,
-0.0307692307692308,-0.0153846153846154,0.),.UNSPECIFIED.)
CURVE()
GEOMETRIC_REPRESENTATION_ITEM()
RATIONAL_B_SPLINE_CURVE((1.,1.,1.,1.,1.,1.,1.,1.,1.,1.,1.,1.,1.,1.,1.,1.,
1.,1.,1.,1.,1.,1.,1.,1.,1.,1.,1.,1.,1.,1.,1.,1.,1.,1.,1.,1.,1.,1.,1.,1.,
1.,1.,1.,1.,1.,1.,1.,1.,1.,1.,1.,1.,1.,1.,1.,1.,1.,1.,1.,1.,1.,1.,1.,1.,
1.,1.,1.,1.,1.,1.))
REPRESENTATION_ITEM('')
);
#111=(
BOUNDED_CURVE()
B_SPLINE_CURVE(5,(#28778,#28779,#28780,#28781,#28782,#28783,#28784,#28785,
#28786,#28787,#28788,#28789,#28790,#28791,#28792,#28793,#28794,#28795,#28796,
#28797,#28798,#28799,#28800,#28801,#28802,#28803,#28804,#28805,#28806,#28807,
#28808,#28809,#28810,#28811,#28812,#28813,#28814,#28815,#28816,#28817,#28818,
#28819,#28820,#28821,#28822,#28823,#28824,#28825,#28826,#28827,#28828,#28829,
#28830,#28831,#28832,#28833,#28834,#28835,#28836,#28837,#28838,#28839,#28840,
#28841,#28842,#28843,#28844,#28845,#28846,#28847),.UNSPECIFIED.,.F.,.F.)
B_SPLINE_CURVE_WITH_KNOTS((6,1,1,1,1,1,1,1,1,1,1,1,1,1,1,1,1,1,1,1,1,1,
1,1,1,1,1,1,1,1,1,1,1,1,1,1,1,1,1,1,1,1,1,1,1,1,1,1,1,1,1,1,1,1,1,1,1,1,
1,1,1,1,1,1,1,6),(-1.,-0.984615384615383,-0.969230769230768,-0.953846153846152,
-0.938461538461537,-0.923076923076922,-0.907692307692306,-0.892307692307691,
-0.876923076923076,-0.86153846153846,-0.846153846153845,-0.83076923076923,
-0.815384615384614,-0.799999999999999,-0.784615384615384,-0.769230769230768,
-0.753846153846153,-0.738461538461538,-0.723076923076922,-0.707692307692307,
-0.692307692307692,-0.676923076923076,-0.661538461538461,-0.646153846153846,
-0.63076923076923,-0.615384615384615,-0.6,-0.584615384615384,-0.569230769230769,
-0.553846153846154,-0.538461538461538,-0.523076923076923,-0.507692307692308,
-0.492307692307692,-0.476923076923077,-0.461538461538462,-0.446153846153846,
-0.430769230769231,-0.415384615384615,-0.4,-0.384615384615385,-0.369230769230769,
-0.353846153846154,-0.338461538461538,-0.323076923076923,-0.307692307692308,
-0.292307692307692,-0.276923076923077,-0.261538461538462,-0.246153846153846,
-0.230769230769231,-0.215384615384615,-0.2,-0.184615384615385,-0.169230769230769,
-0.153846153846154,-0.138461538461538,-0.123076923076923,-0.107692307692308,
-0.0923076923076923,-0.0769230769230769,-0.0615384615384615,-0.0461538461538462,
-0.0307692307692308,-0.0153846153846154,0.),.UNSPECIFIED.)
CURVE()
GEOMETRIC_REPRESENTATION_ITEM()
RATIONAL_B_SPLINE_CURVE((1.,1.,1.,1.,1.,1.,1.,1.,1.,1.,1.,1.,1.,1.,1.,1.,
1.,1.,1.,1.,1.,1.,1.,1.,1.,1.,1.,1.,1.,1.,1.,1.,1.,1.,1.,1.,1.,1.,1.,1.,
1.,1.,1.,1.,1.,1.,1.,1.,1.,1.,1.,1.,1.,1.,1.,1.,1.,1.,1.,1.,1.,1.,1.,1.,
1.,1.,1.,1.,1.,1.))
REPRESENTATION_ITEM('')
);
#112=(
BOUNDED_CURVE()
B_SPLINE_CURVE(5,(#28994,#28995,#28996,#28997,#28998,#28999,#29000,#29001,
#29002,#29003,#29004,#29005,#29006,#29007,#29008,#29009,#29010,#29011,#29012,
#29013,#29014,#29015,#29016,#29017,#29018,#29019,#29020,#29021,#29022,#29023,
#29024,#29025,#29026,#29027,#29028,#29029,#29030,#29031,#29032,#29033,#29034,
#29035,#29036,#29037,#29038,#29039,#29040,#29041,#29042,#29043,#29044,#29045,
#29046,#29047,#29048,#29049,#29050,#29051,#29052,#29053,#29054,#29055,#29056,
#29057,#29058,#29059,#29060,#29061,#29062,#29063),.UNSPECIFIED.,.F.,.F.)
B_SPLINE_CURVE_WITH_KNOTS((6,1,1,1,1,1,1,1,1,1,1,1,1,1,1,1,1,1,1,1,1,1,
1,1,1,1,1,1,1,1,1,1,1,1,1,1,1,1,1,1,1,1,1,1,1,1,1,1,1,1,1,1,1,1,1,1,1,1,
1,1,1,1,1,1,1,6),(-1.,-0.984615384615383,-0.969230769230768,-0.953846153846152,
-0.938461538461537,-0.923076923076922,-0.907692307692306,-0.892307692307691,
-0.876923076923076,-0.86153846153846,-0.846153846153845,-0.83076923076923,
-0.815384615384614,-0.799999999999999,-0.784615384615384,-0.769230769230768,
-0.753846153846153,-0.738461538461538,-0.723076923076922,-0.707692307692307,
-0.692307692307692,-0.676923076923076,-0.661538461538461,-0.646153846153846,
-0.63076923076923,-0.615384615384615,-0.6,-0.584615384615384,-0.569230769230769,
-0.553846153846154,-0.538461538461538,-0.523076923076923,-0.507692307692308,
-0.492307692307692,-0.476923076923077,-0.461538461538462,-0.446153846153846,
-0.430769230769231,-0.415384615384615,-0.4,-0.384615384615385,-0.369230769230769,
-0.353846153846154,-0.338461538461538,-0.323076923076923,-0.307692307692308,
-0.292307692307692,-0.276923076923077,-0.261538461538462,-0.246153846153846,
-0.230769230769231,-0.215384615384615,-0.2,-0.184615384615385,-0.169230769230769,
-0.153846153846154,-0.138461538461538,-0.123076923076923,-0.107692307692308,
-0.0923076923076923,-0.0769230769230769,-0.0615384615384615,-0.0461538461538462,
-0.0307692307692308,-0.0153846153846154,0.),.UNSPECIFIED.)
CURVE()
GEOMETRIC_REPRESENTATION_ITEM()
RATIONAL_B_SPLINE_CURVE((1.,1.,1.,1.,1.,1.,1.,1.,1.,1.,1.,1.,1.,1.,1.,1.,
1.,1.,1.,1.,1.,1.,1.,1.,1.,1.,1.,1.,1.,1.,1.,1.,1.,1.,1.,1.,1.,1.,1.,1.,
1.,1.,1.,1.,1.,1.,1.,1.,1.,1.,1.,1.,1.,1.,1.,1.,1.,1.,1.,1.,1.,1.,1.,1.,
1.,1.,1.,1.,1.,1.))
REPRESENTATION_ITEM('')
);
#113=(
BOUNDED_CURVE()
B_SPLINE_CURVE(5,(#29210,#29211,#29212,#29213,#29214,#29215,#29216,#29217,
#29218,#29219,#29220,#29221,#29222,#29223,#29224,#29225,#29226,#29227,#29228,
#29229,#29230,#29231,#29232,#29233,#29234,#29235,#29236,#29237,#29238,#29239,
#29240,#29241,#29242,#29243,#29244,#29245,#29246,#29247,#29248,#29249,#29250,
#29251,#29252,#29253,#29254,#29255,#29256,#29257,#29258,#29259,#29260,#29261,
#29262,#29263,#29264,#29265,#29266,#29267,#29268,#29269,#29270,#29271,#29272,
#29273,#29274,#29275,#29276,#29277,#29278,#29279),.UNSPECIFIED.,.F.,.F.)
B_SPLINE_CURVE_WITH_KNOTS((6,1,1,1,1,1,1,1,1,1,1,1,1,1,1,1,1,1,1,1,1,1,
1,1,1,1,1,1,1,1,1,1,1,1,1,1,1,1,1,1,1,1,1,1,1,1,1,1,1,1,1,1,1,1,1,1,1,1,
1,1,1,1,1,1,1,6),(-1.,-0.984615384615383,-0.969230769230768,-0.953846153846152,
-0.938461538461537,-0.923076923076922,-0.907692307692306,-0.892307692307691,
-0.876923076923076,-0.86153846153846,-0.846153846153845,-0.83076923076923,
-0.815384615384614,-0.799999999999999,-0.784615384615384,-0.769230769230768,
-0.753846153846153,-0.738461538461538,-0.723076923076922,-0.707692307692307,
-0.692307692307692,-0.676923076923076,-0.661538461538461,-0.646153846153846,
-0.63076923076923,-0.615384615384615,-0.6,-0.584615384615384,-0.569230769230769,
-0.553846153846154,-0.538461538461538,-0.523076923076923,-0.507692307692308,
-0.492307692307692,-0.476923076923077,-0.461538461538462,-0.446153846153846,
-0.430769230769231,-0.415384615384615,-0.4,-0.384615384615385,-0.369230769230769,
-0.353846153846154,-0.338461538461538,-0.323076923076923,-0.307692307692308,
-0.292307692307692,-0.276923076923077,-0.261538461538462,-0.246153846153846,
-0.230769230769231,-0.215384615384615,-0.2,-0.184615384615385,-0.169230769230769,
-0.153846153846154,-0.138461538461538,-0.123076923076923,-0.107692307692308,
-0.0923076923076923,-0.0769230769230769,-0.0615384615384615,-0.0461538461538462,
-0.0307692307692308,-0.0153846153846154,0.),.UNSPECIFIED.)
CURVE()
GEOMETRIC_REPRESENTATION_ITEM()
RATIONAL_B_SPLINE_CURVE((1.,1.,1.,1.,1.,1.,1.,1.,1.,1.,1.,1.,1.,1.,1.,1.,
1.,1.,1.,1.,1.,1.,1.,1.,1.,1.,1.,1.,1.,1.,1.,1.,1.,1.,1.,1.,1.,1.,1.,1.,
1.,1.,1.,1.,1.,1.,1.,1.,1.,1.,1.,1.,1.,1.,1.,1.,1.,1.,1.,1.,1.,1.,1.,1.,
1.,1.,1.,1.,1.,1.))
REPRESENTATION_ITEM('')
);
#114=(
BOUNDED_CURVE()
B_SPLINE_CURVE(5,(#29426,#29427,#29428,#29429,#29430,#29431,#29432,#29433,
#29434,#29435,#29436,#29437,#29438,#29439,#29440,#29441,#29442,#29443,#29444,
#29445,#29446,#29447,#29448,#29449,#29450,#29451,#29452,#29453,#29454,#29455,
#29456,#29457,#29458,#29459,#29460,#29461,#29462,#29463,#29464,#29465,#29466,
#29467,#29468,#29469,#29470,#29471,#29472,#29473,#29474,#29475,#29476,#29477,
#29478,#29479,#29480,#29481,#29482,#29483,#29484,#29485,#29486,#29487,#29488,
#29489,#29490,#29491,#29492,#29493,#29494,#29495),.UNSPECIFIED.,.F.,.F.)
B_SPLINE_CURVE_WITH_KNOTS((6,1,1,1,1,1,1,1,1,1,1,1,1,1,1,1,1,1,1,1,1,1,
1,1,1,1,1,1,1,1,1,1,1,1,1,1,1,1,1,1,1,1,1,1,1,1,1,1,1,1,1,1,1,1,1,1,1,1,
1,1,1,1,1,1,1,6),(-1.,-0.984615384615383,-0.969230769230768,-0.953846153846152,
-0.938461538461537,-0.923076923076922,-0.907692307692306,-0.892307692307691,
-0.876923076923076,-0.86153846153846,-0.846153846153845,-0.83076923076923,
-0.815384615384614,-0.799999999999999,-0.784615384615384,-0.769230769230768,
-0.753846153846153,-0.738461538461538,-0.723076923076922,-0.707692307692307,
-0.692307692307692,-0.676923076923076,-0.661538461538461,-0.646153846153846,
-0.63076923076923,-0.615384615384615,-0.6,-0.584615384615384,-0.569230769230769,
-0.553846153846154,-0.538461538461538,-0.523076923076923,-0.507692307692308,
-0.492307692307692,-0.476923076923077,-0.461538461538462,-0.446153846153846,
-0.430769230769231,-0.415384615384615,-0.4,-0.384615384615385,-0.369230769230769,
-0.353846153846154,-0.338461538461538,-0.323076923076923,-0.307692307692308,
-0.292307692307692,-0.276923076923077,-0.261538461538462,-0.246153846153846,
-0.230769230769231,-0.215384615384615,-0.2,-0.184615384615385,-0.169230769230769,
-0.153846153846154,-0.138461538461538,-0.123076923076923,-0.107692307692308,
-0.0923076923076923,-0.0769230769230769,-0.0615384615384615,-0.0461538461538462,
-0.0307692307692308,-0.0153846153846154,0.),.UNSPECIFIED.)
CURVE()
GEOMETRIC_REPRESENTATION_ITEM()
RATIONAL_B_SPLINE_CURVE((1.,1.,1.,1.,1.,1.,1.,1.,1.,1.,1.,1.,1.,1.,1.,1.,
1.,1.,1.,1.,1.,1.,1.,1.,1.,1.,1.,1.,1.,1.,1.,1.,1.,1.,1.,1.,1.,1.,1.,1.,
1.,1.,1.,1.,1.,1.,1.,1.,1.,1.,1.,1.,1.,1.,1.,1.,1.,1.,1.,1.,1.,1.,1.,1.,
1.,1.,1.,1.,1.,1.))
REPRESENTATION_ITEM('')
);
#115=(
BOUNDED_CURVE()
B_SPLINE_CURVE(5,(#29642,#29643,#29644,#29645,#29646,#29647,#29648,#29649,
#29650,#29651,#29652,#29653,#29654,#29655,#29656,#29657,#29658,#29659,#29660,
#29661,#29662,#29663,#29664,#29665,#29666,#29667,#29668,#29669,#29670,#29671,
#29672,#29673,#29674,#29675,#29676,#29677,#29678,#29679,#29680,#29681,#29682,
#29683,#29684,#29685,#29686,#29687,#29688,#29689,#29690,#29691,#29692,#29693,
#29694,#29695,#29696,#29697,#29698,#29699,#29700,#29701,#29702,#29703,#29704,
#29705,#29706,#29707,#29708,#29709,#29710,#29711),.UNSPECIFIED.,.F.,.F.)
B_SPLINE_CURVE_WITH_KNOTS((6,1,1,1,1,1,1,1,1,1,1,1,1,1,1,1,1,1,1,1,1,1,
1,1,1,1,1,1,1,1,1,1,1,1,1,1,1,1,1,1,1,1,1,1,1,1,1,1,1,1,1,1,1,1,1,1,1,1,
1,1,1,1,1,1,1,6),(-1.,-0.984615384615383,-0.969230769230768,-0.953846153846152,
-0.938461538461537,-0.923076923076922,-0.907692307692306,-0.892307692307691,
-0.876923076923076,-0.86153846153846,-0.846153846153845,-0.83076923076923,
-0.815384615384614,-0.799999999999999,-0.784615384615384,-0.769230769230768,
-0.753846153846153,-0.738461538461538,-0.723076923076922,-0.707692307692307,
-0.692307692307692,-0.676923076923076,-0.661538461538461,-0.646153846153846,
-0.63076923076923,-0.615384615384615,-0.6,-0.584615384615384,-0.569230769230769,
-0.553846153846154,-0.538461538461538,-0.523076923076923,-0.507692307692308,
-0.492307692307692,-0.476923076923077,-0.461538461538462,-0.446153846153846,
-0.430769230769231,-0.415384615384615,-0.4,-0.384615384615385,-0.369230769230769,
-0.353846153846154,-0.338461538461538,-0.323076923076923,-0.307692307692308,
-0.292307692307692,-0.276923076923077,-0.261538461538462,-0.246153846153846,
-0.230769230769231,-0.215384615384615,-0.2,-0.184615384615385,-0.169230769230769,
-0.153846153846154,-0.138461538461538,-0.123076923076923,-0.107692307692308,
-0.0923076923076923,-0.0769230769230769,-0.0615384615384615,-0.0461538461538462,
-0.0307692307692308,-0.0153846153846154,0.),.UNSPECIFIED.)
CURVE()
GEOMETRIC_REPRESENTATION_ITEM()
RATIONAL_B_SPLINE_CURVE((1.,1.,1.,1.,1.,1.,1.,1.,1.,1.,1.,1.,1.,1.,1.,1.,
1.,1.,1.,1.,1.,1.,1.,1.,1.,1.,1.,1.,1.,1.,1.,1.,1.,1.,1.,1.,1.,1.,1.,1.,
1.,1.,1.,1.,1.,1.,1.,1.,1.,1.,1.,1.,1.,1.,1.,1.,1.,1.,1.,1.,1.,1.,1.,1.,
1.,1.,1.,1.,1.,1.))
REPRESENTATION_ITEM('')
);
#116=(
BOUNDED_CURVE()
B_SPLINE_CURVE(5,(#29858,#29859,#29860,#29861,#29862,#29863,#29864,#29865,
#29866,#29867,#29868,#29869,#29870,#29871,#29872,#29873,#29874,#29875,#29876,
#29877,#29878,#29879,#29880,#29881,#29882,#29883,#29884,#29885,#29886,#29887,
#29888,#29889,#29890,#29891,#29892,#29893,#29894,#29895,#29896,#29897,#29898,
#29899,#29900,#29901,#29902,#29903,#29904,#29905,#29906,#29907,#29908,#29909,
#29910,#29911,#29912,#29913,#29914,#29915,#29916,#29917,#29918,#29919,#29920,
#29921,#29922,#29923,#29924,#29925,#29926,#29927),.UNSPECIFIED.,.F.,.F.)
B_SPLINE_CURVE_WITH_KNOTS((6,1,1,1,1,1,1,1,1,1,1,1,1,1,1,1,1,1,1,1,1,1,
1,1,1,1,1,1,1,1,1,1,1,1,1,1,1,1,1,1,1,1,1,1,1,1,1,1,1,1,1,1,1,1,1,1,1,1,
1,1,1,1,1,1,1,6),(-1.,-0.984615384615383,-0.969230769230768,-0.953846153846152,
-0.938461538461537,-0.923076923076922,-0.907692307692306,-0.892307692307691,
-0.876923076923076,-0.86153846153846,-0.846153846153845,-0.83076923076923,
-0.815384615384614,-0.799999999999999,-0.784615384615384,-0.769230769230768,
-0.753846153846153,-0.738461538461538,-0.723076923076922,-0.707692307692307,
-0.692307692307692,-0.676923076923076,-0.661538461538461,-0.646153846153846,
-0.63076923076923,-0.615384615384615,-0.6,-0.584615384615384,-0.569230769230769,
-0.553846153846154,-0.538461538461538,-0.523076923076923,-0.507692307692308,
-0.492307692307692,-0.476923076923077,-0.461538461538462,-0.446153846153846,
-0.430769230769231,-0.415384615384615,-0.4,-0.384615384615385,-0.369230769230769,
-0.353846153846154,-0.338461538461538,-0.323076923076923,-0.307692307692308,
-0.292307692307692,-0.276923076923077,-0.261538461538462,-0.246153846153846,
-0.230769230769231,-0.215384615384615,-0.2,-0.184615384615385,-0.169230769230769,
-0.153846153846154,-0.138461538461538,-0.123076923076923,-0.107692307692308,
-0.0923076923076923,-0.0769230769230769,-0.0615384615384615,-0.0461538461538462,
-0.0307692307692308,-0.0153846153846154,0.),.UNSPECIFIED.)
CURVE()
GEOMETRIC_REPRESENTATION_ITEM()
RATIONAL_B_SPLINE_CURVE((1.,1.,1.,1.,1.,1.,1.,1.,1.,1.,1.,1.,1.,1.,1.,1.,
1.,1.,1.,1.,1.,1.,1.,1.,1.,1.,1.,1.,1.,1.,1.,1.,1.,1.,1.,1.,1.,1.,1.,1.,
1.,1.,1.,1.,1.,1.,1.,1.,1.,1.,1.,1.,1.,1.,1.,1.,1.,1.,1.,1.,1.,1.,1.,1.,
1.,1.,1.,1.,1.,1.))
REPRESENTATION_ITEM('')
);
#117=(
BOUNDED_CURVE()
B_SPLINE_CURVE(5,(#30074,#30075,#30076,#30077,#30078,#30079,#30080,#30081,
#30082,#30083,#30084,#30085,#30086,#30087,#30088,#30089,#30090,#30091,#30092,
#30093,#30094,#30095,#30096,#30097,#30098,#30099,#30100,#30101,#30102,#30103,
#30104,#30105,#30106,#30107,#30108,#30109,#30110,#30111,#30112,#30113,#30114,
#30115,#30116,#30117,#30118,#30119,#30120,#30121,#30122,#30123,#30124,#30125,
#30126,#30127,#30128,#30129,#30130,#30131,#30132,#30133,#30134,#30135,#30136,
#30137,#30138,#30139,#30140,#30141,#30142,#30143),.UNSPECIFIED.,.F.,.F.)
B_SPLINE_CURVE_WITH_KNOTS((6,1,1,1,1,1,1,1,1,1,1,1,1,1,1,1,1,1,1,1,1,1,
1,1,1,1,1,1,1,1,1,1,1,1,1,1,1,1,1,1,1,1,1,1,1,1,1,1,1,1,1,1,1,1,1,1,1,1,
1,1,1,1,1,1,1,6),(-1.,-0.984615384615383,-0.969230769230768,-0.953846153846152,
-0.938461538461537,-0.923076923076922,-0.907692307692306,-0.892307692307691,
-0.876923076923076,-0.86153846153846,-0.846153846153845,-0.83076923076923,
-0.815384615384614,-0.799999999999999,-0.784615384615384,-0.769230769230768,
-0.753846153846153,-0.738461538461538,-0.723076923076922,-0.707692307692307,
-0.692307692307692,-0.676923076923076,-0.661538461538461,-0.646153846153846,
-0.63076923076923,-0.615384615384615,-0.6,-0.584615384615384,-0.569230769230769,
-0.553846153846154,-0.538461538461538,-0.523076923076923,-0.507692307692308,
-0.492307692307692,-0.476923076923077,-0.461538461538462,-0.446153846153846,
-0.430769230769231,-0.415384615384615,-0.4,-0.384615384615385,-0.369230769230769,
-0.353846153846154,-0.338461538461538,-0.323076923076923,-0.307692307692308,
-0.292307692307692,-0.276923076923077,-0.261538461538462,-0.246153846153846,
-0.230769230769231,-0.215384615384615,-0.2,-0.184615384615385,-0.169230769230769,
-0.153846153846154,-0.138461538461538,-0.123076923076923,-0.107692307692308,
-0.0923076923076923,-0.0769230769230769,-0.0615384615384615,-0.0461538461538462,
-0.0307692307692308,-0.0153846153846154,0.),.UNSPECIFIED.)
CURVE()
GEOMETRIC_REPRESENTATION_ITEM()
RATIONAL_B_SPLINE_CURVE((1.,1.,1.,1.,1.,1.,1.,1.,1.,1.,1.,1.,1.,1.,1.,1.,
1.,1.,1.,1.,1.,1.,1.,1.,1.,1.,1.,1.,1.,1.,1.,1.,1.,1.,1.,1.,1.,1.,1.,1.,
1.,1.,1.,1.,1.,1.,1.,1.,1.,1.,1.,1.,1.,1.,1.,1.,1.,1.,1.,1.,1.,1.,1.,1.,
1.,1.,1.,1.,1.,1.))
REPRESENTATION_ITEM('')
);
#118=(
BOUNDED_CURVE()
B_SPLINE_CURVE(5,(#30290,#30291,#30292,#30293,#30294,#30295,#30296,#30297,
#30298,#30299,#30300,#30301,#30302,#30303,#30304,#30305,#30306,#30307,#30308,
#30309,#30310,#30311,#30312,#30313,#30314,#30315,#30316,#30317,#30318,#30319,
#30320,#30321,#30322,#30323,#30324,#30325,#30326,#30327,#30328,#30329,#30330,
#30331,#30332,#30333,#30334,#30335,#30336,#30337,#30338,#30339,#30340,#30341,
#30342,#30343,#30344,#30345,#30346,#30347,#30348,#30349,#30350,#30351,#30352,
#30353,#30354,#30355,#30356,#30357,#30358,#30359),.UNSPECIFIED.,.F.,.F.)
B_SPLINE_CURVE_WITH_KNOTS((6,1,1,1,1,1,1,1,1,1,1,1,1,1,1,1,1,1,1,1,1,1,
1,1,1,1,1,1,1,1,1,1,1,1,1,1,1,1,1,1,1,1,1,1,1,1,1,1,1,1,1,1,1,1,1,1,1,1,
1,1,1,1,1,1,1,6),(-1.,-0.984615384615383,-0.969230769230768,-0.953846153846152,
-0.938461538461537,-0.923076923076922,-0.907692307692306,-0.892307692307691,
-0.876923076923076,-0.86153846153846,-0.846153846153845,-0.83076923076923,
-0.815384615384614,-0.799999999999999,-0.784615384615384,-0.769230769230768,
-0.753846153846153,-0.738461538461538,-0.723076923076922,-0.707692307692307,
-0.692307692307692,-0.676923076923076,-0.661538461538461,-0.646153846153846,
-0.63076923076923,-0.615384615384615,-0.6,-0.584615384615384,-0.569230769230769,
-0.553846153846154,-0.538461538461538,-0.523076923076923,-0.507692307692308,
-0.492307692307692,-0.476923076923077,-0.461538461538462,-0.446153846153846,
-0.430769230769231,-0.415384615384615,-0.4,-0.384615384615385,-0.369230769230769,
-0.353846153846154,-0.338461538461538,-0.323076923076923,-0.307692307692308,
-0.292307692307692,-0.276923076923077,-0.261538461538462,-0.246153846153846,
-0.230769230769231,-0.215384615384615,-0.2,-0.184615384615385,-0.169230769230769,
-0.153846153846154,-0.138461538461538,-0.123076923076923,-0.107692307692308,
-0.0923076923076923,-0.0769230769230769,-0.0615384615384615,-0.0461538461538462,
-0.0307692307692308,-0.0153846153846154,0.),.UNSPECIFIED.)
CURVE()
GEOMETRIC_REPRESENTATION_ITEM()
RATIONAL_B_SPLINE_CURVE((1.,1.,1.,1.,1.,1.,1.,1.,1.,1.,1.,1.,1.,1.,1.,1.,
1.,1.,1.,1.,1.,1.,1.,1.,1.,1.,1.,1.,1.,1.,1.,1.,1.,1.,1.,1.,1.,1.,1.,1.,
1.,1.,1.,1.,1.,1.,1.,1.,1.,1.,1.,1.,1.,1.,1.,1.,1.,1.,1.,1.,1.,1.,1.,1.,
1.,1.,1.,1.,1.,1.))
REPRESENTATION_ITEM('')
);
#119=(
BOUNDED_CURVE()
B_SPLINE_CURVE(5,(#30506,#30507,#30508,#30509,#30510,#30511,#30512,#30513,
#30514,#30515,#30516,#30517,#30518,#30519,#30520,#30521,#30522,#30523,#30524,
#30525,#30526,#30527,#30528,#30529,#30530,#30531,#30532,#30533,#30534,#30535,
#30536,#30537,#30538,#30539,#30540,#30541,#30542,#30543,#30544,#30545,#30546,
#30547,#30548,#30549,#30550,#30551,#30552,#30553,#30554,#30555,#30556,#30557,
#30558,#30559,#30560,#30561,#30562,#30563,#30564,#30565,#30566,#30567,#30568,
#30569,#30570,#30571,#30572,#30573,#30574,#30575),.UNSPECIFIED.,.F.,.F.)
B_SPLINE_CURVE_WITH_KNOTS((6,1,1,1,1,1,1,1,1,1,1,1,1,1,1,1,1,1,1,1,1,1,
1,1,1,1,1,1,1,1,1,1,1,1,1,1,1,1,1,1,1,1,1,1,1,1,1,1,1,1,1,1,1,1,1,1,1,1,
1,1,1,1,1,1,1,6),(-1.,-0.984615384615383,-0.969230769230768,-0.953846153846152,
-0.938461538461537,-0.923076923076922,-0.907692307692306,-0.892307692307691,
-0.876923076923076,-0.86153846153846,-0.846153846153845,-0.83076923076923,
-0.815384615384614,-0.799999999999999,-0.784615384615384,-0.769230769230768,
-0.753846153846153,-0.738461538461538,-0.723076923076922,-0.707692307692307,
-0.692307692307692,-0.676923076923076,-0.661538461538461,-0.646153846153846,
-0.63076923076923,-0.615384615384615,-0.6,-0.584615384615384,-0.569230769230769,
-0.553846153846154,-0.538461538461538,-0.523076923076923,-0.507692307692308,
-0.492307692307692,-0.476923076923077,-0.461538461538462,-0.446153846153846,
-0.430769230769231,-0.415384615384615,-0.4,-0.384615384615385,-0.369230769230769,
-0.353846153846154,-0.338461538461538,-0.323076923076923,-0.307692307692308,
-0.292307692307692,-0.276923076923077,-0.261538461538462,-0.246153846153846,
-0.230769230769231,-0.215384615384615,-0.2,-0.184615384615385,-0.169230769230769,
-0.153846153846154,-0.138461538461538,-0.123076923076923,-0.107692307692308,
-0.0923076923076923,-0.0769230769230769,-0.0615384615384615,-0.0461538461538462,
-0.0307692307692308,-0.0153846153846154,0.),.UNSPECIFIED.)
CURVE()
GEOMETRIC_REPRESENTATION_ITEM()
RATIONAL_B_SPLINE_CURVE((1.,1.,1.,1.,1.,1.,1.,1.,1.,1.,1.,1.,1.,1.,1.,1.,
1.,1.,1.,1.,1.,1.,1.,1.,1.,1.,1.,1.,1.,1.,1.,1.,1.,1.,1.,1.,1.,1.,1.,1.,
1.,1.,1.,1.,1.,1.,1.,1.,1.,1.,1.,1.,1.,1.,1.,1.,1.,1.,1.,1.,1.,1.,1.,1.,
1.,1.,1.,1.,1.,1.))
REPRESENTATION_ITEM('')
);
#120=(
BOUNDED_CURVE()
B_SPLINE_CURVE(5,(#30722,#30723,#30724,#30725,#30726,#30727,#30728,#30729,
#30730,#30731,#30732,#30733,#30734,#30735,#30736,#30737,#30738,#30739,#30740,
#30741,#30742,#30743,#30744,#30745,#30746,#30747,#30748,#30749,#30750,#30751,
#30752,#30753,#30754,#30755,#30756,#30757,#30758,#30759,#30760,#30761,#30762,
#30763,#30764,#30765,#30766,#30767,#30768,#30769,#30770,#30771,#30772,#30773,
#30774,#30775,#30776,#30777,#30778,#30779,#30780,#30781,#30782,#30783,#30784,
#30785,#30786,#30787,#30788,#30789,#30790,#30791),.UNSPECIFIED.,.F.,.F.)
B_SPLINE_CURVE_WITH_KNOTS((6,1,1,1,1,1,1,1,1,1,1,1,1,1,1,1,1,1,1,1,1,1,
1,1,1,1,1,1,1,1,1,1,1,1,1,1,1,1,1,1,1,1,1,1,1,1,1,1,1,1,1,1,1,1,1,1,1,1,
1,1,1,1,1,1,1,6),(-1.,-0.984615384615383,-0.969230769230768,-0.953846153846152,
-0.938461538461537,-0.923076923076922,-0.907692307692306,-0.892307692307691,
-0.876923076923076,-0.86153846153846,-0.846153846153845,-0.83076923076923,
-0.815384615384614,-0.799999999999999,-0.784615384615384,-0.769230769230768,
-0.753846153846153,-0.738461538461538,-0.723076923076922,-0.707692307692307,
-0.692307692307692,-0.676923076923076,-0.661538461538461,-0.646153846153846,
-0.63076923076923,-0.615384615384615,-0.6,-0.584615384615384,-0.569230769230769,
-0.553846153846154,-0.538461538461538,-0.523076923076923,-0.507692307692308,
-0.492307692307692,-0.476923076923077,-0.461538461538462,-0.446153846153846,
-0.430769230769231,-0.415384615384615,-0.4,-0.384615384615385,-0.369230769230769,
-0.353846153846154,-0.338461538461538,-0.323076923076923,-0.307692307692308,
-0.292307692307692,-0.276923076923077,-0.261538461538462,-0.246153846153846,
-0.230769230769231,-0.215384615384615,-0.2,-0.184615384615385,-0.169230769230769,
-0.153846153846154,-0.138461538461538,-0.123076923076923,-0.107692307692308,
-0.0923076923076923,-0.0769230769230769,-0.0615384615384615,-0.0461538461538462,
-0.0307692307692308,-0.0153846153846154,0.),.UNSPECIFIED.)
CURVE()
GEOMETRIC_REPRESENTATION_ITEM()
RATIONAL_B_SPLINE_CURVE((1.,1.,1.,1.,1.,1.,1.,1.,1.,1.,1.,1.,1.,1.,1.,1.,
1.,1.,1.,1.,1.,1.,1.,1.,1.,1.,1.,1.,1.,1.,1.,1.,1.,1.,1.,1.,1.,1.,1.,1.,
1.,1.,1.,1.,1.,1.,1.,1.,1.,1.,1.,1.,1.,1.,1.,1.,1.,1.,1.,1.,1.,1.,1.,1.,
1.,1.,1.,1.,1.,1.))
REPRESENTATION_ITEM('')
);
#121=(
BOUNDED_CURVE()
B_SPLINE_CURVE(5,(#30938,#30939,#30940,#30941,#30942,#30943,#30944,#30945,
#30946,#30947,#30948,#30949,#30950,#30951,#30952,#30953,#30954,#30955,#30956,
#30957,#30958,#30959,#30960,#30961,#30962,#30963,#30964,#30965,#30966,#30967,
#30968,#30969,#30970,#30971,#30972,#30973,#30974,#30975,#30976,#30977,#30978,
#30979,#30980,#30981,#30982,#30983,#30984,#30985,#30986,#30987,#30988,#30989,
#30990,#30991,#30992,#30993,#30994,#30995,#30996,#30997,#30998,#30999,#31000,
#31001,#31002,#31003,#31004,#31005,#31006,#31007),.UNSPECIFIED.,.F.,.F.)
B_SPLINE_CURVE_WITH_KNOTS((6,1,1,1,1,1,1,1,1,1,1,1,1,1,1,1,1,1,1,1,1,1,
1,1,1,1,1,1,1,1,1,1,1,1,1,1,1,1,1,1,1,1,1,1,1,1,1,1,1,1,1,1,1,1,1,1,1,1,
1,1,1,1,1,1,1,6),(-1.,-0.984615384615383,-0.969230769230768,-0.953846153846152,
-0.938461538461537,-0.923076923076922,-0.907692307692306,-0.892307692307691,
-0.876923076923076,-0.86153846153846,-0.846153846153845,-0.83076923076923,
-0.815384615384614,-0.799999999999999,-0.784615384615384,-0.769230769230768,
-0.753846153846153,-0.738461538461538,-0.723076923076922,-0.707692307692307,
-0.692307692307692,-0.676923076923076,-0.661538461538461,-0.646153846153846,
-0.63076923076923,-0.615384615384615,-0.6,-0.584615384615384,-0.569230769230769,
-0.553846153846154,-0.538461538461538,-0.523076923076923,-0.507692307692308,
-0.492307692307692,-0.476923076923077,-0.461538461538462,-0.446153846153846,
-0.430769230769231,-0.415384615384615,-0.4,-0.384615384615385,-0.369230769230769,
-0.353846153846154,-0.338461538461538,-0.323076923076923,-0.307692307692308,
-0.292307692307692,-0.276923076923077,-0.261538461538462,-0.246153846153846,
-0.230769230769231,-0.215384615384615,-0.2,-0.184615384615385,-0.169230769230769,
-0.153846153846154,-0.138461538461538,-0.123076923076923,-0.107692307692308,
-0.0923076923076923,-0.0769230769230769,-0.0615384615384615,-0.0461538461538462,
-0.0307692307692308,-0.0153846153846154,0.),.UNSPECIFIED.)
CURVE()
GEOMETRIC_REPRESENTATION_ITEM()
RATIONAL_B_SPLINE_CURVE((1.,1.,1.,1.,1.,1.,1.,1.,1.,1.,1.,1.,1.,1.,1.,1.,
1.,1.,1.,1.,1.,1.,1.,1.,1.,1.,1.,1.,1.,1.,1.,1.,1.,1.,1.,1.,1.,1.,1.,1.,
1.,1.,1.,1.,1.,1.,1.,1.,1.,1.,1.,1.,1.,1.,1.,1.,1.,1.,1.,1.,1.,1.,1.,1.,
1.,1.,1.,1.,1.,1.))
REPRESENTATION_ITEM('')
);
#122=(
BOUNDED_CURVE()
B_SPLINE_CURVE(5,(#31154,#31155,#31156,#31157,#31158,#31159,#31160,#31161,
#31162,#31163,#31164,#31165,#31166,#31167,#31168,#31169,#31170,#31171,#31172,
#31173,#31174,#31175,#31176,#31177,#31178,#31179,#31180,#31181,#31182,#31183,
#31184,#31185,#31186,#31187,#31188,#31189,#31190,#31191,#31192,#31193,#31194,
#31195,#31196,#31197,#31198,#31199,#31200,#31201,#31202,#31203,#31204,#31205,
#31206,#31207,#31208,#31209,#31210,#31211,#31212,#31213,#31214,#31215,#31216,
#31217,#31218,#31219,#31220,#31221,#31222,#31223),.UNSPECIFIED.,.F.,.F.)
B_SPLINE_CURVE_WITH_KNOTS((6,1,1,1,1,1,1,1,1,1,1,1,1,1,1,1,1,1,1,1,1,1,
1,1,1,1,1,1,1,1,1,1,1,1,1,1,1,1,1,1,1,1,1,1,1,1,1,1,1,1,1,1,1,1,1,1,1,1,
1,1,1,1,1,1,1,6),(-1.,-0.984615384615383,-0.969230769230768,-0.953846153846152,
-0.938461538461537,-0.923076923076922,-0.907692307692306,-0.892307692307691,
-0.876923076923076,-0.86153846153846,-0.846153846153845,-0.83076923076923,
-0.815384615384614,-0.799999999999999,-0.784615384615384,-0.769230769230768,
-0.753846153846153,-0.738461538461538,-0.723076923076922,-0.707692307692307,
-0.692307692307692,-0.676923076923076,-0.661538461538461,-0.646153846153846,
-0.63076923076923,-0.615384615384615,-0.6,-0.584615384615384,-0.569230769230769,
-0.553846153846154,-0.538461538461538,-0.523076923076923,-0.507692307692308,
-0.492307692307692,-0.476923076923077,-0.461538461538462,-0.446153846153846,
-0.430769230769231,-0.415384615384615,-0.4,-0.384615384615385,-0.369230769230769,
-0.353846153846154,-0.338461538461538,-0.323076923076923,-0.307692307692308,
-0.292307692307692,-0.276923076923077,-0.261538461538462,-0.246153846153846,
-0.230769230769231,-0.215384615384615,-0.2,-0.184615384615385,-0.169230769230769,
-0.153846153846154,-0.138461538461538,-0.123076923076923,-0.107692307692308,
-0.0923076923076923,-0.0769230769230769,-0.0615384615384615,-0.0461538461538462,
-0.0307692307692308,-0.0153846153846154,0.),.UNSPECIFIED.)
CURVE()
GEOMETRIC_REPRESENTATION_ITEM()
RATIONAL_B_SPLINE_CURVE((1.,1.,1.,1.,1.,1.,1.,1.,1.,1.,1.,1.,1.,1.,1.,1.,
1.,1.,1.,1.,1.,1.,1.,1.,1.,1.,1.,1.,1.,1.,1.,1.,1.,1.,1.,1.,1.,1.,1.,1.,
1.,1.,1.,1.,1.,1.,1.,1.,1.,1.,1.,1.,1.,1.,1.,1.,1.,1.,1.,1.,1.,1.,1.,1.,
1.,1.,1.,1.,1.,1.))
REPRESENTATION_ITEM('')
);
#123=(
BOUNDED_CURVE()
B_SPLINE_CURVE(5,(#31370,#31371,#31372,#31373,#31374,#31375,#31376,#31377,
#31378,#31379,#31380,#31381,#31382,#31383,#31384,#31385,#31386,#31387,#31388,
#31389,#31390,#31391,#31392,#31393,#31394,#31395,#31396,#31397,#31398,#31399,
#31400,#31401,#31402,#31403,#31404,#31405,#31406,#31407,#31408,#31409,#31410,
#31411,#31412,#31413,#31414,#31415,#31416,#31417,#31418,#31419,#31420,#31421,
#31422,#31423,#31424,#31425,#31426,#31427,#31428,#31429,#31430,#31431,#31432,
#31433,#31434,#31435,#31436,#31437,#31438,#31439),.UNSPECIFIED.,.F.,.F.)
B_SPLINE_CURVE_WITH_KNOTS((6,1,1,1,1,1,1,1,1,1,1,1,1,1,1,1,1,1,1,1,1,1,
1,1,1,1,1,1,1,1,1,1,1,1,1,1,1,1,1,1,1,1,1,1,1,1,1,1,1,1,1,1,1,1,1,1,1,1,
1,1,1,1,1,1,1,6),(-1.,-0.984615384615383,-0.969230769230768,-0.953846153846152,
-0.938461538461537,-0.923076923076922,-0.907692307692306,-0.892307692307691,
-0.876923076923076,-0.86153846153846,-0.846153846153845,-0.83076923076923,
-0.815384615384614,-0.799999999999999,-0.784615384615384,-0.769230769230768,
-0.753846153846153,-0.738461538461538,-0.723076923076922,-0.707692307692307,
-0.692307692307692,-0.676923076923076,-0.661538461538461,-0.646153846153846,
-0.63076923076923,-0.615384615384615,-0.6,-0.584615384615384,-0.569230769230769,
-0.553846153846154,-0.538461538461538,-0.523076923076923,-0.507692307692308,
-0.492307692307692,-0.476923076923077,-0.461538461538462,-0.446153846153846,
-0.430769230769231,-0.415384615384615,-0.4,-0.384615384615385,-0.369230769230769,
-0.353846153846154,-0.338461538461538,-0.323076923076923,-0.307692307692308,
-0.292307692307692,-0.276923076923077,-0.261538461538462,-0.246153846153846,
-0.230769230769231,-0.215384615384615,-0.2,-0.184615384615385,-0.169230769230769,
-0.153846153846154,-0.138461538461538,-0.123076923076923,-0.107692307692308,
-0.0923076923076923,-0.0769230769230769,-0.0615384615384615,-0.0461538461538462,
-0.0307692307692308,-0.0153846153846154,0.),.UNSPECIFIED.)
CURVE()
GEOMETRIC_REPRESENTATION_ITEM()
RATIONAL_B_SPLINE_CURVE((1.,1.,1.,1.,1.,1.,1.,1.,1.,1.,1.,1.,1.,1.,1.,1.,
1.,1.,1.,1.,1.,1.,1.,1.,1.,1.,1.,1.,1.,1.,1.,1.,1.,1.,1.,1.,1.,1.,1.,1.,
1.,1.,1.,1.,1.,1.,1.,1.,1.,1.,1.,1.,1.,1.,1.,1.,1.,1.,1.,1.,1.,1.,1.,1.,
1.,1.,1.,1.,1.,1.))
REPRESENTATION_ITEM('')
);
#124=(
BOUNDED_CURVE()
B_SPLINE_CURVE(5,(#31586,#31587,#31588,#31589,#31590,#31591,#31592,#31593,
#31594,#31595,#31596,#31597,#31598,#31599,#31600,#31601,#31602,#31603,#31604,
#31605,#31606,#31607,#31608,#31609,#31610,#31611,#31612,#31613,#31614,#31615,
#31616,#31617,#31618,#31619,#31620,#31621,#31622,#31623,#31624,#31625,#31626,
#31627,#31628,#31629,#31630,#31631,#31632,#31633,#31634,#31635,#31636,#31637,
#31638,#31639,#31640,#31641,#31642,#31643,#31644,#31645,#31646,#31647,#31648,
#31649,#31650,#31651,#31652,#31653,#31654,#31655),.UNSPECIFIED.,.F.,.F.)
B_SPLINE_CURVE_WITH_KNOTS((6,1,1,1,1,1,1,1,1,1,1,1,1,1,1,1,1,1,1,1,1,1,
1,1,1,1,1,1,1,1,1,1,1,1,1,1,1,1,1,1,1,1,1,1,1,1,1,1,1,1,1,1,1,1,1,1,1,1,
1,1,1,1,1,1,1,6),(-1.,-0.984615384615383,-0.969230769230768,-0.953846153846152,
-0.938461538461537,-0.923076923076922,-0.907692307692306,-0.892307692307691,
-0.876923076923076,-0.86153846153846,-0.846153846153845,-0.83076923076923,
-0.815384615384614,-0.799999999999999,-0.784615384615384,-0.769230769230768,
-0.753846153846153,-0.738461538461538,-0.723076923076922,-0.707692307692307,
-0.692307692307692,-0.676923076923076,-0.661538461538461,-0.646153846153846,
-0.63076923076923,-0.615384615384615,-0.6,-0.584615384615384,-0.569230769230769,
-0.553846153846154,-0.538461538461538,-0.523076923076923,-0.507692307692308,
-0.492307692307692,-0.476923076923077,-0.461538461538462,-0.446153846153846,
-0.430769230769231,-0.415384615384615,-0.4,-0.384615384615385,-0.369230769230769,
-0.353846153846154,-0.338461538461538,-0.323076923076923,-0.307692307692308,
-0.292307692307692,-0.276923076923077,-0.261538461538462,-0.246153846153846,
-0.230769230769231,-0.215384615384615,-0.2,-0.184615384615385,-0.169230769230769,
-0.153846153846154,-0.138461538461538,-0.123076923076923,-0.107692307692308,
-0.0923076923076923,-0.0769230769230769,-0.0615384615384615,-0.0461538461538462,
-0.0307692307692308,-0.0153846153846154,0.),.UNSPECIFIED.)
CURVE()
GEOMETRIC_REPRESENTATION_ITEM()
RATIONAL_B_SPLINE_CURVE((1.,1.,1.,1.,1.,1.,1.,1.,1.,1.,1.,1.,1.,1.,1.,1.,
1.,1.,1.,1.,1.,1.,1.,1.,1.,1.,1.,1.,1.,1.,1.,1.,1.,1.,1.,1.,1.,1.,1.,1.,
1.,1.,1.,1.,1.,1.,1.,1.,1.,1.,1.,1.,1.,1.,1.,1.,1.,1.,1.,1.,1.,1.,1.,1.,
1.,1.,1.,1.,1.,1.))
REPRESENTATION_ITEM('')
);
#125=(
BOUNDED_CURVE()
B_SPLINE_CURVE(5,(#31802,#31803,#31804,#31805,#31806,#31807,#31808,#31809,
#31810,#31811,#31812,#31813,#31814,#31815,#31816,#31817,#31818,#31819,#31820,
#31821,#31822,#31823,#31824,#31825,#31826,#31827,#31828,#31829,#31830,#31831,
#31832,#31833,#31834,#31835,#31836,#31837,#31838,#31839,#31840,#31841,#31842,
#31843,#31844,#31845,#31846,#31847,#31848,#31849,#31850,#31851,#31852,#31853,
#31854,#31855,#31856,#31857,#31858,#31859,#31860,#31861,#31862,#31863,#31864,
#31865,#31866,#31867,#31868,#31869,#31870,#31871),.UNSPECIFIED.,.F.,.F.)
B_SPLINE_CURVE_WITH_KNOTS((6,1,1,1,1,1,1,1,1,1,1,1,1,1,1,1,1,1,1,1,1,1,
1,1,1,1,1,1,1,1,1,1,1,1,1,1,1,1,1,1,1,1,1,1,1,1,1,1,1,1,1,1,1,1,1,1,1,1,
1,1,1,1,1,1,1,6),(-1.,-0.984615384615383,-0.969230769230768,-0.953846153846152,
-0.938461538461537,-0.923076923076922,-0.907692307692306,-0.892307692307691,
-0.876923076923076,-0.86153846153846,-0.846153846153845,-0.83076923076923,
-0.815384615384614,-0.799999999999999,-0.784615384615384,-0.769230769230768,
-0.753846153846153,-0.738461538461538,-0.723076923076922,-0.707692307692307,
-0.692307692307692,-0.676923076923076,-0.661538461538461,-0.646153846153846,
-0.63076923076923,-0.615384615384615,-0.6,-0.584615384615384,-0.569230769230769,
-0.553846153846154,-0.538461538461538,-0.523076923076923,-0.507692307692308,
-0.492307692307692,-0.476923076923077,-0.461538461538462,-0.446153846153846,
-0.430769230769231,-0.415384615384615,-0.4,-0.384615384615385,-0.369230769230769,
-0.353846153846154,-0.338461538461538,-0.323076923076923,-0.307692307692308,
-0.292307692307692,-0.276923076923077,-0.261538461538462,-0.246153846153846,
-0.230769230769231,-0.215384615384615,-0.2,-0.184615384615385,-0.169230769230769,
-0.153846153846154,-0.138461538461538,-0.123076923076923,-0.107692307692308,
-0.0923076923076923,-0.0769230769230769,-0.0615384615384615,-0.0461538461538462,
-0.0307692307692308,-0.0153846153846154,0.),.UNSPECIFIED.)
CURVE()
GEOMETRIC_REPRESENTATION_ITEM()
RATIONAL_B_SPLINE_CURVE((1.,1.,1.,1.,1.,1.,1.,1.,1.,1.,1.,1.,1.,1.,1.,1.,
1.,1.,1.,1.,1.,1.,1.,1.,1.,1.,1.,1.,1.,1.,1.,1.,1.,1.,1.,1.,1.,1.,1.,1.,
1.,1.,1.,1.,1.,1.,1.,1.,1.,1.,1.,1.,1.,1.,1.,1.,1.,1.,1.,1.,1.,1.,1.,1.,
1.,1.,1.,1.,1.,1.))
REPRESENTATION_ITEM('')
);
#126=(
BOUNDED_CURVE()
B_SPLINE_CURVE(5,(#32018,#32019,#32020,#32021,#32022,#32023,#32024,#32025,
#32026,#32027,#32028,#32029,#32030,#32031,#32032,#32033,#32034,#32035,#32036,
#32037,#32038,#32039,#32040,#32041,#32042,#32043,#32044,#32045,#32046,#32047,
#32048,#32049,#32050,#32051,#32052,#32053,#32054,#32055,#32056,#32057,#32058,
#32059,#32060,#32061,#32062,#32063,#32064,#32065,#32066,#32067,#32068,#32069,
#32070,#32071,#32072,#32073,#32074,#32075,#32076,#32077,#32078,#32079,#32080,
#32081,#32082,#32083,#32084,#32085,#32086,#32087),.UNSPECIFIED.,.F.,.F.)
B_SPLINE_CURVE_WITH_KNOTS((6,1,1,1,1,1,1,1,1,1,1,1,1,1,1,1,1,1,1,1,1,1,
1,1,1,1,1,1,1,1,1,1,1,1,1,1,1,1,1,1,1,1,1,1,1,1,1,1,1,1,1,1,1,1,1,1,1,1,
1,1,1,1,1,1,1,6),(-1.,-0.984615384615383,-0.969230769230768,-0.953846153846152,
-0.938461538461537,-0.923076923076922,-0.907692307692306,-0.892307692307691,
-0.876923076923076,-0.86153846153846,-0.846153846153845,-0.83076923076923,
-0.815384615384614,-0.799999999999999,-0.784615384615384,-0.769230769230768,
-0.753846153846153,-0.738461538461538,-0.723076923076922,-0.707692307692307,
-0.692307692307692,-0.676923076923076,-0.661538461538461,-0.646153846153846,
-0.63076923076923,-0.615384615384615,-0.6,-0.584615384615384,-0.569230769230769,
-0.553846153846154,-0.538461538461538,-0.523076923076923,-0.507692307692308,
-0.492307692307692,-0.476923076923077,-0.461538461538462,-0.446153846153846,
-0.430769230769231,-0.415384615384615,-0.4,-0.384615384615385,-0.369230769230769,
-0.353846153846154,-0.338461538461538,-0.323076923076923,-0.307692307692308,
-0.292307692307692,-0.276923076923077,-0.261538461538462,-0.246153846153846,
-0.230769230769231,-0.215384615384615,-0.2,-0.184615384615385,-0.169230769230769,
-0.153846153846154,-0.138461538461538,-0.123076923076923,-0.107692307692308,
-0.0923076923076923,-0.0769230769230769,-0.0615384615384615,-0.0461538461538462,
-0.0307692307692308,-0.0153846153846154,0.),.UNSPECIFIED.)
CURVE()
GEOMETRIC_REPRESENTATION_ITEM()
RATIONAL_B_SPLINE_CURVE((1.,1.,1.,1.,1.,1.,1.,1.,1.,1.,1.,1.,1.,1.,1.,1.,
1.,1.,1.,1.,1.,1.,1.,1.,1.,1.,1.,1.,1.,1.,1.,1.,1.,1.,1.,1.,1.,1.,1.,1.,
1.,1.,1.,1.,1.,1.,1.,1.,1.,1.,1.,1.,1.,1.,1.,1.,1.,1.,1.,1.,1.,1.,1.,1.,
1.,1.,1.,1.,1.,1.))
REPRESENTATION_ITEM('')
);
#127=(
BOUNDED_CURVE()
B_SPLINE_CURVE(5,(#32234,#32235,#32236,#32237,#32238,#32239,#32240,#32241,
#32242,#32243,#32244,#32245,#32246,#32247,#32248,#32249,#32250,#32251,#32252,
#32253,#32254,#32255,#32256,#32257,#32258,#32259,#32260,#32261,#32262,#32263,
#32264,#32265,#32266,#32267,#32268,#32269,#32270,#32271,#32272,#32273,#32274,
#32275,#32276,#32277,#32278,#32279,#32280,#32281,#32282,#32283,#32284,#32285,
#32286,#32287,#32288,#32289,#32290,#32291,#32292,#32293,#32294,#32295,#32296,
#32297,#32298,#32299,#32300,#32301,#32302,#32303),.UNSPECIFIED.,.F.,.F.)
B_SPLINE_CURVE_WITH_KNOTS((6,1,1,1,1,1,1,1,1,1,1,1,1,1,1,1,1,1,1,1,1,1,
1,1,1,1,1,1,1,1,1,1,1,1,1,1,1,1,1,1,1,1,1,1,1,1,1,1,1,1,1,1,1,1,1,1,1,1,
1,1,1,1,1,1,1,6),(-1.,-0.984615384615383,-0.969230769230768,-0.953846153846152,
-0.938461538461537,-0.923076923076922,-0.907692307692306,-0.892307692307691,
-0.876923076923076,-0.86153846153846,-0.846153846153845,-0.83076923076923,
-0.815384615384614,-0.799999999999999,-0.784615384615384,-0.769230769230768,
-0.753846153846153,-0.738461538461538,-0.723076923076922,-0.707692307692307,
-0.692307692307692,-0.676923076923076,-0.661538461538461,-0.646153846153846,
-0.63076923076923,-0.615384615384615,-0.6,-0.584615384615384,-0.569230769230769,
-0.553846153846154,-0.538461538461538,-0.523076923076923,-0.507692307692308,
-0.492307692307692,-0.476923076923077,-0.461538461538462,-0.446153846153846,
-0.430769230769231,-0.415384615384615,-0.4,-0.384615384615385,-0.369230769230769,
-0.353846153846154,-0.338461538461538,-0.323076923076923,-0.307692307692308,
-0.292307692307692,-0.276923076923077,-0.261538461538462,-0.246153846153846,
-0.230769230769231,-0.215384615384615,-0.2,-0.184615384615385,-0.169230769230769,
-0.153846153846154,-0.138461538461538,-0.123076923076923,-0.107692307692308,
-0.0923076923076923,-0.0769230769230769,-0.0615384615384615,-0.0461538461538462,
-0.0307692307692308,-0.0153846153846154,0.),.UNSPECIFIED.)
CURVE()
GEOMETRIC_REPRESENTATION_ITEM()
RATIONAL_B_SPLINE_CURVE((1.,1.,1.,1.,1.,1.,1.,1.,1.,1.,1.,1.,1.,1.,1.,1.,
1.,1.,1.,1.,1.,1.,1.,1.,1.,1.,1.,1.,1.,1.,1.,1.,1.,1.,1.,1.,1.,1.,1.,1.,
1.,1.,1.,1.,1.,1.,1.,1.,1.,1.,1.,1.,1.,1.,1.,1.,1.,1.,1.,1.,1.,1.,1.,1.,
1.,1.,1.,1.,1.,1.))
REPRESENTATION_ITEM('')
);
#128=(
BOUNDED_CURVE()
B_SPLINE_CURVE(5,(#32450,#32451,#32452,#32453,#32454,#32455,#32456,#32457,
#32458,#32459,#32460,#32461,#32462,#32463,#32464,#32465,#32466,#32467,#32468,
#32469,#32470,#32471,#32472,#32473,#32474,#32475,#32476,#32477,#32478,#32479,
#32480,#32481,#32482,#32483,#32484,#32485,#32486,#32487,#32488,#32489,#32490,
#32491,#32492,#32493,#32494,#32495,#32496,#32497,#32498,#32499,#32500,#32501,
#32502,#32503,#32504,#32505,#32506,#32507,#32508,#32509,#32510,#32511,#32512,
#32513,#32514,#32515,#32516,#32517,#32518,#32519),.UNSPECIFIED.,.F.,.F.)
B_SPLINE_CURVE_WITH_KNOTS((6,1,1,1,1,1,1,1,1,1,1,1,1,1,1,1,1,1,1,1,1,1,
1,1,1,1,1,1,1,1,1,1,1,1,1,1,1,1,1,1,1,1,1,1,1,1,1,1,1,1,1,1,1,1,1,1,1,1,
1,1,1,1,1,1,1,6),(-1.,-0.984615384615383,-0.969230769230768,-0.953846153846152,
-0.938461538461537,-0.923076923076922,-0.907692307692306,-0.892307692307691,
-0.876923076923076,-0.86153846153846,-0.846153846153845,-0.83076923076923,
-0.815384615384614,-0.799999999999999,-0.784615384615384,-0.769230769230768,
-0.753846153846153,-0.738461538461538,-0.723076923076922,-0.707692307692307,
-0.692307692307692,-0.676923076923076,-0.661538461538461,-0.646153846153846,
-0.63076923076923,-0.615384615384615,-0.6,-0.584615384615384,-0.569230769230769,
-0.553846153846154,-0.538461538461538,-0.523076923076923,-0.507692307692308,
-0.492307692307692,-0.476923076923077,-0.461538461538462,-0.446153846153846,
-0.430769230769231,-0.415384615384615,-0.4,-0.384615384615385,-0.369230769230769,
-0.353846153846154,-0.338461538461538,-0.323076923076923,-0.307692307692308,
-0.292307692307692,-0.276923076923077,-0.261538461538462,-0.246153846153846,
-0.230769230769231,-0.215384615384615,-0.2,-0.184615384615385,-0.169230769230769,
-0.153846153846154,-0.138461538461538,-0.123076923076923,-0.107692307692308,
-0.0923076923076923,-0.0769230769230769,-0.0615384615384615,-0.0461538461538462,
-0.0307692307692308,-0.0153846153846154,0.),.UNSPECIFIED.)
CURVE()
GEOMETRIC_REPRESENTATION_ITEM()
RATIONAL_B_SPLINE_CURVE((1.,1.,1.,1.,1.,1.,1.,1.,1.,1.,1.,1.,1.,1.,1.,1.,
1.,1.,1.,1.,1.,1.,1.,1.,1.,1.,1.,1.,1.,1.,1.,1.,1.,1.,1.,1.,1.,1.,1.,1.,
1.,1.,1.,1.,1.,1.,1.,1.,1.,1.,1.,1.,1.,1.,1.,1.,1.,1.,1.,1.,1.,1.,1.,1.,
1.,1.,1.,1.,1.,1.))
REPRESENTATION_ITEM('')
);
#129=(
BOUNDED_CURVE()
B_SPLINE_CURVE(5,(#32666,#32667,#32668,#32669,#32670,#32671,#32672,#32673,
#32674,#32675,#32676,#32677,#32678,#32679,#32680,#32681,#32682,#32683,#32684,
#32685,#32686,#32687,#32688,#32689,#32690,#32691,#32692,#32693,#32694,#32695,
#32696,#32697,#32698,#32699,#32700,#32701,#32702,#32703,#32704,#32705,#32706,
#32707,#32708,#32709,#32710,#32711,#32712,#32713,#32714,#32715,#32716,#32717,
#32718,#32719,#32720,#32721,#32722,#32723,#32724,#32725,#32726,#32727,#32728,
#32729,#32730,#32731,#32732,#32733,#32734,#32735),.UNSPECIFIED.,.F.,.F.)
B_SPLINE_CURVE_WITH_KNOTS((6,1,1,1,1,1,1,1,1,1,1,1,1,1,1,1,1,1,1,1,1,1,
1,1,1,1,1,1,1,1,1,1,1,1,1,1,1,1,1,1,1,1,1,1,1,1,1,1,1,1,1,1,1,1,1,1,1,1,
1,1,1,1,1,1,1,6),(-1.,-0.984615384615383,-0.969230769230768,-0.953846153846152,
-0.938461538461537,-0.923076923076922,-0.907692307692306,-0.892307692307691,
-0.876923076923076,-0.86153846153846,-0.846153846153845,-0.83076923076923,
-0.815384615384614,-0.799999999999999,-0.784615384615384,-0.769230769230768,
-0.753846153846153,-0.738461538461538,-0.723076923076922,-0.707692307692307,
-0.692307692307692,-0.676923076923076,-0.661538461538461,-0.646153846153846,
-0.63076923076923,-0.615384615384615,-0.6,-0.584615384615384,-0.569230769230769,
-0.553846153846154,-0.538461538461538,-0.523076923076923,-0.507692307692308,
-0.492307692307692,-0.476923076923077,-0.461538461538462,-0.446153846153846,
-0.430769230769231,-0.415384615384615,-0.4,-0.384615384615385,-0.369230769230769,
-0.353846153846154,-0.338461538461538,-0.323076923076923,-0.307692307692308,
-0.292307692307692,-0.276923076923077,-0.261538461538462,-0.246153846153846,
-0.230769230769231,-0.215384615384615,-0.2,-0.184615384615385,-0.169230769230769,
-0.153846153846154,-0.138461538461538,-0.123076923076923,-0.107692307692308,
-0.0923076923076923,-0.0769230769230769,-0.0615384615384615,-0.0461538461538462,
-0.0307692307692308,-0.0153846153846154,0.),.UNSPECIFIED.)
CURVE()
GEOMETRIC_REPRESENTATION_ITEM()
RATIONAL_B_SPLINE_CURVE((1.,1.,1.,1.,1.,1.,1.,1.,1.,1.,1.,1.,1.,1.,1.,1.,
1.,1.,1.,1.,1.,1.,1.,1.,1.,1.,1.,1.,1.,1.,1.,1.,1.,1.,1.,1.,1.,1.,1.,1.,
1.,1.,1.,1.,1.,1.,1.,1.,1.,1.,1.,1.,1.,1.,1.,1.,1.,1.,1.,1.,1.,1.,1.,1.,
1.,1.,1.,1.,1.,1.))
REPRESENTATION_ITEM('')
);
#130=(
BOUNDED_CURVE()
B_SPLINE_CURVE(5,(#32882,#32883,#32884,#32885,#32886,#32887,#32888,#32889,
#32890,#32891,#32892,#32893,#32894,#32895,#32896,#32897,#32898,#32899,#32900,
#32901,#32902,#32903,#32904,#32905,#32906,#32907,#32908,#32909,#32910,#32911,
#32912,#32913,#32914,#32915,#32916,#32917,#32918,#32919,#32920,#32921,#32922,
#32923,#32924,#32925,#32926,#32927,#32928,#32929,#32930,#32931,#32932,#32933,
#32934,#32935,#32936,#32937,#32938,#32939,#32940,#32941,#32942,#32943,#32944,
#32945,#32946,#32947,#32948,#32949,#32950,#32951),.UNSPECIFIED.,.F.,.F.)
B_SPLINE_CURVE_WITH_KNOTS((6,1,1,1,1,1,1,1,1,1,1,1,1,1,1,1,1,1,1,1,1,1,
1,1,1,1,1,1,1,1,1,1,1,1,1,1,1,1,1,1,1,1,1,1,1,1,1,1,1,1,1,1,1,1,1,1,1,1,
1,1,1,1,1,1,1,6),(-1.,-0.984615384615383,-0.969230769230768,-0.953846153846152,
-0.938461538461537,-0.923076923076922,-0.907692307692306,-0.892307692307691,
-0.876923076923076,-0.86153846153846,-0.846153846153845,-0.83076923076923,
-0.815384615384614,-0.799999999999999,-0.784615384615384,-0.769230769230768,
-0.753846153846153,-0.738461538461538,-0.723076923076922,-0.707692307692307,
-0.692307692307692,-0.676923076923076,-0.661538461538461,-0.646153846153846,
-0.63076923076923,-0.615384615384615,-0.6,-0.584615384615384,-0.569230769230769,
-0.553846153846154,-0.538461538461538,-0.523076923076923,-0.507692307692308,
-0.492307692307692,-0.476923076923077,-0.461538461538462,-0.446153846153846,
-0.430769230769231,-0.415384615384615,-0.4,-0.384615384615385,-0.369230769230769,
-0.353846153846154,-0.338461538461538,-0.323076923076923,-0.307692307692308,
-0.292307692307692,-0.276923076923077,-0.261538461538462,-0.246153846153846,
-0.230769230769231,-0.215384615384615,-0.2,-0.184615384615385,-0.169230769230769,
-0.153846153846154,-0.138461538461538,-0.123076923076923,-0.107692307692308,
-0.0923076923076923,-0.0769230769230769,-0.0615384615384615,-0.0461538461538462,
-0.0307692307692308,-0.0153846153846154,0.),.UNSPECIFIED.)
CURVE()
GEOMETRIC_REPRESENTATION_ITEM()
RATIONAL_B_SPLINE_CURVE((1.,1.,1.,1.,1.,1.,1.,1.,1.,1.,1.,1.,1.,1.,1.,1.,
1.,1.,1.,1.,1.,1.,1.,1.,1.,1.,1.,1.,1.,1.,1.,1.,1.,1.,1.,1.,1.,1.,1.,1.,
1.,1.,1.,1.,1.,1.,1.,1.,1.,1.,1.,1.,1.,1.,1.,1.,1.,1.,1.,1.,1.,1.,1.,1.,
1.,1.,1.,1.,1.,1.))
REPRESENTATION_ITEM('')
);
#569=SHAPE_REPRESENTATION_RELATIONSHIP('SRR','None',#33531,#614);
#614=ADVANCED_BREP_SHAPE_REPRESENTATION('',(#717),#33293);
#666=STYLED_ITEM('',(#33828),#717);
#717=MANIFOLD_SOLID_BREP('Body1',#12685);
#878=FACE_BOUND('',#2749,.T.);
#879=FACE_BOUND('',#2753,.T.);
#880=FACE_BOUND('',#2834,.T.);
#1287=PLANE('',#14135);
#1288=PLANE('',#14136);
#1289=PLANE('',#14137);
#1290=PLANE('',#14138);
#1291=PLANE('',#14165);
#1292=PLANE('',#14166);
#1293=PLANE('',#14169);
#1294=PLANE('',#14172);
#1295=PLANE('',#14175);
#1296=PLANE('',#14178);
#1297=PLANE('',#14181);
#1298=PLANE('',#14184);
#1299=PLANE('',#14187);
#1300=PLANE('',#14190);
#1301=PLANE('',#14193);
#1302=PLANE('',#14196);
#1303=PLANE('',#14199);
#1304=PLANE('',#14202);
#1305=PLANE('',#14205);
#1306=PLANE('',#14208);
#1307=PLANE('',#14211);
#1308=PLANE('',#14214);
#1309=PLANE('',#14217);
#1310=PLANE('',#14220);
#1311=PLANE('',#14223);
#1312=PLANE('',#14224);
#1898=FACE_OUTER_BOUND('',#2745,.T.);
#1899=FACE_OUTER_BOUND('',#2746,.T.);
#1900=FACE_OUTER_BOUND('',#2747,.T.);
#1901=FACE_OUTER_BOUND('',#2748,.T.);
#1902=FACE_OUTER_BOUND('',#2750,.T.);
#1903=FACE_OUTER_BOUND('',#2751,.T.);
#1904=FACE_OUTER_BOUND('',#2752,.T.);
#1905=FACE_OUTER_BOUND('',#2754,.T.);
#1906=FACE_OUTER_BOUND('',#2755,.T.);
#1907=FACE_OUTER_BOUND('',#2756,.T.);
#1908=FACE_OUTER_BOUND('',#2757,.T.);
#1909=FACE_OUTER_BOUND('',#2758,.T.);
#1910=FACE_OUTER_BOUND('',#2759,.T.);
#1911=FACE_OUTER_BOUND('',#2760,.T.);
#1912=FACE_OUTER_BOUND('',#2761,.T.);
#1913=FACE_OUTER_BOUND('',#2762,.T.);
#1914=FACE_OUTER_BOUND('',#2763,.T.);
#1915=FACE_OUTER_BOUND('',#2764,.T.);
#1916=FACE_OUTER_BOUND('',#2765,.T.);
#1917=FACE_OUTER_BOUND('',#2766,.T.);
#1918=FACE_OUTER_BOUND('',#2767,.T.);
#1919=FACE_OUTER_BOUND('',#2768,.T.);
#1920=FACE_OUTER_BOUND('',#2769,.T.);
#1921=FACE_OUTER_BOUND('',#2770,.T.);
#1922=FACE_OUTER_BOUND('',#2771,.T.);
#1923=FACE_OUTER_BOUND('',#2772,.T.);
#1924=FACE_OUTER_BOUND('',#2773,.T.);
#1925=FACE_OUTER_BOUND('',#2774,.T.);
#1926=FACE_OUTER_BOUND('',#2775,.T.);
#1927=FACE_OUTER_BOUND('',#2776,.T.);
#1928=FACE_OUTER_BOUND('',#2777,.T.);
#1929=FACE_OUTER_BOUND('',#2778,.T.);
#1930=FACE_OUTER_BOUND('',#2779,.T.);
#1931=FACE_OUTER_BOUND('',#2780,.T.);
#1932=FACE_OUTER_BOUND('',#2781,.T.);
#1933=FACE_OUTER_BOUND('',#2782,.T.);
#1934=FACE_OUTER_BOUND('',#2783,.T.);
#1935=FACE_OUTER_BOUND('',#2784,.T.);
#1936=FACE_OUTER_BOUND('',#2785,.T.);
#1937=FACE_OUTER_BOUND('',#2786,.T.);
#1938=FACE_OUTER_BOUND('',#2787,.T.);
#1939=FACE_OUTER_BOUND('',#2788,.T.);
#1940=FACE_OUTER_BOUND('',#2789,.T.);
#1941=FACE_OUTER_BOUND('',#2790,.T.);
#1942=FACE_OUTER_BOUND('',#2791,.T.);
#1943=FACE_OUTER_BOUND('',#2792,.T.);
#1944=FACE_OUTER_BOUND('',#2793,.T.);
#1945=FACE_OUTER_BOUND('',#2794,.T.);
#1946=FACE_OUTER_BOUND('',#2795,.T.);
#1947=FACE_OUTER_BOUND('',#2796,.T.);
#1948=FACE_OUTER_BOUND('',#2797,.T.);
#1949=FACE_OUTER_BOUND('',#2798,.T.);
#1950=FACE_OUTER_BOUND('',#2799,.T.);
#1951=FACE_OUTER_BOUND('',#2800,.T.);
#1952=FACE_OUTER_BOUND('',#2801,.T.);
#1953=FACE_OUTER_BOUND('',#2802,.T.);
#1954=FACE_OUTER_BOUND('',#2803,.T.);
#1955=FACE_OUTER_BOUND('',#2804,.T.);
#1956=FACE_OUTER_BOUND('',#2805,.T.);
#1957=FACE_OUTER_BOUND('',#2806,.T.);
#1958=FACE_OUTER_BOUND('',#2807,.T.);
#1959=FACE_OUTER_BOUND('',#2808,.T.);
#1960=FACE_OUTER_BOUND('',#2809,.T.);
#1961=FACE_OUTER_BOUND('',#2810,.T.);
#1962=FACE_OUTER_BOUND('',#2811,.T.);
#1963=FACE_OUTER_BOUND('',#2812,.T.);
#1964=FACE_OUTER_BOUND('',#2813,.T.);
#1965=FACE_OUTER_BOUND('',#2814,.T.);
#1966=FACE_OUTER_BOUND('',#2815,.T.);
#1967=FACE_OUTER_BOUND('',#2816,.T.);
#1968=FACE_OUTER_BOUND('',#2817,.T.);
#1969=FACE_OUTER_BOUND('',#2818,.T.);
#1970=FACE_OUTER_BOUND('',#2819,.T.);
#1971=FACE_OUTER_BOUND('',#2820,.T.);
#1972=FACE_OUTER_BOUND('',#2821,.T.);
#1973=FACE_OUTER_BOUND('',#2822,.T.);
#1974=FACE_OUTER_BOUND('',#2823,.T.);
#1975=FACE_OUTER_BOUND('',#2824,.T.);
#1976=FACE_OUTER_BOUND('',#2825,.T.);
#1977=FACE_OUTER_BOUND('',#2826,.T.);
#1978=FACE_OUTER_BOUND('',#2827,.T.);
#1979=FACE_OUTER_BOUND('',#2828,.T.);
#1980=FACE_OUTER_BOUND('',#2829,.T.);
#1981=FACE_OUTER_BOUND('',#2830,.T.);
#1982=FACE_OUTER_BOUND('',#2831,.T.);
#1983=FACE_OUTER_BOUND('',#2832,.T.);
#1984=FACE_OUTER_BOUND('',#2833,.T.);
#1985=FACE_OUTER_BOUND('',#2835,.T.);
#2745=EDGE_LOOP('',(#11123,#11124,#11125,#11126));
#2746=EDGE_LOOP('',(#11127,#11128,#11129,#11130));
#2747=EDGE_LOOP('',(#11131,#11132,#11133,#11134));
#2748=EDGE_LOOP('',(#11135,#11136,#11137,#11138,#11139,#11140,#11141,#11142,
#11143,#11144,#11145,#11146,#11147,#11148,#11149,#11150,#11151,#11152,#11153,
#11154,#11155,#11156,#11157,#11158,#11159,#11160,#11161,#11162,#11163,#11164,
#11165,#11166,#11167,#11168,#11169,#11170,#11171,#11172,#11173,#11174,#11175,
#11176,#11177,#11178,#11179,#11180,#11181,#11182,#11183,#11184,#11185,#11186,
#11187,#11188,#11189,#11190,#11191,#11192,#11193,#11194,#11195,#11196,#11197,
#11198,#11199,#11200,#11201,#11202,#11203,#11204,#11205,#11206,#11207,#11208,
#11209,#11210,#11211,#11212,#11213,#11214));
#2749=EDGE_LOOP('',(#11215,#11216,#11217,#11218));
#2750=EDGE_LOOP('',(#11219,#11220,#11221,#11222));
#2751=EDGE_LOOP('',(#11223,#11224,#11225,#11226));
#2752=EDGE_LOOP('',(#11227));
#2753=EDGE_LOOP('',(#11228,#11229,#11230,#11231));
#2754=EDGE_LOOP('',(#11232,#11233,#11234,#11235));
#2755=EDGE_LOOP('',(#11236,#11237,#11238,#11239));
#2756=EDGE_LOOP('',(#11240,#11241,#11242,#11243));
#2757=EDGE_LOOP('',(#11244,#11245,#11246,#11247));
#2758=EDGE_LOOP('',(#11248,#11249,#11250,#11251));
#2759=EDGE_LOOP('',(#11252,#11253,#11254,#11255));
#2760=EDGE_LOOP('',(#11256,#11257,#11258,#11259));
#2761=EDGE_LOOP('',(#11260,#11261,#11262,#11263));
#2762=EDGE_LOOP('',(#11264,#11265,#11266,#11267));
#2763=EDGE_LOOP('',(#11268,#11269,#11270,#11271));
#2764=EDGE_LOOP('',(#11272,#11273,#11274,#11275));
#2765=EDGE_LOOP('',(#11276,#11277,#11278,#11279));
#2766=EDGE_LOOP('',(#11280,#11281,#11282,#11283));
#2767=EDGE_LOOP('',(#11284,#11285,#11286,#11287));
#2768=EDGE_LOOP('',(#11288,#11289,#11290,#11291));
#2769=EDGE_LOOP('',(#11292,#11293,#11294,#11295));
#2770=EDGE_LOOP('',(#11296,#11297,#11298,#11299));
#2771=EDGE_LOOP('',(#11300,#11301,#11302,#11303));
#2772=EDGE_LOOP('',(#11304,#11305,#11306,#11307));
#2773=EDGE_LOOP('',(#11308,#11309,#11310,#11311));
#2774=EDGE_LOOP('',(#11312,#11313,#11314,#11315));
#2775=EDGE_LOOP('',(#11316,#11317,#11318,#11319));
#2776=EDGE_LOOP('',(#11320,#11321,#11322,#11323));
#2777=EDGE_LOOP('',(#11324,#11325,#11326,#11327));
#2778=EDGE_LOOP('',(#11328,#11329,#11330,#11331));
#2779=EDGE_LOOP('',(#11332,#11333,#11334,#11335));
#2780=EDGE_LOOP('',(#11336,#11337,#11338,#11339));
#2781=EDGE_LOOP('',(#11340,#11341,#11342,#11343));
#2782=EDGE_LOOP('',(#11344,#11345,#11346,#11347));
#2783=EDGE_LOOP('',(#11348,#11349,#11350,#11351));
#2784=EDGE_LOOP('',(#11352,#11353,#11354,#11355));
#2785=EDGE_LOOP('',(#11356,#11357,#11358,#11359));
#2786=EDGE_LOOP('',(#11360,#11361,#11362,#11363));
#2787=EDGE_LOOP('',(#11364,#11365,#11366,#11367));
#2788=EDGE_LOOP('',(#11368,#11369,#11370,#11371));
#2789=EDGE_LOOP('',(#11372,#11373,#11374,#11375));
#2790=EDGE_LOOP('',(#11376,#11377,#11378,#11379));
#2791=EDGE_LOOP('',(#11380,#11381,#11382,#11383));
#2792=EDGE_LOOP('',(#11384,#11385,#11386,#11387));
#2793=EDGE_LOOP('',(#11388,#11389,#11390,#11391));
#2794=EDGE_LOOP('',(#11392,#11393,#11394,#11395));
#2795=EDGE_LOOP('',(#11396,#11397,#11398,#11399));
#2796=EDGE_LOOP('',(#11400,#11401,#11402,#11403));
#2797=EDGE_LOOP('',(#11404,#11405,#11406,#11407));
#2798=EDGE_LOOP('',(#11408,#11409,#11410,#11411));
#2799=EDGE_LOOP('',(#11412,#11413,#11414,#11415));
#2800=EDGE_LOOP('',(#11416,#11417,#11418,#11419));
#2801=EDGE_LOOP('',(#11420,#11421,#11422,#11423));
#2802=EDGE_LOOP('',(#11424,#11425,#11426,#11427));
#2803=EDGE_LOOP('',(#11428,#11429,#11430,#11431));
#2804=EDGE_LOOP('',(#11432,#11433,#11434,#11435));
#2805=EDGE_LOOP('',(#11436,#11437,#11438,#11439));
#2806=EDGE_LOOP('',(#11440,#11441,#11442,#11443));
#2807=EDGE_LOOP('',(#11444,#11445,#11446,#11447));
#2808=EDGE_LOOP('',(#11448,#11449,#11450,#11451));
#2809=EDGE_LOOP('',(#11452,#11453,#11454,#11455));
#2810=EDGE_LOOP('',(#11456,#11457,#11458,#11459));
#2811=EDGE_LOOP('',(#11460,#11461,#11462,#11463));
#2812=EDGE_LOOP('',(#11464,#11465,#11466,#11467));
#2813=EDGE_LOOP('',(#11468,#11469,#11470,#11471));
#2814=EDGE_LOOP('',(#11472,#11473,#11474,#11475));
#2815=EDGE_LOOP('',(#11476,#11477,#11478,#11479));
#2816=EDGE_LOOP('',(#11480,#11481,#11482,#11483));
#2817=EDGE_LOOP('',(#11484,#11485,#11486,#11487));
#2818=EDGE_LOOP('',(#11488,#11489,#11490,#11491));
#2819=EDGE_LOOP('',(#11492,#11493,#11494,#11495));
#2820=EDGE_LOOP('',(#11496,#11497,#11498,#11499));
#2821=EDGE_LOOP('',(#11500,#11501,#11502,#11503));
#2822=EDGE_LOOP('',(#11504,#11505,#11506,#11507));
#2823=EDGE_LOOP('',(#11508,#11509,#11510,#11511));
#2824=EDGE_LOOP('',(#11512,#11513,#11514,#11515));
#2825=EDGE_LOOP('',(#11516,#11517,#11518,#11519));
#2826=EDGE_LOOP('',(#11520,#11521,#11522,#11523));
#2827=EDGE_LOOP('',(#11524,#11525,#11526,#11527));
#2828=EDGE_LOOP('',(#11528,#11529,#11530,#11531));
#2829=EDGE_LOOP('',(#11532,#11533,#11534,#11535));
#2830=EDGE_LOOP('',(#11536,#11537,#11538,#11539));
#2831=EDGE_LOOP('',(#11540,#11541,#11542,#11543));
#2832=EDGE_LOOP('',(#11544,#11545,#11546,#11547));
#2833=EDGE_LOOP('',(#11548,#11549,#11550,#11551,#11552,#11553,#11554,#11555,
#11556,#11557,#11558,#11559,#11560,#11561,#11562,#11563,#11564,#11565,#11566,
#11567,#11568,#11569,#11570,#11571,#11572,#11573,#11574,#11575,#11576,#11577,
#11578,#11579,#11580,#11581,#11582,#11583,#11584,#11585,#11586,#11587,#11588,
#11589,#11590,#11591,#11592,#11593,#11594,#11595,#11596,#11597,#11598,#11599,
#11600,#11601,#11602,#11603,#11604,#11605,#11606,#11607,#11608,#11609,#11610,
#11611,#11612,#11613,#11614,#11615,#11616,#11617,#11618,#11619,#11620,#11621,
#11622,#11623,#11624,#11625,#11626,#11627));
#2834=EDGE_LOOP('',(#11628));
#2835=EDGE_LOOP('',(#11629,#11630,#11631,#11632));
#3866=LINE('',#21366,#5031);
#3867=LINE('',#21368,#5032);
#3868=LINE('',#21370,#5033);
#3869=LINE('',#21371,#5034);
#3870=LINE('',#21374,#5035);
#3871=LINE('',#21376,#5036);
#3872=LINE('',#21377,#5037);
#3873=LINE('',#21380,#5038);
#3874=LINE('',#21382,#5039);
#3875=LINE('',#21383,#5040);
#3876=LINE('',#21460,#5041);
#3877=LINE('',#21606,#5042);
#3878=LINE('',#21752,#5043);
#3879=LINE('',#21898,#5044);
#3880=LINE('',#22044,#5045);
#3881=LINE('',#22190,#5046);
#3882=LINE('',#22336,#5047);
#3883=LINE('',#22482,#5048);
#3884=LINE('',#22628,#5049);
#3885=LINE('',#22774,#5050);
#3886=LINE('',#22920,#5051);
#3887=LINE('',#23066,#5052);
#3888=LINE('',#23212,#5053);
#3889=LINE('',#23358,#5054);
#3890=LINE('',#23504,#5055);
#3891=LINE('',#23650,#5056);
#3892=LINE('',#23796,#5057);
#3893=LINE('',#23942,#5058);
#3894=LINE('',#24088,#5059);
#3895=LINE('',#24234,#5060);
#3896=LINE('',#24312,#5061);
#3897=LINE('',#24456,#5062);
#3898=LINE('',#24528,#5063);
#3899=LINE('',#24531,#5064);
#3900=LINE('',#24532,#5065);
#3901=LINE('',#24744,#5066);
#3902=LINE('',#24748,#5067);
#3903=LINE('',#24960,#5068);
#3904=LINE('',#24963,#5069);
#3905=LINE('',#24964,#5070);
#3906=LINE('',#25176,#5071);
#3907=LINE('',#25180,#5072);
#3908=LINE('',#25392,#5073);
#3909=LINE('',#25395,#5074);
#3910=LINE('',#25396,#5075);
#3911=LINE('',#25608,#5076);
#3912=LINE('',#25612,#5077);
#3913=LINE('',#25824,#5078);
#3914=LINE('',#25827,#5079);
#3915=LINE('',#25828,#5080);
#3916=LINE('',#26040,#5081);
#3917=LINE('',#26044,#5082);
#3918=LINE('',#26256,#5083);
#3919=LINE('',#26259,#5084);
#3920=LINE('',#26260,#5085);
#3921=LINE('',#26472,#5086);
#3922=LINE('',#26476,#5087);
#3923=LINE('',#26688,#5088);
#3924=LINE('',#26691,#5089);
#3925=LINE('',#26692,#5090);
#3926=LINE('',#26904,#5091);
#3927=LINE('',#26908,#5092);
#3928=LINE('',#27120,#5093);
#3929=LINE('',#27123,#5094);
#3930=LINE('',#27124,#5095);
#3931=LINE('',#27336,#5096);
#3932=LINE('',#27340,#5097);
#3933=LINE('',#27552,#5098);
#3934=LINE('',#27555,#5099);
#3935=LINE('',#27556,#5100);
#3936=LINE('',#27768,#5101);
#3937=LINE('',#27772,#5102);
#3938=LINE('',#27984,#5103);
#3939=LINE('',#27987,#5104);
#3940=LINE('',#27988,#5105);
#3941=LINE('',#28200,#5106);
#3942=LINE('',#28204,#5107);
#3943=LINE('',#28416,#5108);
#3944=LINE('',#28419,#5109);
#3945=LINE('',#28420,#5110);
#3946=LINE('',#28632,#5111);
#3947=LINE('',#28636,#5112);
#3948=LINE('',#28848,#5113);
#3949=LINE('',#28851,#5114);
#3950=LINE('',#28852,#5115);
#3951=LINE('',#29064,#5116);
#3952=LINE('',#29068,#5117);
#3953=LINE('',#29280,#5118);
#3954=LINE('',#29283,#5119);
#3955=LINE('',#29284,#5120);
#3956=LINE('',#29496,#5121);
#3957=LINE('',#29500,#5122);
#3958=LINE('',#29712,#5123);
#3959=LINE('',#29715,#5124);
#3960=LINE('',#29716,#5125);
#3961=LINE('',#29928,#5126);
#3962=LINE('',#29932,#5127);
#3963=LINE('',#30144,#5128);
#3964=LINE('',#30147,#5129);
#3965=LINE('',#30148,#5130);
#3966=LINE('',#30360,#5131);
#3967=LINE('',#30364,#5132);
#3968=LINE('',#30576,#5133);
#3969=LINE('',#30579,#5134);
#3970=LINE('',#30580,#5135);
#3971=LINE('',#30792,#5136);
#3972=LINE('',#30796,#5137);
#3973=LINE('',#31008,#5138);
#3974=LINE('',#31011,#5139);
#3975=LINE('',#31012,#5140);
#3976=LINE('',#31224,#5141);
#3977=LINE('',#31228,#5142);
#3978=LINE('',#31440,#5143);
#3979=LINE('',#31443,#5144);
#3980=LINE('',#31444,#5145);
#3981=LINE('',#31656,#5146);
#3982=LINE('',#31660,#5147);
#3983=LINE('',#31872,#5148);
#3984=LINE('',#31875,#5149);
#3985=LINE('',#31876,#5150);
#3986=LINE('',#32088,#5151);
#3987=LINE('',#32092,#5152);
#3988=LINE('',#32304,#5153);
#3989=LINE('',#32307,#5154);
#3990=LINE('',#32308,#5155);
#3991=LINE('',#32520,#5156);
#3992=LINE('',#32524,#5157);
#3993=LINE('',#32736,#5158);
#3994=LINE('',#32739,#5159);
#3995=LINE('',#32740,#5160);
#3996=LINE('',#32952,#5161);
#5031=VECTOR('',#17245,1.);
#5032=VECTOR('',#17246,1.);
#5033=VECTOR('',#17247,1.);
#5034=VECTOR('',#17248,1.);
#5035=VECTOR('',#17251,1.);
#5036=VECTOR('',#17252,1.);
#5037=VECTOR('',#17253,1.);
#5038=VECTOR('',#17256,1.);
#5039=VECTOR('',#17257,1.);
#5040=VECTOR('',#17258,1.);
#5041=VECTOR('',#17263,1.);
#5042=VECTOR('',#17266,1.);
#5043=VECTOR('',#17269,1.);
#5044=VECTOR('',#17272,1.);
#5045=VECTOR('',#17275,1.);
#5046=VECTOR('',#17278,1.);
#5047=VECTOR('',#17281,1.);
#5048=VECTOR('',#17284,1.);
#5049=VECTOR('',#17287,1.);
#5050=VECTOR('',#17290,1.);
#5051=VECTOR('',#17293,1.);
#5052=VECTOR('',#17296,1.);
#5053=VECTOR('',#17299,1.);
#5054=VECTOR('',#17302,1.);
#5055=VECTOR('',#17305,1.);
#5056=VECTOR('',#17308,1.);
#5057=VECTOR('',#17311,1.);
#5058=VECTOR('',#17314,1.);
#5059=VECTOR('',#17317,1.);
#5060=VECTOR('',#17320,1.);
#5061=VECTOR('',#17331,1.4);
#5062=VECTOR('',#17336,1.);
#5063=VECTOR('',#17337,1.);
#5064=VECTOR('',#17340,1.);
#5065=VECTOR('',#17341,1.);
#5066=VECTOR('',#17342,1.);
#5067=VECTOR('',#17347,1.);
#5068=VECTOR('',#17348,1.);
#5069=VECTOR('',#17351,1.);
#5070=VECTOR('',#17352,1.);
#5071=VECTOR('',#17353,1.);
#5072=VECTOR('',#17358,1.);
#5073=VECTOR('',#17359,1.);
#5074=VECTOR('',#17362,1.);
#5075=VECTOR('',#17363,1.);
#5076=VECTOR('',#17364,1.);
#5077=VECTOR('',#17369,1.);
#5078=VECTOR('',#17370,1.);
#5079=VECTOR('',#17373,1.);
#5080=VECTOR('',#17374,1.);
#5081=VECTOR('',#17375,1.);
#5082=VECTOR('',#17380,1.);
#5083=VECTOR('',#17381,1.);
#5084=VECTOR('',#17384,1.);
#5085=VECTOR('',#17385,1.);
#5086=VECTOR('',#17386,1.);
#5087=VECTOR('',#17391,1.);
#5088=VECTOR('',#17392,1.);
#5089=VECTOR('',#17395,1.);
#5090=VECTOR('',#17396,1.);
#5091=VECTOR('',#17397,1.);
#5092=VECTOR('',#17402,1.);
#5093=VECTOR('',#17403,1.);
#5094=VECTOR('',#17406,1.);
#5095=VECTOR('',#17407,1.);
#5096=VECTOR('',#17408,1.);
#5097=VECTOR('',#17413,1.);
#5098=VECTOR('',#17414,1.);
#5099=VECTOR('',#17417,1.);
#5100=VECTOR('',#17418,1.);
#5101=VECTOR('',#17419,1.);
#5102=VECTOR('',#17424,1.);
#5103=VECTOR('',#17425,1.);
#5104=VECTOR('',#17428,1.);
#5105=VECTOR('',#17429,1.);
#5106=VECTOR('',#17430,1.);
#5107=VECTOR('',#17435,1.);
#5108=VECTOR('',#17436,1.);
#5109=VECTOR('',#17439,1.);
#5110=VECTOR('',#17440,1.);
#5111=VECTOR('',#17441,1.);
#5112=VECTOR('',#17446,1.);
#5113=VECTOR('',#17447,1.);
#5114=VECTOR('',#17450,1.);
#5115=VECTOR('',#17451,1.);
#5116=VECTOR('',#17452,1.);
#5117=VECTOR('',#17457,1.);
#5118=VECTOR('',#17458,1.);
#5119=VECTOR('',#17461,1.);
#5120=VECTOR('',#17462,1.);
#5121=VECTOR('',#17463,1.);
#5122=VECTOR('',#17468,1.);
#5123=VECTOR('',#17469,1.);
#5124=VECTOR('',#17472,1.);
#5125=VECTOR('',#17473,1.);
#5126=VECTOR('',#17474,1.);
#5127=VECTOR('',#17479,1.);
#5128=VECTOR('',#17480,1.);
#5129=VECTOR('',#17483,1.);
#5130=VECTOR('',#17484,1.);
#5131=VECTOR('',#17485,1.);
#5132=VECTOR('',#17490,1.);
#5133=VECTOR('',#17491,1.);
#5134=VECTOR('',#17494,1.);
#5135=VECTOR('',#17495,1.);
#5136=VECTOR('',#17496,1.);
#5137=VECTOR('',#17501,1.);
#5138=VECTOR('',#17502,1.);
#5139=VECTOR('',#17505,1.);
#5140=VECTOR('',#17506,1.);
#5141=VECTOR('',#17507,1.);
#5142=VECTOR('',#17512,1.);
#5143=VECTOR('',#17513,1.);
#5144=VECTOR('',#17516,1.);
#5145=VECTOR('',#17517,1.);
#5146=VECTOR('',#17518,1.);
#5147=VECTOR('',#17523,1.);
#5148=VECTOR('',#17524,1.);
#5149=VECTOR('',#17527,1.);
#5150=VECTOR('',#17528,1.);
#5151=VECTOR('',#17529,1.);
#5152=VECTOR('',#17534,1.);
#5153=VECTOR('',#17535,1.);
#5154=VECTOR('',#17538,1.);
#5155=VECTOR('',#17539,1.);
#5156=VECTOR('',#17540,1.);
#5157=VECTOR('',#17545,1.);
#5158=VECTOR('',#17546,1.);
#5159=VECTOR('',#17549,1.);
#5160=VECTOR('',#17550,1.);
#5161=VECTOR('',#17551,1.);
#5545=CIRCLE('',#14139,1.75);
#5546=CIRCLE('',#14140,1.75);
#5547=CIRCLE('',#14141,1.75);
#5548=CIRCLE('',#14142,1.75);
#5549=CIRCLE('',#14143,1.75);
#5550=CIRCLE('',#14144,1.75);
#5551=CIRCLE('',#14145,1.75);
#5552=CIRCLE('',#14146,1.75);
#5553=CIRCLE('',#14147,1.75);
#5554=CIRCLE('',#14148,1.75);
#5555=CIRCLE('',#14149,1.75);
#5556=CIRCLE('',#14150,1.75);
#5557=CIRCLE('',#14151,1.75);
#5558=CIRCLE('',#14152,1.75);
#5559=CIRCLE('',#14153,1.75);
#5560=CIRCLE('',#14154,1.75);
#5561=CIRCLE('',#14155,1.75);
#5562=CIRCLE('',#14156,1.75);
#5563=CIRCLE('',#14157,1.75);
#5564=CIRCLE('',#14158,1.75);
#5565=CIRCLE('',#14159,0.6);
#5566=CIRCLE('',#14161,0.6);
#5567=CIRCLE('',#14163,1.4);
#5568=CIRCLE('',#14164,1.4);
#5569=CIRCLE('',#14168,1.75);
#5570=CIRCLE('',#14171,1.75);
#5571=CIRCLE('',#14174,1.75);
#5572=CIRCLE('',#14177,1.75);
#5573=CIRCLE('',#14180,1.75);
#5574=CIRCLE('',#14183,1.75);
#5575=CIRCLE('',#14186,1.75);
#5576=CIRCLE('',#14189,1.75);
#5577=CIRCLE('',#14192,1.75);
#5578=CIRCLE('',#14195,1.75);
#5579=CIRCLE('',#14198,1.75);
#5580=CIRCLE('',#14201,1.75);
#5581=CIRCLE('',#14204,1.75);
#5582=CIRCLE('',#14207,1.75);
#5583=CIRCLE('',#14210,1.75);
#5584=CIRCLE('',#14213,1.75);
#5585=CIRCLE('',#14216,1.75);
#5586=CIRCLE('',#14219,1.75);
#5587=CIRCLE('',#14222,1.75);
#5588=CIRCLE('',#14225,1.75);
#6521=VERTEX_POINT('',#21364);
#6522=VERTEX_POINT('',#21365);
#6523=VERTEX_POINT('',#21367);
#6524=VERTEX_POINT('',#21369);
#6525=VERTEX_POINT('',#21373);
#6526=VERTEX_POINT('',#21375);
#6527=VERTEX_POINT('',#21379);
#6528=VERTEX_POINT('',#21381);
#6529=VERTEX_POINT('',#21385);
#6530=VERTEX_POINT('',#21386);
#6531=VERTEX_POINT('',#21388);
#6532=VERTEX_POINT('',#21459);
#6533=VERTEX_POINT('',#21461);
#6534=VERTEX_POINT('',#21532);
#6535=VERTEX_POINT('',#21534);
#6536=VERTEX_POINT('',#21605);
#6537=VERTEX_POINT('',#21607);
#6538=VERTEX_POINT('',#21678);
#6539=VERTEX_POINT('',#21680);
#6540=VERTEX_POINT('',#21751);
#6541=VERTEX_POINT('',#21753);
#6542=VERTEX_POINT('',#21824);
#6543=VERTEX_POINT('',#21826);
#6544=VERTEX_POINT('',#21897);
#6545=VERTEX_POINT('',#21899);
#6546=VERTEX_POINT('',#21970);
#6547=VERTEX_POINT('',#21972);
#6548=VERTEX_POINT('',#22043);
#6549=VERTEX_POINT('',#22045);
#6550=VERTEX_POINT('',#22116);
#6551=VERTEX_POINT('',#22118);
#6552=VERTEX_POINT('',#22189);
#6553=VERTEX_POINT('',#22191);
#6554=VERTEX_POINT('',#22262);
#6555=VERTEX_POINT('',#22264);
#6556=VERTEX_POINT('',#22335);
#6557=VERTEX_POINT('',#22337);
#6558=VERTEX_POINT('',#22408);
#6559=VERTEX_POINT('',#22410);
#6560=VERTEX_POINT('',#22481);
#6561=VERTEX_POINT('',#22483);
#6562=VERTEX_POINT('',#22554);
#6563=VERTEX_POINT('',#22556);
#6564=VERTEX_POINT('',#22627);
#6565=VERTEX_POINT('',#22629);
#6566=VERTEX_POINT('',#22700);
#6567=VERTEX_POINT('',#22702);
#6568=VERTEX_POINT('',#22773);
#6569=VERTEX_POINT('',#22775);
#6570=VERTEX_POINT('',#22846);
#6571=VERTEX_POINT('',#22848);
#6572=VERTEX_POINT('',#22919);
#6573=VERTEX_POINT('',#22921);
#6574=VERTEX_POINT('',#22992);
#6575=VERTEX_POINT('',#22994);
#6576=VERTEX_POINT('',#23065);
#6577=VERTEX_POINT('',#23067);
#6578=VERTEX_POINT('',#23138);
#6579=VERTEX_POINT('',#23140);
#6580=VERTEX_POINT('',#23211);
#6581=VERTEX_POINT('',#23213);
#6582=VERTEX_POINT('',#23284);
#6583=VERTEX_POINT('',#23286);
#6584=VERTEX_POINT('',#23357);
#6585=VERTEX_POINT('',#23359);
#6586=VERTEX_POINT('',#23430);
#6587=VERTEX_POINT('',#23432);
#6588=VERTEX_POINT('',#23503);
#6589=VERTEX_POINT('',#23505);
#6590=VERTEX_POINT('',#23576);
#6591=VERTEX_POINT('',#23578);
#6592=VERTEX_POINT('',#23649);
#6593=VERTEX_POINT('',#23651);
#6594=VERTEX_POINT('',#23722);
#6595=VERTEX_POINT('',#23724);
#6596=VERTEX_POINT('',#23795);
#6597=VERTEX_POINT('',#23797);
#6598=VERTEX_POINT('',#23868);
#6599=VERTEX_POINT('',#23870);
#6600=VERTEX_POINT('',#23941);
#6601=VERTEX_POINT('',#23943);
#6602=VERTEX_POINT('',#24014);
#6603=VERTEX_POINT('',#24016);
#6604=VERTEX_POINT('',#24087);
#6605=VERTEX_POINT('',#24089);
#6606=VERTEX_POINT('',#24160);
#6607=VERTEX_POINT('',#24162);
#6608=VERTEX_POINT('',#24233);
#6609=VERTEX_POINT('',#24309);
#6610=VERTEX_POINT('',#24311);
#6611=VERTEX_POINT('',#24455);
#6612=VERTEX_POINT('',#24457);
#6613=VERTEX_POINT('',#24530);
#6614=VERTEX_POINT('',#24673);
#6615=VERTEX_POINT('',#24746);
#6616=VERTEX_POINT('',#24889);
#6617=VERTEX_POINT('',#24962);
#6618=VERTEX_POINT('',#25105);
#6619=VERTEX_POINT('',#25178);
#6620=VERTEX_POINT('',#25321);
#6621=VERTEX_POINT('',#25394);
#6622=VERTEX_POINT('',#25537);
#6623=VERTEX_POINT('',#25610);
#6624=VERTEX_POINT('',#25753);
#6625=VERTEX_POINT('',#25826);
#6626=VERTEX_POINT('',#25969);
#6627=VERTEX_POINT('',#26042);
#6628=VERTEX_POINT('',#26185);
#6629=VERTEX_POINT('',#26258);
#6630=VERTEX_POINT('',#26401);
#6631=VERTEX_POINT('',#26474);
#6632=VERTEX_POINT('',#26617);
#6633=VERTEX_POINT('',#26690);
#6634=VERTEX_POINT('',#26833);
#6635=VERTEX_POINT('',#26906);
#6636=VERTEX_POINT('',#27049);
#6637=VERTEX_POINT('',#27122);
#6638=VERTEX_POINT('',#27265);
#6639=VERTEX_POINT('',#27338);
#6640=VERTEX_POINT('',#27481);
#6641=VERTEX_POINT('',#27554);
#6642=VERTEX_POINT('',#27697);
#6643=VERTEX_POINT('',#27770);
#6644=VERTEX_POINT('',#27913);
#6645=VERTEX_POINT('',#27986);
#6646=VERTEX_POINT('',#28129);
#6647=VERTEX_POINT('',#28202);
#6648=VERTEX_POINT('',#28345);
#6649=VERTEX_POINT('',#28418);
#6650=VERTEX_POINT('',#28561);
#6651=VERTEX_POINT('',#28634);
#6652=VERTEX_POINT('',#28777);
#6653=VERTEX_POINT('',#28850);
#6654=VERTEX_POINT('',#28993);
#6655=VERTEX_POINT('',#29066);
#6656=VERTEX_POINT('',#29209);
#6657=VERTEX_POINT('',#29282);
#6658=VERTEX_POINT('',#29425);
#6659=VERTEX_POINT('',#29498);
#6660=VERTEX_POINT('',#29641);
#6661=VERTEX_POINT('',#29714);
#6662=VERTEX_POINT('',#29857);
#6663=VERTEX_POINT('',#29930);
#6664=VERTEX_POINT('',#30073);
#6665=VERTEX_POINT('',#30146);
#6666=VERTEX_POINT('',#30289);
#6667=VERTEX_POINT('',#30362);
#6668=VERTEX_POINT('',#30505);
#6669=VERTEX_POINT('',#30578);
#6670=VERTEX_POINT('',#30721);
#6671=VERTEX_POINT('',#30794);
#6672=VERTEX_POINT('',#30937);
#6673=VERTEX_POINT('',#31010);
#6674=VERTEX_POINT('',#31153);
#6675=VERTEX_POINT('',#31226);
#6676=VERTEX_POINT('',#31369);
#6677=VERTEX_POINT('',#31442);
#6678=VERTEX_POINT('',#31585);
#6679=VERTEX_POINT('',#31658);
#6680=VERTEX_POINT('',#31801);
#6681=VERTEX_POINT('',#31874);
#6682=VERTEX_POINT('',#32017);
#6683=VERTEX_POINT('',#32090);
#6684=VERTEX_POINT('',#32233);
#6685=VERTEX_POINT('',#32306);
#6686=VERTEX_POINT('',#32449);
#6687=VERTEX_POINT('',#32522);
#6688=VERTEX_POINT('',#32665);
#6689=VERTEX_POINT('',#32738);
#6690=VERTEX_POINT('',#32881);
#8090=EDGE_CURVE('',#6521,#6522,#3866,.T.);
#8091=EDGE_CURVE('',#6523,#6521,#3867,.T.);
#8092=EDGE_CURVE('',#6524,#6523,#3868,.T.);
#8093=EDGE_CURVE('',#6522,#6524,#3869,.T.);
#8094=EDGE_CURVE('',#6525,#6521,#3870,.T.);
#8095=EDGE_CURVE('',#6525,#6526,#3871,.T.);
#8096=EDGE_CURVE('',#6523,#6526,#3872,.T.);
#8097=EDGE_CURVE('',#6527,#6525,#3873,.T.);
#8098=EDGE_CURVE('',#6528,#6527,#3874,.T.);
#8099=EDGE_CURVE('',#6526,#6528,#3875,.T.);
#8100=EDGE_CURVE('',#6529,#6530,#5545,.T.);
#8101=EDGE_CURVE('',#6530,#6531,#51,.T.);
#8102=EDGE_CURVE('',#6531,#6532,#3876,.T.);
#8103=EDGE_CURVE('',#6532,#6533,#52,.T.);
#8104=EDGE_CURVE('',#6533,#6534,#5546,.T.);
#8105=EDGE_CURVE('',#6534,#6535,#53,.T.);
#8106=EDGE_CURVE('',#6535,#6536,#3877,.T.);
#8107=EDGE_CURVE('',#6536,#6537,#54,.T.);
#8108=EDGE_CURVE('',#6537,#6538,#5547,.T.);
#8109=EDGE_CURVE('',#6538,#6539,#55,.T.);
#8110=EDGE_CURVE('',#6539,#6540,#3878,.T.);
#8111=EDGE_CURVE('',#6540,#6541,#56,.T.);
#8112=EDGE_CURVE('',#6541,#6542,#5548,.T.);
#8113=EDGE_CURVE('',#6542,#6543,#57,.T.);
#8114=EDGE_CURVE('',#6543,#6544,#3879,.T.);
#8115=EDGE_CURVE('',#6544,#6545,#58,.T.);
#8116=EDGE_CURVE('',#6545,#6546,#5549,.T.);
#8117=EDGE_CURVE('',#6546,#6547,#59,.T.);
#8118=EDGE_CURVE('',#6547,#6548,#3880,.T.);
#8119=EDGE_CURVE('',#6548,#6549,#60,.T.);
#8120=EDGE_CURVE('',#6549,#6550,#5550,.T.);
#8121=EDGE_CURVE('',#6550,#6551,#61,.T.);
#8122=EDGE_CURVE('',#6551,#6552,#3881,.T.);
#8123=EDGE_CURVE('',#6552,#6553,#62,.T.);
#8124=EDGE_CURVE('',#6553,#6554,#5551,.T.);
#8125=EDGE_CURVE('',#6554,#6555,#63,.T.);
#8126=EDGE_CURVE('',#6555,#6556,#3882,.T.);
#8127=EDGE_CURVE('',#6556,#6557,#64,.T.);
#8128=EDGE_CURVE('',#6557,#6558,#5552,.T.);
#8129=EDGE_CURVE('',#6558,#6559,#65,.T.);
#8130=EDGE_CURVE('',#6559,#6560,#3883,.T.);
#8131=EDGE_CURVE('',#6560,#6561,#66,.T.);
#8132=EDGE_CURVE('',#6561,#6562,#5553,.T.);
#8133=EDGE_CURVE('',#6562,#6563,#67,.T.);
#8134=EDGE_CURVE('',#6563,#6564,#3884,.T.);
#8135=EDGE_CURVE('',#6564,#6565,#68,.T.);
#8136=EDGE_CURVE('',#6565,#6566,#5554,.T.);
#8137=EDGE_CURVE('',#6566,#6567,#69,.T.);
#8138=EDGE_CURVE('',#6567,#6568,#3885,.T.);
#8139=EDGE_CURVE('',#6568,#6569,#70,.T.);
#8140=EDGE_CURVE('',#6569,#6570,#5555,.T.);
#8141=EDGE_CURVE('',#6570,#6571,#71,.T.);
#8142=EDGE_CURVE('',#6571,#6572,#3886,.T.);
#8143=EDGE_CURVE('',#6572,#6573,#72,.T.);
#8144=EDGE_CURVE('',#6573,#6574,#5556,.T.);
#8145=EDGE_CURVE('',#6574,#6575,#73,.T.);
#8146=EDGE_CURVE('',#6575,#6576,#3887,.T.);
#8147=EDGE_CURVE('',#6576,#6577,#74,.T.);
#8148=EDGE_CURVE('',#6577,#6578,#5557,.T.);
#8149=EDGE_CURVE('',#6578,#6579,#75,.T.);
#8150=EDGE_CURVE('',#6579,#6580,#3888,.T.);
#8151=EDGE_CURVE('',#6580,#6581,#76,.T.);
#8152=EDGE_CURVE('',#6581,#6582,#5558,.T.);
#8153=EDGE_CURVE('',#6582,#6583,#77,.T.);
#8154=EDGE_CURVE('',#6583,#6584,#3889,.T.);
#8155=EDGE_CURVE('',#6584,#6585,#78,.T.);
#8156=EDGE_CURVE('',#6585,#6586,#5559,.T.);
#8157=EDGE_CURVE('',#6586,#6587,#79,.T.);
#8158=EDGE_CURVE('',#6587,#6588,#3890,.T.);
#8159=EDGE_CURVE('',#6588,#6589,#80,.T.);
#8160=EDGE_CURVE('',#6589,#6590,#5560,.T.);
#8161=EDGE_CURVE('',#6590,#6591,#81,.T.);
#8162=EDGE_CURVE('',#6591,#6592,#3891,.T.);
#8163=EDGE_CURVE('',#6592,#6593,#82,.T.);
#8164=EDGE_CURVE('',#6593,#6594,#5561,.T.);
#8165=EDGE_CURVE('',#6594,#6595,#83,.T.);
#8166=EDGE_CURVE('',#6595,#6596,#3892,.T.);
#8167=EDGE_CURVE('',#6596,#6597,#84,.T.);
#8168=EDGE_CURVE('',#6597,#6598,#5562,.T.);
#8169=EDGE_CURVE('',#6598,#6599,#85,.T.);
#8170=EDGE_CURVE('',#6599,#6600,#3893,.T.);
#8171=EDGE_CURVE('',#6600,#6601,#86,.T.);
#8172=EDGE_CURVE('',#6601,#6602,#5563,.T.);
#8173=EDGE_CURVE('',#6602,#6603,#87,.T.);
#8174=EDGE_CURVE('',#6603,#6604,#3894,.T.);
#8175=EDGE_CURVE('',#6604,#6605,#88,.T.);
#8176=EDGE_CURVE('',#6605,#6606,#5564,.T.);
#8177=EDGE_CURVE('',#6606,#6607,#89,.T.);
#8178=EDGE_CURVE('',#6607,#6608,#3895,.T.);
#8179=EDGE_CURVE('',#6608,#6529,#90,.T.);
#8180=EDGE_CURVE('',#6528,#6524,#5565,.T.);
#8181=EDGE_CURVE('',#6522,#6527,#5566,.T.);
#8182=EDGE_CURVE('',#6609,#6609,#5567,.T.);
#8183=EDGE_CURVE('',#6609,#6610,#3896,.T.);
#8184=EDGE_CURVE('',#6610,#6610,#5568,.T.);
#8185=EDGE_CURVE('',#6611,#6606,#3897,.T.);
#8186=EDGE_CURVE('',#6612,#6611,#91,.T.);
#8187=EDGE_CURVE('',#6607,#6612,#3898,.T.);
#8188=EDGE_CURVE('',#6613,#6612,#3899,.T.);
#8189=EDGE_CURVE('',#6608,#6613,#3900,.T.);
#8190=EDGE_CURVE('',#6614,#6613,#92,.T.);
#8191=EDGE_CURVE('',#6529,#6614,#3901,.T.);
#8192=EDGE_CURVE('',#6615,#6614,#5569,.T.);
#8193=EDGE_CURVE('',#6615,#6530,#3902,.T.);
#8194=EDGE_CURVE('',#6616,#6615,#93,.T.);
#8195=EDGE_CURVE('',#6531,#6616,#3903,.T.);
#8196=EDGE_CURVE('',#6617,#6616,#3904,.T.);
#8197=EDGE_CURVE('',#6532,#6617,#3905,.T.);
#8198=EDGE_CURVE('',#6618,#6617,#94,.T.);
#8199=EDGE_CURVE('',#6533,#6618,#3906,.T.);
#8200=EDGE_CURVE('',#6619,#6618,#5570,.T.);
#8201=EDGE_CURVE('',#6619,#6534,#3907,.T.);
#8202=EDGE_CURVE('',#6620,#6619,#95,.T.);
#8203=EDGE_CURVE('',#6535,#6620,#3908,.T.);
#8204=EDGE_CURVE('',#6621,#6620,#3909,.T.);
#8205=EDGE_CURVE('',#6536,#6621,#3910,.T.);
#8206=EDGE_CURVE('',#6622,#6621,#96,.T.);
#8207=EDGE_CURVE('',#6537,#6622,#3911,.T.);
#8208=EDGE_CURVE('',#6623,#6622,#5571,.T.);
#8209=EDGE_CURVE('',#6623,#6538,#3912,.T.);
#8210=EDGE_CURVE('',#6624,#6623,#97,.T.);
#8211=EDGE_CURVE('',#6539,#6624,#3913,.T.);
#8212=EDGE_CURVE('',#6625,#6624,#3914,.T.);
#8213=EDGE_CURVE('',#6540,#6625,#3915,.T.);
#8214=EDGE_CURVE('',#6626,#6625,#98,.T.);
#8215=EDGE_CURVE('',#6541,#6626,#3916,.T.);
#8216=EDGE_CURVE('',#6627,#6626,#5572,.T.);
#8217=EDGE_CURVE('',#6627,#6542,#3917,.T.);
#8218=EDGE_CURVE('',#6628,#6627,#99,.T.);
#8219=EDGE_CURVE('',#6543,#6628,#3918,.T.);
#8220=EDGE_CURVE('',#6629,#6628,#3919,.T.);
#8221=EDGE_CURVE('',#6544,#6629,#3920,.T.);
#8222=EDGE_CURVE('',#6630,#6629,#100,.T.);
#8223=EDGE_CURVE('',#6545,#6630,#3921,.T.);
#8224=EDGE_CURVE('',#6631,#6630,#5573,.T.);
#8225=EDGE_CURVE('',#6631,#6546,#3922,.T.);
#8226=EDGE_CURVE('',#6632,#6631,#101,.T.);
#8227=EDGE_CURVE('',#6547,#6632,#3923,.T.);
#8228=EDGE_CURVE('',#6633,#6632,#3924,.T.);
#8229=EDGE_CURVE('',#6548,#6633,#3925,.T.);
#8230=EDGE_CURVE('',#6634,#6633,#102,.T.);
#8231=EDGE_CURVE('',#6549,#6634,#3926,.T.);
#8232=EDGE_CURVE('',#6635,#6634,#5574,.T.);
#8233=EDGE_CURVE('',#6635,#6550,#3927,.T.);
#8234=EDGE_CURVE('',#6636,#6635,#103,.T.);
#8235=EDGE_CURVE('',#6551,#6636,#3928,.T.);
#8236=EDGE_CURVE('',#6637,#6636,#3929,.T.);
#8237=EDGE_CURVE('',#6552,#6637,#3930,.T.);
#8238=EDGE_CURVE('',#6638,#6637,#104,.T.);
#8239=EDGE_CURVE('',#6553,#6638,#3931,.T.);
#8240=EDGE_CURVE('',#6639,#6638,#5575,.T.);
#8241=EDGE_CURVE('',#6639,#6554,#3932,.T.);
#8242=EDGE_CURVE('',#6640,#6639,#105,.T.);
#8243=EDGE_CURVE('',#6555,#6640,#3933,.T.);
#8244=EDGE_CURVE('',#6641,#6640,#3934,.T.);
#8245=EDGE_CURVE('',#6556,#6641,#3935,.T.);
#8246=EDGE_CURVE('',#6642,#6641,#106,.T.);
#8247=EDGE_CURVE('',#6557,#6642,#3936,.T.);
#8248=EDGE_CURVE('',#6643,#6642,#5576,.T.);
#8249=EDGE_CURVE('',#6643,#6558,#3937,.T.);
#8250=EDGE_CURVE('',#6644,#6643,#107,.T.);
#8251=EDGE_CURVE('',#6559,#6644,#3938,.T.);
#8252=EDGE_CURVE('',#6645,#6644,#3939,.T.);
#8253=EDGE_CURVE('',#6560,#6645,#3940,.T.);
#8254=EDGE_CURVE('',#6646,#6645,#108,.T.);
#8255=EDGE_CURVE('',#6561,#6646,#3941,.T.);
#8256=EDGE_CURVE('',#6647,#6646,#5577,.T.);
#8257=EDGE_CURVE('',#6647,#6562,#3942,.T.);
#8258=EDGE_CURVE('',#6648,#6647,#109,.T.);
#8259=EDGE_CURVE('',#6563,#6648,#3943,.T.);
#8260=EDGE_CURVE('',#6649,#6648,#3944,.T.);
#8261=EDGE_CURVE('',#6564,#6649,#3945,.T.);
#8262=EDGE_CURVE('',#6650,#6649,#110,.T.);
#8263=EDGE_CURVE('',#6565,#6650,#3946,.T.);
#8264=EDGE_CURVE('',#6651,#6650,#5578,.T.);
#8265=EDGE_CURVE('',#6651,#6566,#3947,.T.);
#8266=EDGE_CURVE('',#6652,#6651,#111,.T.);
#8267=EDGE_CURVE('',#6567,#6652,#3948,.T.);
#8268=EDGE_CURVE('',#6653,#6652,#3949,.T.);
#8269=EDGE_CURVE('',#6568,#6653,#3950,.T.);
#8270=EDGE_CURVE('',#6654,#6653,#112,.T.);
#8271=EDGE_CURVE('',#6569,#6654,#3951,.T.);
#8272=EDGE_CURVE('',#6655,#6654,#5579,.T.);
#8273=EDGE_CURVE('',#6655,#6570,#3952,.T.);
#8274=EDGE_CURVE('',#6656,#6655,#113,.T.);
#8275=EDGE_CURVE('',#6571,#6656,#3953,.T.);
#8276=EDGE_CURVE('',#6657,#6656,#3954,.T.);
#8277=EDGE_CURVE('',#6572,#6657,#3955,.T.);
#8278=EDGE_CURVE('',#6658,#6657,#114,.T.);
#8279=EDGE_CURVE('',#6573,#6658,#3956,.T.);
#8280=EDGE_CURVE('',#6659,#6658,#5580,.T.);
#8281=EDGE_CURVE('',#6659,#6574,#3957,.T.);
#8282=EDGE_CURVE('',#6660,#6659,#115,.T.);
#8283=EDGE_CURVE('',#6575,#6660,#3958,.T.);
#8284=EDGE_CURVE('',#6661,#6660,#3959,.T.);
#8285=EDGE_CURVE('',#6576,#6661,#3960,.T.);
#8286=EDGE_CURVE('',#6662,#6661,#116,.T.);
#8287=EDGE_CURVE('',#6577,#6662,#3961,.T.);
#8288=EDGE_CURVE('',#6663,#6662,#5581,.T.);
#8289=EDGE_CURVE('',#6663,#6578,#3962,.T.);
#8290=EDGE_CURVE('',#6664,#6663,#117,.T.);
#8291=EDGE_CURVE('',#6579,#6664,#3963,.T.);
#8292=EDGE_CURVE('',#6665,#6664,#3964,.T.);
#8293=EDGE_CURVE('',#6580,#6665,#3965,.T.);
#8294=EDGE_CURVE('',#6666,#6665,#118,.T.);
#8295=EDGE_CURVE('',#6581,#6666,#3966,.T.);
#8296=EDGE_CURVE('',#6667,#6666,#5582,.T.);
#8297=EDGE_CURVE('',#6667,#6582,#3967,.T.);
#8298=EDGE_CURVE('',#6668,#6667,#119,.T.);
#8299=EDGE_CURVE('',#6583,#6668,#3968,.T.);
#8300=EDGE_CURVE('',#6669,#6668,#3969,.T.);
#8301=EDGE_CURVE('',#6584,#6669,#3970,.T.);
#8302=EDGE_CURVE('',#6670,#6669,#120,.T.);
#8303=EDGE_CURVE('',#6585,#6670,#3971,.T.);
#8304=EDGE_CURVE('',#6671,#6670,#5583,.T.);
#8305=EDGE_CURVE('',#6671,#6586,#3972,.T.);
#8306=EDGE_CURVE('',#6672,#6671,#121,.T.);
#8307=EDGE_CURVE('',#6587,#6672,#3973,.T.);
#8308=EDGE_CURVE('',#6673,#6672,#3974,.T.);
#8309=EDGE_CURVE('',#6588,#6673,#3975,.T.);
#8310=EDGE_CURVE('',#6674,#6673,#122,.T.);
#8311=EDGE_CURVE('',#6589,#6674,#3976,.T.);
#8312=EDGE_CURVE('',#6675,#6674,#5584,.T.);
#8313=EDGE_CURVE('',#6675,#6590,#3977,.T.);
#8314=EDGE_CURVE('',#6676,#6675,#123,.T.);
#8315=EDGE_CURVE('',#6591,#6676,#3978,.T.);
#8316=EDGE_CURVE('',#6677,#6676,#3979,.T.);
#8317=EDGE_CURVE('',#6592,#6677,#3980,.T.);
#8318=EDGE_CURVE('',#6678,#6677,#124,.T.);
#8319=EDGE_CURVE('',#6593,#6678,#3981,.T.);
#8320=EDGE_CURVE('',#6679,#6678,#5585,.T.);
#8321=EDGE_CURVE('',#6679,#6594,#3982,.T.);
#8322=EDGE_CURVE('',#6680,#6679,#125,.T.);
#8323=EDGE_CURVE('',#6595,#6680,#3983,.T.);
#8324=EDGE_CURVE('',#6681,#6680,#3984,.T.);
#8325=EDGE_CURVE('',#6596,#6681,#3985,.T.);
#8326=EDGE_CURVE('',#6682,#6681,#126,.T.);
#8327=EDGE_CURVE('',#6597,#6682,#3986,.T.);
#8328=EDGE_CURVE('',#6683,#6682,#5586,.T.);
#8329=EDGE_CURVE('',#6683,#6598,#3987,.T.);
#8330=EDGE_CURVE('',#6684,#6683,#127,.T.);
#8331=EDGE_CURVE('',#6599,#6684,#3988,.T.);
#8332=EDGE_CURVE('',#6685,#6684,#3989,.T.);
#8333=EDGE_CURVE('',#6600,#6685,#3990,.T.);
#8334=EDGE_CURVE('',#6686,#6685,#128,.T.);
#8335=EDGE_CURVE('',#6601,#6686,#3991,.T.);
#8336=EDGE_CURVE('',#6687,#6686,#5587,.T.);
#8337=EDGE_CURVE('',#6687,#6602,#3992,.T.);
#8338=EDGE_CURVE('',#6688,#6687,#129,.T.);
#8339=EDGE_CURVE('',#6603,#6688,#3993,.T.);
#8340=EDGE_CURVE('',#6689,#6688,#3994,.T.);
#8341=EDGE_CURVE('',#6604,#6689,#3995,.T.);
#8342=EDGE_CURVE('',#6690,#6689,#130,.T.);
#8343=EDGE_CURVE('',#6605,#6690,#3996,.T.);
#8344=EDGE_CURVE('',#6611,#6690,#5588,.T.);
#11123=ORIENTED_EDGE('',*,*,#8090,.F.);
#11124=ORIENTED_EDGE('',*,*,#8091,.F.);
#11125=ORIENTED_EDGE('',*,*,#8092,.F.);
#11126=ORIENTED_EDGE('',*,*,#8093,.F.);
#11127=ORIENTED_EDGE('',*,*,#8094,.F.);
#11128=ORIENTED_EDGE('',*,*,#8095,.T.);
#11129=ORIENTED_EDGE('',*,*,#8096,.F.);
#11130=ORIENTED_EDGE('',*,*,#8091,.T.);
#11131=ORIENTED_EDGE('',*,*,#8097,.F.);
#11132=ORIENTED_EDGE('',*,*,#8098,.F.);
#11133=ORIENTED_EDGE('',*,*,#8099,.F.);
#11134=ORIENTED_EDGE('',*,*,#8095,.F.);
#11135=ORIENTED_EDGE('',*,*,#8100,.T.);
#11136=ORIENTED_EDGE('',*,*,#8101,.T.);
#11137=ORIENTED_EDGE('',*,*,#8102,.T.);
#11138=ORIENTED_EDGE('',*,*,#8103,.T.);
#11139=ORIENTED_EDGE('',*,*,#8104,.T.);
#11140=ORIENTED_EDGE('',*,*,#8105,.T.);
#11141=ORIENTED_EDGE('',*,*,#8106,.T.);
#11142=ORIENTED_EDGE('',*,*,#8107,.T.);
#11143=ORIENTED_EDGE('',*,*,#8108,.T.);
#11144=ORIENTED_EDGE('',*,*,#8109,.T.);
#11145=ORIENTED_EDGE('',*,*,#8110,.T.);
#11146=ORIENTED_EDGE('',*,*,#8111,.T.);
#11147=ORIENTED_EDGE('',*,*,#8112,.T.);
#11148=ORIENTED_EDGE('',*,*,#8113,.T.);
#11149=ORIENTED_EDGE('',*,*,#8114,.T.);
#11150=ORIENTED_EDGE('',*,*,#8115,.T.);
#11151=ORIENTED_EDGE('',*,*,#8116,.T.);
#11152=ORIENTED_EDGE('',*,*,#8117,.T.);
#11153=ORIENTED_EDGE('',*,*,#8118,.T.);
#11154=ORIENTED_EDGE('',*,*,#8119,.T.);
#11155=ORIENTED_EDGE('',*,*,#8120,.T.);
#11156=ORIENTED_EDGE('',*,*,#8121,.T.);
#11157=ORIENTED_EDGE('',*,*,#8122,.T.);
#11158=ORIENTED_EDGE('',*,*,#8123,.T.);
#11159=ORIENTED_EDGE('',*,*,#8124,.T.);
#11160=ORIENTED_EDGE('',*,*,#8125,.T.);
#11161=ORIENTED_EDGE('',*,*,#8126,.T.);
#11162=ORIENTED_EDGE('',*,*,#8127,.T.);
#11163=ORIENTED_EDGE('',*,*,#8128,.T.);
#11164=ORIENTED_EDGE('',*,*,#8129,.T.);
#11165=ORIENTED_EDGE('',*,*,#8130,.T.);
#11166=ORIENTED_EDGE('',*,*,#8131,.T.);
#11167=ORIENTED_EDGE('',*,*,#8132,.T.);
#11168=ORIENTED_EDGE('',*,*,#8133,.T.);
#11169=ORIENTED_EDGE('',*,*,#8134,.T.);
#11170=ORIENTED_EDGE('',*,*,#8135,.T.);
#11171=ORIENTED_EDGE('',*,*,#8136,.T.);
#11172=ORIENTED_EDGE('',*,*,#8137,.T.);
#11173=ORIENTED_EDGE('',*,*,#8138,.T.);
#11174=ORIENTED_EDGE('',*,*,#8139,.T.);
#11175=ORIENTED_EDGE('',*,*,#8140,.T.);
#11176=ORIENTED_EDGE('',*,*,#8141,.T.);
#11177=ORIENTED_EDGE('',*,*,#8142,.T.);
#11178=ORIENTED_EDGE('',*,*,#8143,.T.);
#11179=ORIENTED_EDGE('',*,*,#8144,.T.);
#11180=ORIENTED_EDGE('',*,*,#8145,.T.);
#11181=ORIENTED_EDGE('',*,*,#8146,.T.);
#11182=ORIENTED_EDGE('',*,*,#8147,.T.);
#11183=ORIENTED_EDGE('',*,*,#8148,.T.);
#11184=ORIENTED_EDGE('',*,*,#8149,.T.);
#11185=ORIENTED_EDGE('',*,*,#8150,.T.);
#11186=ORIENTED_EDGE('',*,*,#8151,.T.);
#11187=ORIENTED_EDGE('',*,*,#8152,.T.);
#11188=ORIENTED_EDGE('',*,*,#8153,.T.);
#11189=ORIENTED_EDGE('',*,*,#8154,.T.);
#11190=ORIENTED_EDGE('',*,*,#8155,.T.);
#11191=ORIENTED_EDGE('',*,*,#8156,.T.);
#11192=ORIENTED_EDGE('',*,*,#8157,.T.);
#11193=ORIENTED_EDGE('',*,*,#8158,.T.);
#11194=ORIENTED_EDGE('',*,*,#8159,.T.);
#11195=ORIENTED_EDGE('',*,*,#8160,.T.);
#11196=ORIENTED_EDGE('',*,*,#8161,.T.);
#11197=ORIENTED_EDGE('',*,*,#8162,.T.);
#11198=ORIENTED_EDGE('',*,*,#8163,.T.);
#11199=ORIENTED_EDGE('',*,*,#8164,.T.);
#11200=ORIENTED_EDGE('',*,*,#8165,.T.);
#11201=ORIENTED_EDGE('',*,*,#8166,.T.);
#11202=ORIENTED_EDGE('',*,*,#8167,.T.);
#11203=ORIENTED_EDGE('',*,*,#8168,.T.);
#11204=ORIENTED_EDGE('',*,*,#8169,.T.);
#11205=ORIENTED_EDGE('',*,*,#8170,.T.);
#11206=ORIENTED_EDGE('',*,*,#8171,.T.);
#11207=ORIENTED_EDGE('',*,*,#8172,.T.);
#11208=ORIENTED_EDGE('',*,*,#8173,.T.);
#11209=ORIENTED_EDGE('',*,*,#8174,.T.);
#11210=ORIENTED_EDGE('',*,*,#8175,.T.);
#11211=ORIENTED_EDGE('',*,*,#8176,.T.);
#11212=ORIENTED_EDGE('',*,*,#8177,.T.);
#11213=ORIENTED_EDGE('',*,*,#8178,.T.);
#11214=ORIENTED_EDGE('',*,*,#8179,.T.);
#11215=ORIENTED_EDGE('',*,*,#8092,.T.);
#11216=ORIENTED_EDGE('',*,*,#8096,.T.);
#11217=ORIENTED_EDGE('',*,*,#8099,.T.);
#11218=ORIENTED_EDGE('',*,*,#8180,.T.);
#11219=ORIENTED_EDGE('',*,*,#8093,.T.);
#11220=ORIENTED_EDGE('',*,*,#8180,.F.);
#11221=ORIENTED_EDGE('',*,*,#8098,.T.);
#11222=ORIENTED_EDGE('',*,*,#8181,.F.);
#11223=ORIENTED_EDGE('',*,*,#8182,.F.);
#11224=ORIENTED_EDGE('',*,*,#8183,.T.);
#11225=ORIENTED_EDGE('',*,*,#8184,.F.);
#11226=ORIENTED_EDGE('',*,*,#8183,.F.);
#11227=ORIENTED_EDGE('',*,*,#8182,.T.);
#11228=ORIENTED_EDGE('',*,*,#8090,.T.);
#11229=ORIENTED_EDGE('',*,*,#8181,.T.);
#11230=ORIENTED_EDGE('',*,*,#8097,.T.);
#11231=ORIENTED_EDGE('',*,*,#8094,.T.);
#11232=ORIENTED_EDGE('',*,*,#8185,.F.);
#11233=ORIENTED_EDGE('',*,*,#8186,.F.);
#11234=ORIENTED_EDGE('',*,*,#8187,.F.);
#11235=ORIENTED_EDGE('',*,*,#8177,.F.);
#11236=ORIENTED_EDGE('',*,*,#8187,.T.);
#11237=ORIENTED_EDGE('',*,*,#8188,.F.);
#11238=ORIENTED_EDGE('',*,*,#8189,.F.);
#11239=ORIENTED_EDGE('',*,*,#8178,.F.);
#11240=ORIENTED_EDGE('',*,*,#8189,.T.);
#11241=ORIENTED_EDGE('',*,*,#8190,.F.);
#11242=ORIENTED_EDGE('',*,*,#8191,.F.);
#11243=ORIENTED_EDGE('',*,*,#8179,.F.);
#11244=ORIENTED_EDGE('',*,*,#8191,.T.);
#11245=ORIENTED_EDGE('',*,*,#8192,.F.);
#11246=ORIENTED_EDGE('',*,*,#8193,.T.);
#11247=ORIENTED_EDGE('',*,*,#8100,.F.);
#11248=ORIENTED_EDGE('',*,*,#8193,.F.);
#11249=ORIENTED_EDGE('',*,*,#8194,.F.);
#11250=ORIENTED_EDGE('',*,*,#8195,.F.);
#11251=ORIENTED_EDGE('',*,*,#8101,.F.);
#11252=ORIENTED_EDGE('',*,*,#8195,.T.);
#11253=ORIENTED_EDGE('',*,*,#8196,.F.);
#11254=ORIENTED_EDGE('',*,*,#8197,.F.);
#11255=ORIENTED_EDGE('',*,*,#8102,.F.);
#11256=ORIENTED_EDGE('',*,*,#8197,.T.);
#11257=ORIENTED_EDGE('',*,*,#8198,.F.);
#11258=ORIENTED_EDGE('',*,*,#8199,.F.);
#11259=ORIENTED_EDGE('',*,*,#8103,.F.);
#11260=ORIENTED_EDGE('',*,*,#8199,.T.);
#11261=ORIENTED_EDGE('',*,*,#8200,.F.);
#11262=ORIENTED_EDGE('',*,*,#8201,.T.);
#11263=ORIENTED_EDGE('',*,*,#8104,.F.);
#11264=ORIENTED_EDGE('',*,*,#8201,.F.);
#11265=ORIENTED_EDGE('',*,*,#8202,.F.);
#11266=ORIENTED_EDGE('',*,*,#8203,.F.);
#11267=ORIENTED_EDGE('',*,*,#8105,.F.);
#11268=ORIENTED_EDGE('',*,*,#8203,.T.);
#11269=ORIENTED_EDGE('',*,*,#8204,.F.);
#11270=ORIENTED_EDGE('',*,*,#8205,.F.);
#11271=ORIENTED_EDGE('',*,*,#8106,.F.);
#11272=ORIENTED_EDGE('',*,*,#8205,.T.);
#11273=ORIENTED_EDGE('',*,*,#8206,.F.);
#11274=ORIENTED_EDGE('',*,*,#8207,.F.);
#11275=ORIENTED_EDGE('',*,*,#8107,.F.);
#11276=ORIENTED_EDGE('',*,*,#8207,.T.);
#11277=ORIENTED_EDGE('',*,*,#8208,.F.);
#11278=ORIENTED_EDGE('',*,*,#8209,.T.);
#11279=ORIENTED_EDGE('',*,*,#8108,.F.);
#11280=ORIENTED_EDGE('',*,*,#8209,.F.);
#11281=ORIENTED_EDGE('',*,*,#8210,.F.);
#11282=ORIENTED_EDGE('',*,*,#8211,.F.);
#11283=ORIENTED_EDGE('',*,*,#8109,.F.);
#11284=ORIENTED_EDGE('',*,*,#8211,.T.);
#11285=ORIENTED_EDGE('',*,*,#8212,.F.);
#11286=ORIENTED_EDGE('',*,*,#8213,.F.);
#11287=ORIENTED_EDGE('',*,*,#8110,.F.);
#11288=ORIENTED_EDGE('',*,*,#8213,.T.);
#11289=ORIENTED_EDGE('',*,*,#8214,.F.);
#11290=ORIENTED_EDGE('',*,*,#8215,.F.);
#11291=ORIENTED_EDGE('',*,*,#8111,.F.);
#11292=ORIENTED_EDGE('',*,*,#8215,.T.);
#11293=ORIENTED_EDGE('',*,*,#8216,.F.);
#11294=ORIENTED_EDGE('',*,*,#8217,.T.);
#11295=ORIENTED_EDGE('',*,*,#8112,.F.);
#11296=ORIENTED_EDGE('',*,*,#8217,.F.);
#11297=ORIENTED_EDGE('',*,*,#8218,.F.);
#11298=ORIENTED_EDGE('',*,*,#8219,.F.);
#11299=ORIENTED_EDGE('',*,*,#8113,.F.);
#11300=ORIENTED_EDGE('',*,*,#8219,.T.);
#11301=ORIENTED_EDGE('',*,*,#8220,.F.);
#11302=ORIENTED_EDGE('',*,*,#8221,.F.);
#11303=ORIENTED_EDGE('',*,*,#8114,.F.);
#11304=ORIENTED_EDGE('',*,*,#8221,.T.);
#11305=ORIENTED_EDGE('',*,*,#8222,.F.);
#11306=ORIENTED_EDGE('',*,*,#8223,.F.);
#11307=ORIENTED_EDGE('',*,*,#8115,.F.);
#11308=ORIENTED_EDGE('',*,*,#8223,.T.);
#11309=ORIENTED_EDGE('',*,*,#8224,.F.);
#11310=ORIENTED_EDGE('',*,*,#8225,.T.);
#11311=ORIENTED_EDGE('',*,*,#8116,.F.);
#11312=ORIENTED_EDGE('',*,*,#8225,.F.);
#11313=ORIENTED_EDGE('',*,*,#8226,.F.);
#11314=ORIENTED_EDGE('',*,*,#8227,.F.);
#11315=ORIENTED_EDGE('',*,*,#8117,.F.);
#11316=ORIENTED_EDGE('',*,*,#8227,.T.);
#11317=ORIENTED_EDGE('',*,*,#8228,.F.);
#11318=ORIENTED_EDGE('',*,*,#8229,.F.);
#11319=ORIENTED_EDGE('',*,*,#8118,.F.);
#11320=ORIENTED_EDGE('',*,*,#8229,.T.);
#11321=ORIENTED_EDGE('',*,*,#8230,.F.);
#11322=ORIENTED_EDGE('',*,*,#8231,.F.);
#11323=ORIENTED_EDGE('',*,*,#8119,.F.);
#11324=ORIENTED_EDGE('',*,*,#8231,.T.);
#11325=ORIENTED_EDGE('',*,*,#8232,.F.);
#11326=ORIENTED_EDGE('',*,*,#8233,.T.);
#11327=ORIENTED_EDGE('',*,*,#8120,.F.);
#11328=ORIENTED_EDGE('',*,*,#8233,.F.);
#11329=ORIENTED_EDGE('',*,*,#8234,.F.);
#11330=ORIENTED_EDGE('',*,*,#8235,.F.);
#11331=ORIENTED_EDGE('',*,*,#8121,.F.);
#11332=ORIENTED_EDGE('',*,*,#8235,.T.);
#11333=ORIENTED_EDGE('',*,*,#8236,.F.);
#11334=ORIENTED_EDGE('',*,*,#8237,.F.);
#11335=ORIENTED_EDGE('',*,*,#8122,.F.);
#11336=ORIENTED_EDGE('',*,*,#8237,.T.);
#11337=ORIENTED_EDGE('',*,*,#8238,.F.);
#11338=ORIENTED_EDGE('',*,*,#8239,.F.);
#11339=ORIENTED_EDGE('',*,*,#8123,.F.);
#11340=ORIENTED_EDGE('',*,*,#8239,.T.);
#11341=ORIENTED_EDGE('',*,*,#8240,.F.);
#11342=ORIENTED_EDGE('',*,*,#8241,.T.);
#11343=ORIENTED_EDGE('',*,*,#8124,.F.);
#11344=ORIENTED_EDGE('',*,*,#8241,.F.);
#11345=ORIENTED_EDGE('',*,*,#8242,.F.);
#11346=ORIENTED_EDGE('',*,*,#8243,.F.);
#11347=ORIENTED_EDGE('',*,*,#8125,.F.);
#11348=ORIENTED_EDGE('',*,*,#8243,.T.);
#11349=ORIENTED_EDGE('',*,*,#8244,.F.);
#11350=ORIENTED_EDGE('',*,*,#8245,.F.);
#11351=ORIENTED_EDGE('',*,*,#8126,.F.);
#11352=ORIENTED_EDGE('',*,*,#8245,.T.);
#11353=ORIENTED_EDGE('',*,*,#8246,.F.);
#11354=ORIENTED_EDGE('',*,*,#8247,.F.);
#11355=ORIENTED_EDGE('',*,*,#8127,.F.);
#11356=ORIENTED_EDGE('',*,*,#8247,.T.);
#11357=ORIENTED_EDGE('',*,*,#8248,.F.);
#11358=ORIENTED_EDGE('',*,*,#8249,.T.);
#11359=ORIENTED_EDGE('',*,*,#8128,.F.);
#11360=ORIENTED_EDGE('',*,*,#8249,.F.);
#11361=ORIENTED_EDGE('',*,*,#8250,.F.);
#11362=ORIENTED_EDGE('',*,*,#8251,.F.);
#11363=ORIENTED_EDGE('',*,*,#8129,.F.);
#11364=ORIENTED_EDGE('',*,*,#8251,.T.);
#11365=ORIENTED_EDGE('',*,*,#8252,.F.);
#11366=ORIENTED_EDGE('',*,*,#8253,.F.);
#11367=ORIENTED_EDGE('',*,*,#8130,.F.);
#11368=ORIENTED_EDGE('',*,*,#8253,.T.);
#11369=ORIENTED_EDGE('',*,*,#8254,.F.);
#11370=ORIENTED_EDGE('',*,*,#8255,.F.);
#11371=ORIENTED_EDGE('',*,*,#8131,.F.);
#11372=ORIENTED_EDGE('',*,*,#8255,.T.);
#11373=ORIENTED_EDGE('',*,*,#8256,.F.);
#11374=ORIENTED_EDGE('',*,*,#8257,.T.);
#11375=ORIENTED_EDGE('',*,*,#8132,.F.);
#11376=ORIENTED_EDGE('',*,*,#8257,.F.);
#11377=ORIENTED_EDGE('',*,*,#8258,.F.);
#11378=ORIENTED_EDGE('',*,*,#8259,.F.);
#11379=ORIENTED_EDGE('',*,*,#8133,.F.);
#11380=ORIENTED_EDGE('',*,*,#8259,.T.);
#11381=ORIENTED_EDGE('',*,*,#8260,.F.);
#11382=ORIENTED_EDGE('',*,*,#8261,.F.);
#11383=ORIENTED_EDGE('',*,*,#8134,.F.);
#11384=ORIENTED_EDGE('',*,*,#8261,.T.);
#11385=ORIENTED_EDGE('',*,*,#8262,.F.);
#11386=ORIENTED_EDGE('',*,*,#8263,.F.);
#11387=ORIENTED_EDGE('',*,*,#8135,.F.);
#11388=ORIENTED_EDGE('',*,*,#8263,.T.);
#11389=ORIENTED_EDGE('',*,*,#8264,.F.);
#11390=ORIENTED_EDGE('',*,*,#8265,.T.);
#11391=ORIENTED_EDGE('',*,*,#8136,.F.);
#11392=ORIENTED_EDGE('',*,*,#8265,.F.);
#11393=ORIENTED_EDGE('',*,*,#8266,.F.);
#11394=ORIENTED_EDGE('',*,*,#8267,.F.);
#11395=ORIENTED_EDGE('',*,*,#8137,.F.);
#11396=ORIENTED_EDGE('',*,*,#8267,.T.);
#11397=ORIENTED_EDGE('',*,*,#8268,.F.);
#11398=ORIENTED_EDGE('',*,*,#8269,.F.);
#11399=ORIENTED_EDGE('',*,*,#8138,.F.);
#11400=ORIENTED_EDGE('',*,*,#8269,.T.);
#11401=ORIENTED_EDGE('',*,*,#8270,.F.);
#11402=ORIENTED_EDGE('',*,*,#8271,.F.);
#11403=ORIENTED_EDGE('',*,*,#8139,.F.);
#11404=ORIENTED_EDGE('',*,*,#8271,.T.);
#11405=ORIENTED_EDGE('',*,*,#8272,.F.);
#11406=ORIENTED_EDGE('',*,*,#8273,.T.);
#11407=ORIENTED_EDGE('',*,*,#8140,.F.);
#11408=ORIENTED_EDGE('',*,*,#8273,.F.);
#11409=ORIENTED_EDGE('',*,*,#8274,.F.);
#11410=ORIENTED_EDGE('',*,*,#8275,.F.);
#11411=ORIENTED_EDGE('',*,*,#8141,.F.);
#11412=ORIENTED_EDGE('',*,*,#8275,.T.);
#11413=ORIENTED_EDGE('',*,*,#8276,.F.);
#11414=ORIENTED_EDGE('',*,*,#8277,.F.);
#11415=ORIENTED_EDGE('',*,*,#8142,.F.);
#11416=ORIENTED_EDGE('',*,*,#8277,.T.);
#11417=ORIENTED_EDGE('',*,*,#8278,.F.);
#11418=ORIENTED_EDGE('',*,*,#8279,.F.);
#11419=ORIENTED_EDGE('',*,*,#8143,.F.);
#11420=ORIENTED_EDGE('',*,*,#8279,.T.);
#11421=ORIENTED_EDGE('',*,*,#8280,.F.);
#11422=ORIENTED_EDGE('',*,*,#8281,.T.);
#11423=ORIENTED_EDGE('',*,*,#8144,.F.);
#11424=ORIENTED_EDGE('',*,*,#8281,.F.);
#11425=ORIENTED_EDGE('',*,*,#8282,.F.);
#11426=ORIENTED_EDGE('',*,*,#8283,.F.);
#11427=ORIENTED_EDGE('',*,*,#8145,.F.);
#11428=ORIENTED_EDGE('',*,*,#8283,.T.);
#11429=ORIENTED_EDGE('',*,*,#8284,.F.);
#11430=ORIENTED_EDGE('',*,*,#8285,.F.);
#11431=ORIENTED_EDGE('',*,*,#8146,.F.);
#11432=ORIENTED_EDGE('',*,*,#8285,.T.);
#11433=ORIENTED_EDGE('',*,*,#8286,.F.);
#11434=ORIENTED_EDGE('',*,*,#8287,.F.);
#11435=ORIENTED_EDGE('',*,*,#8147,.F.);
#11436=ORIENTED_EDGE('',*,*,#8287,.T.);
#11437=ORIENTED_EDGE('',*,*,#8288,.F.);
#11438=ORIENTED_EDGE('',*,*,#8289,.T.);
#11439=ORIENTED_EDGE('',*,*,#8148,.F.);
#11440=ORIENTED_EDGE('',*,*,#8289,.F.);
#11441=ORIENTED_EDGE('',*,*,#8290,.F.);
#11442=ORIENTED_EDGE('',*,*,#8291,.F.);
#11443=ORIENTED_EDGE('',*,*,#8149,.F.);
#11444=ORIENTED_EDGE('',*,*,#8291,.T.);
#11445=ORIENTED_EDGE('',*,*,#8292,.F.);
#11446=ORIENTED_EDGE('',*,*,#8293,.F.);
#11447=ORIENTED_EDGE('',*,*,#8150,.F.);
#11448=ORIENTED_EDGE('',*,*,#8293,.T.);
#11449=ORIENTED_EDGE('',*,*,#8294,.F.);
#11450=ORIENTED_EDGE('',*,*,#8295,.F.);
#11451=ORIENTED_EDGE('',*,*,#8151,.F.);
#11452=ORIENTED_EDGE('',*,*,#8295,.T.);
#11453=ORIENTED_EDGE('',*,*,#8296,.F.);
#11454=ORIENTED_EDGE('',*,*,#8297,.T.);
#11455=ORIENTED_EDGE('',*,*,#8152,.F.);
#11456=ORIENTED_EDGE('',*,*,#8297,.F.);
#11457=ORIENTED_EDGE('',*,*,#8298,.F.);
#11458=ORIENTED_EDGE('',*,*,#8299,.F.);
#11459=ORIENTED_EDGE('',*,*,#8153,.F.);
#11460=ORIENTED_EDGE('',*,*,#8299,.T.);
#11461=ORIENTED_EDGE('',*,*,#8300,.F.);
#11462=ORIENTED_EDGE('',*,*,#8301,.F.);
#11463=ORIENTED_EDGE('',*,*,#8154,.F.);
#11464=ORIENTED_EDGE('',*,*,#8301,.T.);
#11465=ORIENTED_EDGE('',*,*,#8302,.F.);
#11466=ORIENTED_EDGE('',*,*,#8303,.F.);
#11467=ORIENTED_EDGE('',*,*,#8155,.F.);
#11468=ORIENTED_EDGE('',*,*,#8303,.T.);
#11469=ORIENTED_EDGE('',*,*,#8304,.F.);
#11470=ORIENTED_EDGE('',*,*,#8305,.T.);
#11471=ORIENTED_EDGE('',*,*,#8156,.F.);
#11472=ORIENTED_EDGE('',*,*,#8305,.F.);
#11473=ORIENTED_EDGE('',*,*,#8306,.F.);
#11474=ORIENTED_EDGE('',*,*,#8307,.F.);
#11475=ORIENTED_EDGE('',*,*,#8157,.F.);
#11476=ORIENTED_EDGE('',*,*,#8307,.T.);
#11477=ORIENTED_EDGE('',*,*,#8308,.F.);
#11478=ORIENTED_EDGE('',*,*,#8309,.F.);
#11479=ORIENTED_EDGE('',*,*,#8158,.F.);
#11480=ORIENTED_EDGE('',*,*,#8309,.T.);
#11481=ORIENTED_EDGE('',*,*,#8310,.F.);
#11482=ORIENTED_EDGE('',*,*,#8311,.F.);
#11483=ORIENTED_EDGE('',*,*,#8159,.F.);
#11484=ORIENTED_EDGE('',*,*,#8311,.T.);
#11485=ORIENTED_EDGE('',*,*,#8312,.F.);
#11486=ORIENTED_EDGE('',*,*,#8313,.T.);
#11487=ORIENTED_EDGE('',*,*,#8160,.F.);
#11488=ORIENTED_EDGE('',*,*,#8313,.F.);
#11489=ORIENTED_EDGE('',*,*,#8314,.F.);
#11490=ORIENTED_EDGE('',*,*,#8315,.F.);
#11491=ORIENTED_EDGE('',*,*,#8161,.F.);
#11492=ORIENTED_EDGE('',*,*,#8315,.T.);
#11493=ORIENTED_EDGE('',*,*,#8316,.F.);
#11494=ORIENTED_EDGE('',*,*,#8317,.F.);
#11495=ORIENTED_EDGE('',*,*,#8162,.F.);
#11496=ORIENTED_EDGE('',*,*,#8317,.T.);
#11497=ORIENTED_EDGE('',*,*,#8318,.F.);
#11498=ORIENTED_EDGE('',*,*,#8319,.F.);
#11499=ORIENTED_EDGE('',*,*,#8163,.F.);
#11500=ORIENTED_EDGE('',*,*,#8319,.T.);
#11501=ORIENTED_EDGE('',*,*,#8320,.F.);
#11502=ORIENTED_EDGE('',*,*,#8321,.T.);
#11503=ORIENTED_EDGE('',*,*,#8164,.F.);
#11504=ORIENTED_EDGE('',*,*,#8321,.F.);
#11505=ORIENTED_EDGE('',*,*,#8322,.F.);
#11506=ORIENTED_EDGE('',*,*,#8323,.F.);
#11507=ORIENTED_EDGE('',*,*,#8165,.F.);
#11508=ORIENTED_EDGE('',*,*,#8323,.T.);
#11509=ORIENTED_EDGE('',*,*,#8324,.F.);
#11510=ORIENTED_EDGE('',*,*,#8325,.F.);
#11511=ORIENTED_EDGE('',*,*,#8166,.F.);
#11512=ORIENTED_EDGE('',*,*,#8325,.T.);
#11513=ORIENTED_EDGE('',*,*,#8326,.F.);
#11514=ORIENTED_EDGE('',*,*,#8327,.F.);
#11515=ORIENTED_EDGE('',*,*,#8167,.F.);
#11516=ORIENTED_EDGE('',*,*,#8327,.T.);
#11517=ORIENTED_EDGE('',*,*,#8328,.F.);
#11518=ORIENTED_EDGE('',*,*,#8329,.T.);
#11519=ORIENTED_EDGE('',*,*,#8168,.F.);
#11520=ORIENTED_EDGE('',*,*,#8329,.F.);
#11521=ORIENTED_EDGE('',*,*,#8330,.F.);
#11522=ORIENTED_EDGE('',*,*,#8331,.F.);
#11523=ORIENTED_EDGE('',*,*,#8169,.F.);
#11524=ORIENTED_EDGE('',*,*,#8331,.T.);
#11525=ORIENTED_EDGE('',*,*,#8332,.F.);
#11526=ORIENTED_EDGE('',*,*,#8333,.F.);
#11527=ORIENTED_EDGE('',*,*,#8170,.F.);
#11528=ORIENTED_EDGE('',*,*,#8333,.T.);
#11529=ORIENTED_EDGE('',*,*,#8334,.F.);
#11530=ORIENTED_EDGE('',*,*,#8335,.F.);
#11531=ORIENTED_EDGE('',*,*,#8171,.F.);
#11532=ORIENTED_EDGE('',*,*,#8335,.T.);
#11533=ORIENTED_EDGE('',*,*,#8336,.F.);
#11534=ORIENTED_EDGE('',*,*,#8337,.T.);
#11535=ORIENTED_EDGE('',*,*,#8172,.F.);
#11536=ORIENTED_EDGE('',*,*,#8337,.F.);
#11537=ORIENTED_EDGE('',*,*,#8338,.F.);
#11538=ORIENTED_EDGE('',*,*,#8339,.F.);
#11539=ORIENTED_EDGE('',*,*,#8173,.F.);
#11540=ORIENTED_EDGE('',*,*,#8339,.T.);
#11541=ORIENTED_EDGE('',*,*,#8340,.F.);
#11542=ORIENTED_EDGE('',*,*,#8341,.F.);
#11543=ORIENTED_EDGE('',*,*,#8174,.F.);
#11544=ORIENTED_EDGE('',*,*,#8341,.T.);
#11545=ORIENTED_EDGE('',*,*,#8342,.F.);
#11546=ORIENTED_EDGE('',*,*,#8343,.F.);
#11547=ORIENTED_EDGE('',*,*,#8175,.F.);
#11548=ORIENTED_EDGE('',*,*,#8344,.T.);
#11549=ORIENTED_EDGE('',*,*,#8342,.T.);
#11550=ORIENTED_EDGE('',*,*,#8340,.T.);
#11551=ORIENTED_EDGE('',*,*,#8338,.T.);
#11552=ORIENTED_EDGE('',*,*,#8336,.T.);
#11553=ORIENTED_EDGE('',*,*,#8334,.T.);
#11554=ORIENTED_EDGE('',*,*,#8332,.T.);
#11555=ORIENTED_EDGE('',*,*,#8330,.T.);
#11556=ORIENTED_EDGE('',*,*,#8328,.T.);
#11557=ORIENTED_EDGE('',*,*,#8326,.T.);
#11558=ORIENTED_EDGE('',*,*,#8324,.T.);
#11559=ORIENTED_EDGE('',*,*,#8322,.T.);
#11560=ORIENTED_EDGE('',*,*,#8320,.T.);
#11561=ORIENTED_EDGE('',*,*,#8318,.T.);
#11562=ORIENTED_EDGE('',*,*,#8316,.T.);
#11563=ORIENTED_EDGE('',*,*,#8314,.T.);
#11564=ORIENTED_EDGE('',*,*,#8312,.T.);
#11565=ORIENTED_EDGE('',*,*,#8310,.T.);
#11566=ORIENTED_EDGE('',*,*,#8308,.T.);
#11567=ORIENTED_EDGE('',*,*,#8306,.T.);
#11568=ORIENTED_EDGE('',*,*,#8304,.T.);
#11569=ORIENTED_EDGE('',*,*,#8302,.T.);
#11570=ORIENTED_EDGE('',*,*,#8300,.T.);
#11571=ORIENTED_EDGE('',*,*,#8298,.T.);
#11572=ORIENTED_EDGE('',*,*,#8296,.T.);
#11573=ORIENTED_EDGE('',*,*,#8294,.T.);
#11574=ORIENTED_EDGE('',*,*,#8292,.T.);
#11575=ORIENTED_EDGE('',*,*,#8290,.T.);
#11576=ORIENTED_EDGE('',*,*,#8288,.T.);
#11577=ORIENTED_EDGE('',*,*,#8286,.T.);
#11578=ORIENTED_EDGE('',*,*,#8284,.T.);
#11579=ORIENTED_EDGE('',*,*,#8282,.T.);
#11580=ORIENTED_EDGE('',*,*,#8280,.T.);
#11581=ORIENTED_EDGE('',*,*,#8278,.T.);
#11582=ORIENTED_EDGE('',*,*,#8276,.T.);
#11583=ORIENTED_EDGE('',*,*,#8274,.T.);
#11584=ORIENTED_EDGE('',*,*,#8272,.T.);
#11585=ORIENTED_EDGE('',*,*,#8270,.T.);
#11586=ORIENTED_EDGE('',*,*,#8268,.T.);
#11587=ORIENTED_EDGE('',*,*,#8266,.T.);
#11588=ORIENTED_EDGE('',*,*,#8264,.T.);
#11589=ORIENTED_EDGE('',*,*,#8262,.T.);
#11590=ORIENTED_EDGE('',*,*,#8260,.T.);
#11591=ORIENTED_EDGE('',*,*,#8258,.T.);
#11592=ORIENTED_EDGE('',*,*,#8256,.T.);
#11593=ORIENTED_EDGE('',*,*,#8254,.T.);
#11594=ORIENTED_EDGE('',*,*,#8252,.T.);
#11595=ORIENTED_EDGE('',*,*,#8250,.T.);
#11596=ORIENTED_EDGE('',*,*,#8248,.T.);
#11597=ORIENTED_EDGE('',*,*,#8246,.T.);
#11598=ORIENTED_EDGE('',*,*,#8244,.T.);
#11599=ORIENTED_EDGE('',*,*,#8242,.T.);
#11600=ORIENTED_EDGE('',*,*,#8240,.T.);
#11601=ORIENTED_EDGE('',*,*,#8238,.T.);
#11602=ORIENTED_EDGE('',*,*,#8236,.T.);
#11603=ORIENTED_EDGE('',*,*,#8234,.T.);
#11604=ORIENTED_EDGE('',*,*,#8232,.T.);
#11605=ORIENTED_EDGE('',*,*,#8230,.T.);
#11606=ORIENTED_EDGE('',*,*,#8228,.T.);
#11607=ORIENTED_EDGE('',*,*,#8226,.T.);
#11608=ORIENTED_EDGE('',*,*,#8224,.T.);
#11609=ORIENTED_EDGE('',*,*,#8222,.T.);
#11610=ORIENTED_EDGE('',*,*,#8220,.T.);
#11611=ORIENTED_EDGE('',*,*,#8218,.T.);
#11612=ORIENTED_EDGE('',*,*,#8216,.T.);
#11613=ORIENTED_EDGE('',*,*,#8214,.T.);
#11614=ORIENTED_EDGE('',*,*,#8212,.T.);
#11615=ORIENTED_EDGE('',*,*,#8210,.T.);
#11616=ORIENTED_EDGE('',*,*,#8208,.T.);
#11617=ORIENTED_EDGE('',*,*,#8206,.T.);
#11618=ORIENTED_EDGE('',*,*,#8204,.T.);
#11619=ORIENTED_EDGE('',*,*,#8202,.T.);
#11620=ORIENTED_EDGE('',*,*,#8200,.T.);
#11621=ORIENTED_EDGE('',*,*,#8198,.T.);
#11622=ORIENTED_EDGE('',*,*,#8196,.T.);
#11623=ORIENTED_EDGE('',*,*,#8194,.T.);
#11624=ORIENTED_EDGE('',*,*,#8192,.T.);
#11625=ORIENTED_EDGE('',*,*,#8190,.T.);
#11626=ORIENTED_EDGE('',*,*,#8188,.T.);
#11627=ORIENTED_EDGE('',*,*,#8186,.T.);
#11628=ORIENTED_EDGE('',*,*,#8184,.T.);
#11629=ORIENTED_EDGE('',*,*,#8185,.T.);
#11630=ORIENTED_EDGE('',*,*,#8176,.F.);
#11631=ORIENTED_EDGE('',*,*,#8343,.T.);
#11632=ORIENTED_EDGE('',*,*,#8344,.F.);
#11918=CYLINDRICAL_SURFACE('',#14160,0.6);
#11919=CYLINDRICAL_SURFACE('',#14162,1.4);
#11920=CYLINDRICAL_SURFACE('',#14167,1.75);
#11921=CYLINDRICAL_SURFACE('',#14170,1.75);
#11922=CYLINDRICAL_SURFACE('',#14173,1.75);
#11923=CYLINDRICAL_SURFACE('',#14176,1.75);
#11924=CYLINDRICAL_SURFACE('',#14179,1.75);
#11925=CYLINDRICAL_SURFACE('',#14182,1.75);
#11926=CYLINDRICAL_SURFACE('',#14185,1.75);
#11927=CYLINDRICAL_SURFACE('',#14188,1.75);
#11928=CYLINDRICAL_SURFACE('',#14191,1.75);
#11929=CYLINDRICAL_SURFACE('',#14194,1.75);
#11930=CYLINDRICAL_SURFACE('',#14197,1.75);
#11931=CYLINDRICAL_SURFACE('',#14200,1.75);
#11932=CYLINDRICAL_SURFACE('',#14203,1.75);
#11933=CYLINDRICAL_SURFACE('',#14206,1.75);
#11934=CYLINDRICAL_SURFACE('',#14209,1.75);
#11935=CYLINDRICAL_SURFACE('',#14212,1.75);
#11936=CYLINDRICAL_SURFACE('',#14215,1.75);
#11937=CYLINDRICAL_SURFACE('',#14218,1.75);
#11938=CYLINDRICAL_SURFACE('',#14221,1.75);
#11939=CYLINDRICAL_SURFACE('',#14226,1.75);
#12507=ADVANCED_FACE('',(#1898),#1287,.F.);
#12508=ADVANCED_FACE('',(#1899),#1288,.F.);
#12509=ADVANCED_FACE('',(#1900),#1289,.F.);
#12510=ADVANCED_FACE('',(#1901,#878),#1290,.F.);
#12511=ADVANCED_FACE('',(#1902),#11918,.F.);
#12512=ADVANCED_FACE('',(#1903),#11919,.T.);
#12513=ADVANCED_FACE('',(#1904,#879),#1291,.T.);
#12514=ADVANCED_FACE('',(#1905),#11,.T.);
#12515=ADVANCED_FACE('',(#1906),#1292,.T.);
#12516=ADVANCED_FACE('',(#1907),#12,.T.);
#12517=ADVANCED_FACE('',(#1908),#11920,.T.);
#12518=ADVANCED_FACE('',(#1909),#13,.T.);
#12519=ADVANCED_FACE('',(#1910),#1293,.T.);
#12520=ADVANCED_FACE('',(#1911),#14,.T.);
#12521=ADVANCED_FACE('',(#1912),#11921,.T.);
#12522=ADVANCED_FACE('',(#1913),#15,.T.);
#12523=ADVANCED_FACE('',(#1914),#1294,.T.);
#12524=ADVANCED_FACE('',(#1915),#16,.T.);
#12525=ADVANCED_FACE('',(#1916),#11922,.T.);
#12526=ADVANCED_FACE('',(#1917),#17,.T.);
#12527=ADVANCED_FACE('',(#1918),#1295,.T.);
#12528=ADVANCED_FACE('',(#1919),#18,.T.);
#12529=ADVANCED_FACE('',(#1920),#11923,.T.);
#12530=ADVANCED_FACE('',(#1921),#19,.T.);
#12531=ADVANCED_FACE('',(#1922),#1296,.T.);
#12532=ADVANCED_FACE('',(#1923),#20,.T.);
#12533=ADVANCED_FACE('',(#1924),#11924,.T.);
#12534=ADVANCED_FACE('',(#1925),#21,.T.);
#12535=ADVANCED_FACE('',(#1926),#1297,.T.);
#12536=ADVANCED_FACE('',(#1927),#22,.T.);
#12537=ADVANCED_FACE('',(#1928),#11925,.T.);
#12538=ADVANCED_FACE('',(#1929),#23,.T.);
#12539=ADVANCED_FACE('',(#1930),#1298,.T.);
#12540=ADVANCED_FACE('',(#1931),#24,.T.);
#12541=ADVANCED_FACE('',(#1932),#11926,.T.);
#12542=ADVANCED_FACE('',(#1933),#25,.T.);
#12543=ADVANCED_FACE('',(#1934),#1299,.T.);
#12544=ADVANCED_FACE('',(#1935),#26,.T.);
#12545=ADVANCED_FACE('',(#1936),#11927,.T.);
#12546=ADVANCED_FACE('',(#1937),#27,.T.);
#12547=ADVANCED_FACE('',(#1938),#1300,.T.);
#12548=ADVANCED_FACE('',(#1939),#28,.T.);
#12549=ADVANCED_FACE('',(#1940),#11928,.T.);
#12550=ADVANCED_FACE('',(#1941),#29,.T.);
#12551=ADVANCED_FACE('',(#1942),#1301,.T.);
#12552=ADVANCED_FACE('',(#1943),#30,.T.);
#12553=ADVANCED_FACE('',(#1944),#11929,.T.);
#12554=ADVANCED_FACE('',(#1945),#31,.T.);
#12555=ADVANCED_FACE('',(#1946),#1302,.T.);
#12556=ADVANCED_FACE('',(#1947),#32,.T.);
#12557=ADVANCED_FACE('',(#1948),#11930,.T.);
#12558=ADVANCED_FACE('',(#1949),#33,.T.);
#12559=ADVANCED_FACE('',(#1950),#1303,.T.);
#12560=ADVANCED_FACE('',(#1951),#34,.T.);
#12561=ADVANCED_FACE('',(#1952),#11931,.T.);
#12562=ADVANCED_FACE('',(#1953),#35,.T.);
#12563=ADVANCED_FACE('',(#1954),#1304,.T.);
#12564=ADVANCED_FACE('',(#1955),#36,.T.);
#12565=ADVANCED_FACE('',(#1956),#11932,.T.);
#12566=ADVANCED_FACE('',(#1957),#37,.T.);
#12567=ADVANCED_FACE('',(#1958),#1305,.T.);
#12568=ADVANCED_FACE('',(#1959),#38,.T.);
#12569=ADVANCED_FACE('',(#1960),#11933,.T.);
#12570=ADVANCED_FACE('',(#1961),#39,.T.);
#12571=ADVANCED_FACE('',(#1962),#1306,.T.);
#12572=ADVANCED_FACE('',(#1963),#40,.T.);
#12573=ADVANCED_FACE('',(#1964),#11934,.T.);
#12574=ADVANCED_FACE('',(#1965),#41,.T.);
#12575=ADVANCED_FACE('',(#1966),#1307,.T.);
#12576=ADVANCED_FACE('',(#1967),#42,.T.);
#12577=ADVANCED_FACE('',(#1968),#11935,.T.);
#12578=ADVANCED_FACE('',(#1969),#43,.T.);
#12579=ADVANCED_FACE('',(#1970),#1308,.T.);
#12580=ADVANCED_FACE('',(#1971),#44,.T.);
#12581=ADVANCED_FACE('',(#1972),#11936,.T.);
#12582=ADVANCED_FACE('',(#1973),#45,.T.);
#12583=ADVANCED_FACE('',(#1974),#1309,.T.);
#12584=ADVANCED_FACE('',(#1975),#46,.T.);
#12585=ADVANCED_FACE('',(#1976),#11937,.T.);
#12586=ADVANCED_FACE('',(#1977),#47,.T.);
#12587=ADVANCED_FACE('',(#1978),#1310,.T.);
#12588=ADVANCED_FACE('',(#1979),#48,.T.);
#12589=ADVANCED_FACE('',(#1980),#11938,.T.);
#12590=ADVANCED_FACE('',(#1981),#49,.T.);
#12591=ADVANCED_FACE('',(#1982),#1311,.T.);
#12592=ADVANCED_FACE('',(#1983),#50,.T.);
#12593=ADVANCED_FACE('',(#1984,#880),#1312,.T.);
#12594=ADVANCED_FACE('',(#1985),#11939,.T.);
#12685=CLOSED_SHELL('',(#12507,#12508,#12509,#12510,#12511,#12512,#12513,
#12514,#12515,#12516,#12517,#12518,#12519,#12520,#12521,#12522,#12523,#12524,
#12525,#12526,#12527,#12528,#12529,#12530,#12531,#12532,#12533,#12534,#12535,
#12536,#12537,#12538,#12539,#12540,#12541,#12542,#12543,#12544,#12545,#12546,
#12547,#12548,#12549,#12550,#12551,#12552,#12553,#12554,#12555,#12556,#12557,
#12558,#12559,#12560,#12561,#12562,#12563,#12564,#12565,#12566,#12567,#12568,
#12569,#12570,#12571,#12572,#12573,#12574,#12575,#12576,#12577,#12578,#12579,
#12580,#12581,#12582,#12583,#12584,#12585,#12586,#12587,#12588,#12589,#12590,
#12591,#12592,#12593,#12594));
#14134=AXIS2_PLACEMENT_3D('',#21362,#17241,#17242);
#14135=AXIS2_PLACEMENT_3D('',#21363,#17243,#17244);
#14136=AXIS2_PLACEMENT_3D('',#21372,#17249,#17250);
#14137=AXIS2_PLACEMENT_3D('',#21378,#17254,#17255);
#14138=AXIS2_PLACEMENT_3D('',#21384,#17259,#17260);
#14139=AXIS2_PLACEMENT_3D('',#21387,#17261,#17262);
#14140=AXIS2_PLACEMENT_3D('',#21533,#17264,#17265);
#14141=AXIS2_PLACEMENT_3D('',#21679,#17267,#17268);
#14142=AXIS2_PLACEMENT_3D('',#21825,#17270,#17271);
#14143=AXIS2_PLACEMENT_3D('',#21971,#17273,#17274);
#14144=AXIS2_PLACEMENT_3D('',#22117,#17276,#17277);
#14145=AXIS2_PLACEMENT_3D('',#22263,#17279,#17280);
#14146=AXIS2_PLACEMENT_3D('',#22409,#17282,#17283);
#14147=AXIS2_PLACEMENT_3D('',#22555,#17285,#17286);
#14148=AXIS2_PLACEMENT_3D('',#22701,#17288,#17289);
#14149=AXIS2_PLACEMENT_3D('',#22847,#17291,#17292);
#14150=AXIS2_PLACEMENT_3D('',#22993,#17294,#17295);
#14151=AXIS2_PLACEMENT_3D('',#23139,#17297,#17298);
#14152=AXIS2_PLACEMENT_3D('',#23285,#17300,#17301);
#14153=AXIS2_PLACEMENT_3D('',#23431,#17303,#17304);
#14154=AXIS2_PLACEMENT_3D('',#23577,#17306,#17307);
#14155=AXIS2_PLACEMENT_3D('',#23723,#17309,#17310);
#14156=AXIS2_PLACEMENT_3D('',#23869,#17312,#17313);
#14157=AXIS2_PLACEMENT_3D('',#24015,#17315,#17316);
#14158=AXIS2_PLACEMENT_3D('',#24161,#17318,#17319);
#14159=AXIS2_PLACEMENT_3D('',#24305,#17321,#17322);
#14160=AXIS2_PLACEMENT_3D('',#24306,#17323,#17324);
#14161=AXIS2_PLACEMENT_3D('',#24307,#17325,#17326);
#14162=AXIS2_PLACEMENT_3D('',#24308,#17327,#17328);
#14163=AXIS2_PLACEMENT_3D('',#24310,#17329,#17330);
#14164=AXIS2_PLACEMENT_3D('',#24313,#17332,#17333);
#14165=AXIS2_PLACEMENT_3D('',#24314,#17334,#17335);
#14166=AXIS2_PLACEMENT_3D('',#24529,#17338,#17339);
#14167=AXIS2_PLACEMENT_3D('',#24745,#17343,#17344);
#14168=AXIS2_PLACEMENT_3D('',#24747,#17345,#17346);
#14169=AXIS2_PLACEMENT_3D('',#24961,#17349,#17350);
#14170=AXIS2_PLACEMENT_3D('',#25177,#17354,#17355);
#14171=AXIS2_PLACEMENT_3D('',#25179,#17356,#17357);
#14172=AXIS2_PLACEMENT_3D('',#25393,#17360,#17361);
#14173=AXIS2_PLACEMENT_3D('',#25609,#17365,#17366);
#14174=AXIS2_PLACEMENT_3D('',#25611,#17367,#17368);
#14175=AXIS2_PLACEMENT_3D('',#25825,#17371,#17372);
#14176=AXIS2_PLACEMENT_3D('',#26041,#17376,#17377);
#14177=AXIS2_PLACEMENT_3D('',#26043,#17378,#17379);
#14178=AXIS2_PLACEMENT_3D('',#26257,#17382,#17383);
#14179=AXIS2_PLACEMENT_3D('',#26473,#17387,#17388);
#14180=AXIS2_PLACEMENT_3D('',#26475,#17389,#17390);
#14181=AXIS2_PLACEMENT_3D('',#26689,#17393,#17394);
#14182=AXIS2_PLACEMENT_3D('',#26905,#17398,#17399);
#14183=AXIS2_PLACEMENT_3D('',#26907,#17400,#17401);
#14184=AXIS2_PLACEMENT_3D('',#27121,#17404,#17405);
#14185=AXIS2_PLACEMENT_3D('',#27337,#17409,#17410);
#14186=AXIS2_PLACEMENT_3D('',#27339,#17411,#17412);
#14187=AXIS2_PLACEMENT_3D('',#27553,#17415,#17416);
#14188=AXIS2_PLACEMENT_3D('',#27769,#17420,#17421);
#14189=AXIS2_PLACEMENT_3D('',#27771,#17422,#17423);
#14190=AXIS2_PLACEMENT_3D('',#27985,#17426,#17427);
#14191=AXIS2_PLACEMENT_3D('',#28201,#17431,#17432);
#14192=AXIS2_PLACEMENT_3D('',#28203,#17433,#17434);
#14193=AXIS2_PLACEMENT_3D('',#28417,#17437,#17438);
#14194=AXIS2_PLACEMENT_3D('',#28633,#17442,#17443);
#14195=AXIS2_PLACEMENT_3D('',#28635,#17444,#17445);
#14196=AXIS2_PLACEMENT_3D('',#28849,#17448,#17449);
#14197=AXIS2_PLACEMENT_3D('',#29065,#17453,#17454);
#14198=AXIS2_PLACEMENT_3D('',#29067,#17455,#17456);
#14199=AXIS2_PLACEMENT_3D('',#29281,#17459,#17460);
#14200=AXIS2_PLACEMENT_3D('',#29497,#17464,#17465);
#14201=AXIS2_PLACEMENT_3D('',#29499,#17466,#17467);
#14202=AXIS2_PLACEMENT_3D('',#29713,#17470,#17471);
#14203=AXIS2_PLACEMENT_3D('',#29929,#17475,#17476);
#14204=AXIS2_PLACEMENT_3D('',#29931,#17477,#17478);
#14205=AXIS2_PLACEMENT_3D('',#30145,#17481,#17482);
#14206=AXIS2_PLACEMENT_3D('',#30361,#17486,#17487);
#14207=AXIS2_PLACEMENT_3D('',#30363,#17488,#17489);
#14208=AXIS2_PLACEMENT_3D('',#30577,#17492,#17493);
#14209=AXIS2_PLACEMENT_3D('',#30793,#17497,#17498);
#14210=AXIS2_PLACEMENT_3D('',#30795,#17499,#17500);
#14211=AXIS2_PLACEMENT_3D('',#31009,#17503,#17504);
#14212=AXIS2_PLACEMENT_3D('',#31225,#17508,#17509);
#14213=AXIS2_PLACEMENT_3D('',#31227,#17510,#17511);
#14214=AXIS2_PLACEMENT_3D('',#31441,#17514,#17515);
#14215=AXIS2_PLACEMENT_3D('',#31657,#17519,#17520);
#14216=AXIS2_PLACEMENT_3D('',#31659,#17521,#17522);
#14217=AXIS2_PLACEMENT_3D('',#31873,#17525,#17526);
#14218=AXIS2_PLACEMENT_3D('',#32089,#17530,#17531);
#14219=AXIS2_PLACEMENT_3D('',#32091,#17532,#17533);
#14220=AXIS2_PLACEMENT_3D('',#32305,#17536,#17537);
#14221=AXIS2_PLACEMENT_3D('',#32521,#17541,#17542);
#14222=AXIS2_PLACEMENT_3D('',#32523,#17543,#17544);
#14223=AXIS2_PLACEMENT_3D('',#32737,#17547,#17548);
#14224=AXIS2_PLACEMENT_3D('',#32953,#17552,#17553);
#14225=AXIS2_PLACEMENT_3D('',#32954,#17554,#17555);
#14226=AXIS2_PLACEMENT_3D('',#32955,#17556,#17557);
#17241=DIRECTION('axis',(0.,0.,1.));
#17242=DIRECTION('refdir',(1.,0.,0.));
#17243=DIRECTION('center_axis',(1.,0.,0.));
#17244=DIRECTION('ref_axis',(0.,0.,-1.));
#17245=DIRECTION('',(0.,0.,1.));
#17246=DIRECTION('',(0.,1.,0.));
#17247=DIRECTION('',(0.,0.,-1.));
#17248=DIRECTION('',(0.,-1.,0.));
#17249=DIRECTION('center_axis',(0.,0.,-1.));
#17250=DIRECTION('ref_axis',(-1.,0.,0.));
#17251=DIRECTION('',(1.,0.,0.));
#17252=DIRECTION('',(0.,-1.,0.));
#17253=DIRECTION('',(-1.,0.,0.));
#17254=DIRECTION('center_axis',(-1.,0.,0.));
#17255=DIRECTION('ref_axis',(0.,0.,1.));
#17256=DIRECTION('',(0.,0.,-1.));
#17257=DIRECTION('',(0.,1.,0.));
#17258=DIRECTION('',(0.,0.,1.));
#17259=DIRECTION('center_axis',(0.,1.,0.));
#17260=DIRECTION('ref_axis',(1.,0.,0.));
#17261=DIRECTION('center_axis',(0.,-1.,0.));
#17262=DIRECTION('ref_axis',(1.,0.,0.));
#17263=DIRECTION('',(-0.587785252292473,0.,0.809016994374947));
#17264=DIRECTION('center_axis',(0.,-1.,0.));
#17265=DIRECTION('ref_axis',(1.,0.,0.));
#17266=DIRECTION('',(-0.809016994374948,0.,0.587785252292473));
#17267=DIRECTION('center_axis',(0.,-1.,0.));
#17268=DIRECTION('ref_axis',(1.,0.,0.));
#17269=DIRECTION('',(-0.951056516295154,0.,0.309016994374947));
#17270=DIRECTION('center_axis',(0.,-1.,0.));
#17271=DIRECTION('ref_axis',(1.,0.,0.));
#17272=DIRECTION('',(-1.,0.,-1.83697019872103E-16));
#17273=DIRECTION('center_axis',(0.,-1.,0.));
#17274=DIRECTION('ref_axis',(1.,0.,0.));
#17275=DIRECTION('',(-0.951056516295154,0.,-0.309016994374948));
#17276=DIRECTION('center_axis',(0.,-1.,0.));
#17277=DIRECTION('ref_axis',(1.,0.,0.));
#17278=DIRECTION('',(-0.809016994374947,0.,-0.587785252292473));
#17279=DIRECTION('center_axis',(0.,-1.,0.));
#17280=DIRECTION('ref_axis',(1.,0.,0.));
#17281=DIRECTION('',(-0.587785252292473,0.,-0.809016994374948));
#17282=DIRECTION('center_axis',(0.,-1.,0.));
#17283=DIRECTION('ref_axis',(1.,0.,0.));
#17284=DIRECTION('',(-0.309016994374947,0.,-0.951056516295154));
#17285=DIRECTION('center_axis',(0.,-1.,0.));
#17286=DIRECTION('ref_axis',(1.,0.,0.));
#17287=DIRECTION('',(1.22464679914735E-16,0.,-1.));
#17288=DIRECTION('center_axis',(0.,-1.,0.));
#17289=DIRECTION('ref_axis',(1.,0.,0.));
#17290=DIRECTION('',(0.309016994374948,0.,-0.951056516295154));
#17291=DIRECTION('center_axis',(0.,-1.,0.));
#17292=DIRECTION('ref_axis',(1.,0.,0.));
#17293=DIRECTION('',(0.587785252292473,0.,-0.809016994374947));
#17294=DIRECTION('center_axis',(0.,-1.,0.));
#17295=DIRECTION('ref_axis',(1.,0.,0.));
#17296=DIRECTION('',(0.809016994374948,0.,-0.587785252292473));
#17297=DIRECTION('center_axis',(0.,-1.,0.));
#17298=DIRECTION('ref_axis',(1.,0.,0.));
#17299=DIRECTION('',(0.951056516295154,0.,-0.309016994374947));
#17300=DIRECTION('center_axis',(0.,-1.,0.));
#17301=DIRECTION('ref_axis',(1.,0.,0.));
#17302=DIRECTION('',(1.,0.,6.12323399573677E-17));
#17303=DIRECTION('center_axis',(0.,-1.,0.));
#17304=DIRECTION('ref_axis',(1.,0.,0.));
#17305=DIRECTION('',(0.951056516295154,0.,0.309016994374948));
#17306=DIRECTION('center_axis',(0.,-1.,0.));
#17307=DIRECTION('ref_axis',(1.,0.,0.));
#17308=DIRECTION('',(0.809016994374947,0.,0.587785252292473));
#17309=DIRECTION('center_axis',(0.,-1.,0.));
#17310=DIRECTION('ref_axis',(1.,0.,0.));
#17311=DIRECTION('',(0.587785252292473,0.,0.809016994374947));
#17312=DIRECTION('center_axis',(0.,-1.,0.));
#17313=DIRECTION('ref_axis',(1.,0.,0.));
#17314=DIRECTION('',(0.309016994374947,0.,0.951056516295154));
#17315=DIRECTION('center_axis',(0.,-1.,0.));
#17316=DIRECTION('ref_axis',(1.,0.,0.));
#17317=DIRECTION('',(0.,0.,1.));
#17318=DIRECTION('center_axis',(0.,-1.,0.));
#17319=DIRECTION('ref_axis',(1.,0.,0.));
#17320=DIRECTION('',(-0.309016994374948,0.,0.951056516295154));
#17321=DIRECTION('center_axis',(0.,1.,0.));
#17322=DIRECTION('ref_axis',(1.,0.,0.));
#17323=DIRECTION('center_axis',(0.,1.,0.));
#17324=DIRECTION('ref_axis',(6.12323399573677E-17,0.,1.));
#17325=DIRECTION('center_axis',(0.,-1.,0.));
#17326=DIRECTION('ref_axis',(1.,0.,0.));
#17327=DIRECTION('center_axis',(0.,1.,0.));
#17328=DIRECTION('ref_axis',(1.,0.,0.));
#17329=DIRECTION('center_axis',(0.,1.,0.));
#17330=DIRECTION('ref_axis',(1.,0.,0.));
#17331=DIRECTION('',(0.,-1.,0.));
#17332=DIRECTION('center_axis',(0.,-1.,0.));
#17333=DIRECTION('ref_axis',(1.,0.,0.));
#17334=DIRECTION('center_axis',(0.,1.,0.));
#17335=DIRECTION('ref_axis',(1.,0.,0.));
#17336=DIRECTION('',(0.,-1.,0.));
#17337=DIRECTION('',(0.,1.,0.));
#17338=DIRECTION('center_axis',(0.951056516295154,0.,0.309016994374948));
#17339=DIRECTION('ref_axis',(0.309016994374948,0.,-0.951056516295154));
#17340=DIRECTION('',(0.309016994374948,0.,-0.951056516295154));
#17341=DIRECTION('',(0.,1.,0.));
#17342=DIRECTION('',(0.,1.,0.));
#17343=DIRECTION('center_axis',(0.,1.,0.));
#17344=DIRECTION('ref_axis',(1.,0.,0.));
#17345=DIRECTION('center_axis',(0.,1.,0.));
#17346=DIRECTION('ref_axis',(1.,0.,0.));
#17347=DIRECTION('',(0.,-1.,0.));
#17348=DIRECTION('',(0.,1.,0.));
#17349=DIRECTION('center_axis',(0.809016994374947,0.,0.587785252292473));
#17350=DIRECTION('ref_axis',(0.587785252292473,0.,-0.809016994374947));
#17351=DIRECTION('',(0.587785252292473,0.,-0.809016994374947));
#17352=DIRECTION('',(0.,1.,0.));
#17353=DIRECTION('',(0.,1.,0.));
#17354=DIRECTION('center_axis',(0.,1.,0.));
#17355=DIRECTION('ref_axis',(1.,0.,0.));
#17356=DIRECTION('center_axis',(0.,1.,0.));
#17357=DIRECTION('ref_axis',(1.,0.,0.));
#17358=DIRECTION('',(0.,-1.,0.));
#17359=DIRECTION('',(0.,1.,0.));
#17360=DIRECTION('center_axis',(0.587785252292473,0.,0.809016994374948));
#17361=DIRECTION('ref_axis',(0.809016994374948,0.,-0.587785252292473));
#17362=DIRECTION('',(0.809016994374948,0.,-0.587785252292473));
#17363=DIRECTION('',(0.,1.,0.));
#17364=DIRECTION('',(0.,1.,0.));
#17365=DIRECTION('center_axis',(0.,1.,0.));
#17366=DIRECTION('ref_axis',(1.,0.,0.));
#17367=DIRECTION('center_axis',(0.,1.,0.));
#17368=DIRECTION('ref_axis',(1.,0.,0.));
#17369=DIRECTION('',(0.,-1.,0.));
#17370=DIRECTION('',(0.,1.,0.));
#17371=DIRECTION('center_axis',(0.309016994374947,0.,0.951056516295154));
#17372=DIRECTION('ref_axis',(0.951056516295154,0.,-0.309016994374947));
#17373=DIRECTION('',(0.951056516295154,0.,-0.309016994374947));
#17374=DIRECTION('',(0.,1.,0.));
#17375=DIRECTION('',(0.,1.,0.));
#17376=DIRECTION('center_axis',(0.,1.,0.));
#17377=DIRECTION('ref_axis',(1.,0.,0.));
#17378=DIRECTION('center_axis',(0.,1.,0.));
#17379=DIRECTION('ref_axis',(1.,0.,0.));
#17380=DIRECTION('',(0.,-1.,0.));
#17381=DIRECTION('',(0.,1.,0.));
#17382=DIRECTION('center_axis',(-1.83697019872103E-16,0.,1.));
#17383=DIRECTION('ref_axis',(1.,0.,1.83697019872103E-16));
#17384=DIRECTION('',(1.,0.,1.83697019872103E-16));
#17385=DIRECTION('',(0.,1.,0.));
#17386=DIRECTION('',(0.,1.,0.));
#17387=DIRECTION('center_axis',(0.,1.,0.));
#17388=DIRECTION('ref_axis',(1.,0.,0.));
#17389=DIRECTION('center_axis',(0.,1.,0.));
#17390=DIRECTION('ref_axis',(1.,0.,0.));
#17391=DIRECTION('',(0.,-1.,0.));
#17392=DIRECTION('',(0.,1.,0.));
#17393=DIRECTION('center_axis',(-0.309016994374948,0.,0.951056516295154));
#17394=DIRECTION('ref_axis',(0.951056516295154,0.,0.309016994374948));
#17395=DIRECTION('',(0.951056516295154,0.,0.309016994374948));
#17396=DIRECTION('',(0.,1.,0.));
#17397=DIRECTION('',(0.,1.,0.));
#17398=DIRECTION('center_axis',(0.,1.,0.));
#17399=DIRECTION('ref_axis',(1.,0.,0.));
#17400=DIRECTION('center_axis',(0.,1.,0.));
#17401=DIRECTION('ref_axis',(1.,0.,0.));
#17402=DIRECTION('',(0.,-1.,0.));
#17403=DIRECTION('',(0.,1.,0.));
#17404=DIRECTION('center_axis',(-0.587785252292473,0.,0.809016994374947));
#17405=DIRECTION('ref_axis',(0.809016994374947,0.,0.587785252292473));
#17406=DIRECTION('',(0.809016994374947,0.,0.587785252292473));
#17407=DIRECTION('',(0.,1.,0.));
#17408=DIRECTION('',(0.,1.,0.));
#17409=DIRECTION('center_axis',(0.,1.,0.));
#17410=DIRECTION('ref_axis',(1.,0.,0.));
#17411=DIRECTION('center_axis',(0.,1.,0.));
#17412=DIRECTION('ref_axis',(1.,0.,0.));
#17413=DIRECTION('',(0.,-1.,0.));
#17414=DIRECTION('',(0.,1.,0.));
#17415=DIRECTION('center_axis',(-0.809016994374948,0.,0.587785252292473));
#17416=DIRECTION('ref_axis',(0.587785252292473,0.,0.809016994374948));
#17417=DIRECTION('',(0.587785252292473,0.,0.809016994374948));
#17418=DIRECTION('',(0.,1.,0.));
#17419=DIRECTION('',(0.,1.,0.));
#17420=DIRECTION('center_axis',(0.,1.,0.));
#17421=DIRECTION('ref_axis',(1.,0.,0.));
#17422=DIRECTION('center_axis',(0.,1.,0.));
#17423=DIRECTION('ref_axis',(1.,0.,0.));
#17424=DIRECTION('',(0.,-1.,0.));
#17425=DIRECTION('',(0.,1.,0.));
#17426=DIRECTION('center_axis',(-0.951056516295154,0.,0.309016994374947));
#17427=DIRECTION('ref_axis',(0.309016994374947,0.,0.951056516295154));
#17428=DIRECTION('',(0.309016994374947,0.,0.951056516295154));
#17429=DIRECTION('',(0.,1.,0.));
#17430=DIRECTION('',(0.,1.,0.));
#17431=DIRECTION('center_axis',(0.,1.,0.));
#17432=DIRECTION('ref_axis',(1.,0.,0.));
#17433=DIRECTION('center_axis',(0.,1.,0.));
#17434=DIRECTION('ref_axis',(1.,0.,0.));
#17435=DIRECTION('',(0.,-1.,0.));
#17436=DIRECTION('',(0.,1.,0.));
#17437=DIRECTION('center_axis',(-1.,0.,-1.22464679914735E-16));
#17438=DIRECTION('ref_axis',(-1.22464679914735E-16,0.,1.));
#17439=DIRECTION('',(-1.22464679914735E-16,0.,1.));
#17440=DIRECTION('',(0.,1.,0.));
#17441=DIRECTION('',(0.,1.,0.));
#17442=DIRECTION('center_axis',(0.,1.,0.));
#17443=DIRECTION('ref_axis',(1.,0.,0.));
#17444=DIRECTION('center_axis',(0.,1.,0.));
#17445=DIRECTION('ref_axis',(1.,0.,0.));
#17446=DIRECTION('',(0.,-1.,0.));
#17447=DIRECTION('',(0.,1.,0.));
#17448=DIRECTION('center_axis',(-0.951056516295154,0.,-0.309016994374948));
#17449=DIRECTION('ref_axis',(-0.309016994374948,0.,0.951056516295154));
#17450=DIRECTION('',(-0.309016994374948,0.,0.951056516295154));
#17451=DIRECTION('',(0.,1.,0.));
#17452=DIRECTION('',(0.,1.,0.));
#17453=DIRECTION('center_axis',(0.,1.,0.));
#17454=DIRECTION('ref_axis',(1.,0.,0.));
#17455=DIRECTION('center_axis',(0.,1.,0.));
#17456=DIRECTION('ref_axis',(1.,0.,0.));
#17457=DIRECTION('',(0.,-1.,0.));
#17458=DIRECTION('',(0.,1.,0.));
#17459=DIRECTION('center_axis',(-0.809016994374947,0.,-0.587785252292473));
#17460=DIRECTION('ref_axis',(-0.587785252292473,0.,0.809016994374947));
#17461=DIRECTION('',(-0.587785252292473,0.,0.809016994374947));
#17462=DIRECTION('',(0.,1.,0.));
#17463=DIRECTION('',(0.,1.,0.));
#17464=DIRECTION('center_axis',(0.,1.,0.));
#17465=DIRECTION('ref_axis',(1.,0.,0.));
#17466=DIRECTION('center_axis',(0.,1.,0.));
#17467=DIRECTION('ref_axis',(1.,0.,0.));
#17468=DIRECTION('',(0.,-1.,0.));
#17469=DIRECTION('',(0.,1.,0.));
#17470=DIRECTION('center_axis',(-0.587785252292473,0.,-0.809016994374948));
#17471=DIRECTION('ref_axis',(-0.809016994374948,0.,0.587785252292473));
#17472=DIRECTION('',(-0.809016994374948,0.,0.587785252292473));
#17473=DIRECTION('',(0.,1.,0.));
#17474=DIRECTION('',(0.,1.,0.));
#17475=DIRECTION('center_axis',(0.,1.,0.));
#17476=DIRECTION('ref_axis',(1.,0.,0.));
#17477=DIRECTION('center_axis',(0.,1.,0.));
#17478=DIRECTION('ref_axis',(1.,0.,0.));
#17479=DIRECTION('',(0.,-1.,0.));
#17480=DIRECTION('',(0.,1.,0.));
#17481=DIRECTION('center_axis',(-0.309016994374947,0.,-0.951056516295154));
#17482=DIRECTION('ref_axis',(-0.951056516295154,0.,0.309016994374947));
#17483=DIRECTION('',(-0.951056516295154,0.,0.309016994374947));
#17484=DIRECTION('',(0.,1.,0.));
#17485=DIRECTION('',(0.,1.,0.));
#17486=DIRECTION('center_axis',(0.,1.,0.));
#17487=DIRECTION('ref_axis',(1.,0.,0.));
#17488=DIRECTION('center_axis',(0.,1.,0.));
#17489=DIRECTION('ref_axis',(1.,0.,0.));
#17490=DIRECTION('',(0.,-1.,0.));
#17491=DIRECTION('',(0.,1.,0.));
#17492=DIRECTION('center_axis',(6.12323399573677E-17,0.,-1.));
#17493=DIRECTION('ref_axis',(-1.,0.,-6.12323399573677E-17));
#17494=DIRECTION('',(-1.,0.,-6.12323399573677E-17));
#17495=DIRECTION('',(0.,1.,0.));
#17496=DIRECTION('',(0.,1.,0.));
#17497=DIRECTION('center_axis',(0.,1.,0.));
#17498=DIRECTION('ref_axis',(1.,0.,0.));
#17499=DIRECTION('center_axis',(0.,1.,0.));
#17500=DIRECTION('ref_axis',(1.,0.,0.));
#17501=DIRECTION('',(0.,-1.,0.));
#17502=DIRECTION('',(0.,1.,0.));
#17503=DIRECTION('center_axis',(0.309016994374948,0.,-0.951056516295154));
#17504=DIRECTION('ref_axis',(-0.951056516295154,0.,-0.309016994374948));
#17505=DIRECTION('',(-0.951056516295154,0.,-0.309016994374948));
#17506=DIRECTION('',(0.,1.,0.));
#17507=DIRECTION('',(0.,1.,0.));
#17508=DIRECTION('center_axis',(0.,1.,0.));
#17509=DIRECTION('ref_axis',(1.,0.,0.));
#17510=DIRECTION('center_axis',(0.,1.,0.));
#17511=DIRECTION('ref_axis',(1.,0.,0.));
#17512=DIRECTION('',(0.,-1.,0.));
#17513=DIRECTION('',(0.,1.,0.));
#17514=DIRECTION('center_axis',(0.587785252292473,0.,-0.809016994374947));
#17515=DIRECTION('ref_axis',(-0.809016994374947,0.,-0.587785252292473));
#17516=DIRECTION('',(-0.809016994374947,0.,-0.587785252292473));
#17517=DIRECTION('',(0.,1.,0.));
#17518=DIRECTION('',(0.,1.,0.));
#17519=DIRECTION('center_axis',(0.,1.,0.));
#17520=DIRECTION('ref_axis',(1.,0.,0.));
#17521=DIRECTION('center_axis',(0.,1.,0.));
#17522=DIRECTION('ref_axis',(1.,0.,0.));
#17523=DIRECTION('',(0.,-1.,0.));
#17524=DIRECTION('',(0.,1.,0.));
#17525=DIRECTION('center_axis',(0.809016994374947,0.,-0.587785252292473));
#17526=DIRECTION('ref_axis',(-0.587785252292473,0.,-0.809016994374947));
#17527=DIRECTION('',(-0.587785252292473,0.,-0.809016994374947));
#17528=DIRECTION('',(0.,1.,0.));
#17529=DIRECTION('',(0.,1.,0.));
#17530=DIRECTION('center_axis',(0.,1.,0.));
#17531=DIRECTION('ref_axis',(1.,0.,0.));
#17532=DIRECTION('center_axis',(0.,1.,0.));
#17533=DIRECTION('ref_axis',(1.,0.,0.));
#17534=DIRECTION('',(0.,-1.,0.));
#17535=DIRECTION('',(0.,1.,0.));
#17536=DIRECTION('center_axis',(0.951056516295154,0.,-0.309016994374947));
#17537=DIRECTION('ref_axis',(-0.309016994374947,0.,-0.951056516295154));
#17538=DIRECTION('',(-0.309016994374947,0.,-0.951056516295154));
#17539=DIRECTION('',(0.,1.,0.));
#17540=DIRECTION('',(0.,1.,0.));
#17541=DIRECTION('center_axis',(0.,1.,0.));
#17542=DIRECTION('ref_axis',(1.,0.,0.));
#17543=DIRECTION('center_axis',(0.,1.,0.));
#17544=DIRECTION('ref_axis',(1.,0.,0.));
#17545=DIRECTION('',(0.,-1.,0.));
#17546=DIRECTION('',(0.,1.,0.));
#17547=DIRECTION('center_axis',(1.,0.,0.));
#17548=DIRECTION('ref_axis',(0.,0.,-1.));
#17549=DIRECTION('',(0.,0.,-1.));
#17550=DIRECTION('',(0.,1.,0.));
#17551=DIRECTION('',(0.,1.,0.));
#17552=DIRECTION('center_axis',(0.,1.,0.));
#17553=DIRECTION('ref_axis',(1.,0.,0.));
#17554=DIRECTION('center_axis',(0.,1.,0.));
#17555=DIRECTION('ref_axis',(1.,0.,0.));
#17556=DIRECTION('center_axis',(0.,1.,0.));
#17557=DIRECTION('ref_axis',(1.,0.,0.));
#21362=CARTESIAN_POINT('',(0.,0.,0.));
#21363=CARTESIAN_POINT('Origin',(0.2,0.,0.));
#21364=CARTESIAN_POINT('',(0.2,2.2,-0.78));
#21365=CARTESIAN_POINT('',(0.2,2.2,-0.565685424949238));
#21366=CARTESIAN_POINT('',(0.2,2.2,0.));
#21367=CARTESIAN_POINT('',(0.2,-1.,-0.78));
#21368=CARTESIAN_POINT('',(0.2,0.,-0.78));
#21369=CARTESIAN_POINT('',(0.2,-1.,-0.565685424949238));
#21370=CARTESIAN_POINT('',(0.2,-1.,0.));
#21371=CARTESIAN_POINT('',(0.2,0.,-0.565685424949238));
#21372=CARTESIAN_POINT('Origin',(0.2,0.,-0.78));
#21373=CARTESIAN_POINT('',(-0.2,2.2,-0.78));
#21374=CARTESIAN_POINT('',(0.1,2.2,-0.78));
#21375=CARTESIAN_POINT('',(-0.2,-1.,-0.78));
#21376=CARTESIAN_POINT('',(-0.2,0.,-0.78));
#21377=CARTESIAN_POINT('',(0.1,-1.,-0.78));
#21378=CARTESIAN_POINT('Origin',(-0.2,0.,-0.78));
#21379=CARTESIAN_POINT('',(-0.2,2.2,-0.565685424949238));
#21380=CARTESIAN_POINT('',(-0.2,2.2,-0.39));
#21381=CARTESIAN_POINT('',(-0.2,-1.,-0.565685424949238));
#21382=CARTESIAN_POINT('',(-0.2,0.,-0.565685424949238));
#21383=CARTESIAN_POINT('',(-0.2,-1.,-0.39));
#21384=CARTESIAN_POINT('Origin',(0.,-1.,0.));
#21385=CARTESIAN_POINT('',(1.60662857109684,-1.,0.693717979106306));
#21386=CARTESIAN_POINT('',(1.5055822144029,-1.,0.892032620296856));
#21387=CARTESIAN_POINT('Origin',(0.,-1.,0.));
#21388=CARTESIAN_POINT('',(1.81978687191668,-1.,1.23627494547115));
#21389=CARTESIAN_POINT('Ctrl Pts',(1.5055822144029,-1.,0.892032620296856));
#21390=CARTESIAN_POINT('Ctrl Pts',(1.50980486806688,-1.,0.894452006964544));
#21391=CARTESIAN_POINT('Ctrl Pts',(1.51805569590094,-1.,0.899185047483511));
#21392=CARTESIAN_POINT('Ctrl Pts',(1.52984849887993,-1.,0.905967409625651));
#21393=CARTESIAN_POINT('Ctrl Pts',(1.54440491149498,-1.,0.914375919026456));
#21394=CARTESIAN_POINT('Ctrl Pts',(1.56065988578893,-1.,0.923832188944341));
#21395=CARTESIAN_POINT('Ctrl Pts',(1.57499388382243,-1.,0.932246680108685));
#21396=CARTESIAN_POINT('Ctrl Pts',(1.58744937487176,-1.,0.939646377893399));
#21397=CARTESIAN_POINT('Ctrl Pts',(1.59810042043673,-1.,0.946078063315257));
#21398=CARTESIAN_POINT('Ctrl Pts',(1.60706069896936,-1.,0.951613284356035));
#21399=CARTESIAN_POINT('Ctrl Pts',(1.61449324337085,-1.,0.956354422920671));
#21400=CARTESIAN_POINT('Ctrl Pts',(1.62061638140221,-1.,0.960438326101729));
#21401=CARTESIAN_POINT('Ctrl Pts',(1.62571930670187,-1.,0.964046107040536));
#21402=CARTESIAN_POINT('Ctrl Pts',(1.63013849959461,-1.,0.967387853230345));
#21403=CARTESIAN_POINT('Ctrl Pts',(1.63420665729798,-1.,0.970669715997509));
#21404=CARTESIAN_POINT('Ctrl Pts',(1.63820952658144,-1.,0.974066058287419));
#21405=CARTESIAN_POINT('Ctrl Pts',(1.64233990826687,-1.,0.977689794119417));
#21406=CARTESIAN_POINT('Ctrl Pts',(1.64665139190656,-1.,0.981562530939489));
#21407=CARTESIAN_POINT('Ctrl Pts',(1.65110016612638,-1.,0.985642622920821));
#21408=CARTESIAN_POINT('Ctrl Pts',(1.65559044289699,-1.,0.989855627854165));
#21409=CARTESIAN_POINT('Ctrl Pts',(1.66001553809947,-1.,0.994121836661306));
#21410=CARTESIAN_POINT('Ctrl Pts',(1.66430758030376,-1.,0.998389654952758));
#21411=CARTESIAN_POINT('Ctrl Pts',(1.66846059277303,-1.,1.00265091003727));
#21412=CARTESIAN_POINT('Ctrl Pts',(1.67250335383293,-1.,1.00692206696414));
#21413=CARTESIAN_POINT('Ctrl Pts',(1.67648246776464,-1.,1.01123236493511));
#21414=CARTESIAN_POINT('Ctrl Pts',(1.68044289894798,-1.,1.01561026162773));
#21415=CARTESIAN_POINT('Ctrl Pts',(1.68440578021706,-1.,1.02006795074201));
#21416=CARTESIAN_POINT('Ctrl Pts',(1.68836910178447,-1.,1.02460180535255));
#21417=CARTESIAN_POINT('Ctrl Pts',(1.69231840863458,-1.,1.02919977579147));
#21418=CARTESIAN_POINT('Ctrl Pts',(1.69623414782771,-1.,1.03384646003588));
#21419=CARTESIAN_POINT('Ctrl Pts',(1.70010052930962,-1.,1.03852922490789));
#21420=CARTESIAN_POINT('Ctrl Pts',(1.70391338707982,-1.,1.04324363334554));
#21421=CARTESIAN_POINT('Ctrl Pts',(1.70767646263649,-1.,1.04799085404995));
#21422=CARTESIAN_POINT('Ctrl Pts',(1.71139783543989,-1.,1.05277517202855));
#21423=CARTESIAN_POINT('Ctrl Pts',(1.7150865442702,-1.,1.05760163192479));
#21424=CARTESIAN_POINT('Ctrl Pts',(1.71874858456904,-1.,1.06247324680647));
#21425=CARTESIAN_POINT('Ctrl Pts',(1.72238500928453,-1.,1.06738966975462));
#21426=CARTESIAN_POINT('Ctrl Pts',(1.72599406198488,-1.,1.07234866990252));
#21427=CARTESIAN_POINT('Ctrl Pts',(1.72957248977424,-1.,1.0773470373727));
#21428=CARTESIAN_POINT('Ctrl Pts',(1.73311705663407,-1.,1.08238162784749));
#21429=CARTESIAN_POINT('Ctrl Pts',(1.73662628326091,-1.,1.08745056285427));
#21430=CARTESIAN_POINT('Ctrl Pts',(1.74010053962247,-1.,1.09255329056493));
#21431=CARTESIAN_POINT('Ctrl Pts',(1.74354119236208,-1.,1.09768999241226));
#21432=CARTESIAN_POINT('Ctrl Pts',(1.74695004214923,-1.,1.10286118991143));
#21433=CARTESIAN_POINT('Ctrl Pts',(1.7503286607592,-1.,1.10806728183007));
#21434=CARTESIAN_POINT('Ctrl Pts',(1.7536777209463,-1.,1.11330807582551));
#21435=CARTESIAN_POINT('Ctrl Pts',(1.75699720772105,-1.,1.11858293216763));
#21436=CARTESIAN_POINT('Ctrl Pts',(1.76028671825096,-1.,1.12389096855086));
#21437=CARTESIAN_POINT('Ctrl Pts',(1.7635457196617,-1.,1.12923123555075));
#21438=CARTESIAN_POINT('Ctrl Pts',(1.76677384551862,-1.,1.1346029180462));
#21439=CARTESIAN_POINT('Ctrl Pts',(1.76997111386769,-1.,1.14000548336975));
#21440=CARTESIAN_POINT('Ctrl Pts',(1.77313777896194,-1.,1.1454385822692));
#21441=CARTESIAN_POINT('Ctrl Pts',(1.7762742255701,-1.,1.15090197841515));
#21442=CARTESIAN_POINT('Ctrl Pts',(1.77938085564275,-1.,1.15639547194698));
#21443=CARTESIAN_POINT('Ctrl Pts',(1.78245795881009,-1.,1.16191881298499));
#21444=CARTESIAN_POINT('Ctrl Pts',(1.78550566040443,-1.,1.16747166312303));
#21445=CARTESIAN_POINT('Ctrl Pts',(1.78852398877616,-1.,1.17305363177328));
#21446=CARTESIAN_POINT('Ctrl Pts',(1.79151291552689,-1.,1.17866429440809));
#21447=CARTESIAN_POINT('Ctrl Pts',(1.79447240321515,-1.,1.18430321697432));
#21448=CARTESIAN_POINT('Ctrl Pts',(1.79740245923478,-1.,1.18996997934445));
#21449=CARTESIAN_POINT('Ctrl Pts',(1.80030314369879,-1.,1.19566418930242));
#21450=CARTESIAN_POINT('Ctrl Pts',(1.80317454838603,-1.,1.20138548938974));
#21451=CARTESIAN_POINT('Ctrl Pts',(1.80601678480707,-1.,1.20713356605475));
#21452=CARTESIAN_POINT('Ctrl Pts',(1.80882996917129,-1.,1.21290815708314));
#21453=CARTESIAN_POINT('Ctrl Pts',(1.81161420806656,-1.,1.21870906103557));
#21454=CARTESIAN_POINT('Ctrl Pts',(1.81436959210434,-1.,1.2245361330495));
#21455=CARTESIAN_POINT('Ctrl Pts',(1.8165508718364,-1.,1.2292186489137));
#21456=CARTESIAN_POINT('Ctrl Pts',(1.81817389921279,-1.,1.2327422452705));
#21457=CARTESIAN_POINT('Ctrl Pts',(1.81925017193666,-1.,1.23509651170476));
#21458=CARTESIAN_POINT('Ctrl Pts',(1.81978687191668,-1.,1.23627494547115));
#21459=CARTESIAN_POINT('',(1.73811241238545,-1.,1.34869019493419));
#21460=CARTESIAN_POINT('',(1.81978687191668,-1.,1.23627494547115));
#21461=CARTESIAN_POINT('',(1.31362392696032,-1.,1.15624053661742));
#21462=CARTESIAN_POINT('Ctrl Pts',(1.73811241238545,-1.,1.34869019493419));
#21463=CARTESIAN_POINT('Ctrl Pts',(1.73682580585691,-1.,1.34854391898045));
#21464=CARTESIAN_POINT('Ctrl Pts',(1.73425417885907,-1.,1.34824783112887));
#21465=CARTESIAN_POINT('Ctrl Pts',(1.7304014965394,-1.,1.34779309152035));
#21466=CARTESIAN_POINT('Ctrl Pts',(1.72527410680674,-1.,1.34716554819527));
#21467=CARTESIAN_POINT('Ctrl Pts',(1.7188807715049,-1.,1.34634568653227));
#21468=CARTESIAN_POINT('Ctrl Pts',(1.71250340686822,-1.,1.34549029589416));
#21469=CARTESIAN_POINT('Ctrl Pts',(1.70614212266738,-1.,1.34459924533831));
#21470=CARTESIAN_POINT('Ctrl Pts',(1.69979707754427,-1.,1.34367237124483));
#21471=CARTESIAN_POINT('Ctrl Pts',(1.6934684849687,-1.,1.34270948206319));
#21472=CARTESIAN_POINT('Ctrl Pts',(1.68715660868764,-1.,1.341710374848));
#21473=CARTESIAN_POINT('Ctrl Pts',(1.68086176030362,-1.,1.34067485185203));
#21474=CARTESIAN_POINT('Ctrl Pts',(1.67458429426086,-1.,1.3396027347034));
#21475=CARTESIAN_POINT('Ctrl Pts',(1.66832460783989,-1.,1.33849388654388));
#21476=CARTESIAN_POINT('Ctrl Pts',(1.66208312541983,-1.,1.33734820885262));
#21477=CARTESIAN_POINT('Ctrl Pts',(1.65586025952593,-1.,1.33616559745172));
#21478=CARTESIAN_POINT('Ctrl Pts',(1.6496563728683,-1.,1.33494590467993));
#21479=CARTESIAN_POINT('Ctrl Pts',(1.6434717485603,-1.,1.33368890676572));
#21480=CARTESIAN_POINT('Ctrl Pts',(1.63730653475089,-1.,1.33239425103724));
#21481=CARTESIAN_POINT('Ctrl Pts',(1.63116079730923,-1.,1.33106149345645));
#21482=CARTESIAN_POINT('Ctrl Pts',(1.62503464209797,-1.,1.3296901950568));
#21483=CARTESIAN_POINT('Ctrl Pts',(1.61892832270724,-1.,1.32828000610449));
#21484=CARTESIAN_POINT('Ctrl Pts',(1.6128423401575,-1.,1.32683074483356));
#21485=CARTESIAN_POINT('Ctrl Pts',(1.60677758290954,-1.,1.32534250785782));
#21486=CARTESIAN_POINT('Ctrl Pts',(1.60073511858687,-1.,1.32381550858256));
#21487=CARTESIAN_POINT('Ctrl Pts',(1.59471591079403,-1.,1.32224985747682));
#21488=CARTESIAN_POINT('Ctrl Pts',(1.58872057258245,-1.,1.32064537110892));
#21489=CARTESIAN_POINT('Ctrl Pts',(1.58274907898834,-1.,1.31900135021432));
#21490=CARTESIAN_POINT('Ctrl Pts',(1.5768005650559,-1.,1.31731642317187));
#21491=CARTESIAN_POINT('Ctrl Pts',(1.57087397835723,-1.,1.31558903860016));
#21492=CARTESIAN_POINT('Ctrl Pts',(1.56496872402353,-1.,1.31381795281002));
#21493=CARTESIAN_POINT('Ctrl Pts',(1.55908521254821,-1.,1.31200264341696));
#21494=CARTESIAN_POINT('Ctrl Pts',(1.55322568759481,-1.,1.31014393684222));
#21495=CARTESIAN_POINT('Ctrl Pts',(1.54739413957185,-1.,1.30824393907473));
#21496=CARTESIAN_POINT('Ctrl Pts',(1.54159462645432,-1.,1.30630475189556));
#21497=CARTESIAN_POINT('Ctrl Pts',(1.53582981268977,-1.,1.30432735639489));
#21498=CARTESIAN_POINT('Ctrl Pts',(1.53009970283891,-1.,1.30231064395568));
#21499=CARTESIAN_POINT('Ctrl Pts',(1.52439957861062,-1.,1.30024984366328));
#21500=CARTESIAN_POINT('Ctrl Pts',(1.51872184912724,-1.,1.29813791800747));
#21501=CARTESIAN_POINT('Ctrl Pts',(1.51305994241402,-1.,1.29596850710509));
#21502=CARTESIAN_POINT('Ctrl Pts',(1.50741159078365,-1.,1.29373841372842));
#21503=CARTESIAN_POINT('Ctrl Pts',(1.50178230149776,-1.,1.29145022885181));
#21504=CARTESIAN_POINT('Ctrl Pts',(1.49618896881754,-1.,1.28911506584254));
#21505=CARTESIAN_POINT('Ctrl Pts',(1.4906522831278,-1.,1.2867467611644));
#21506=CARTESIAN_POINT('Ctrl Pts',(1.4851881711891,-1.,1.28435533880201));
#21507=CARTESIAN_POINT('Ctrl Pts',(1.47980070347095,-1.,1.28194158939517));
#21508=CARTESIAN_POINT('Ctrl Pts',(1.4744717526707,-1.,1.2794891824849));
#21509=CARTESIAN_POINT('Ctrl Pts',(1.46916035917133,-1.,1.2769641483109));
#21510=CARTESIAN_POINT('Ctrl Pts',(1.46382431332476,-1.,1.27433119897822));
#21511=CARTESIAN_POINT('Ctrl Pts',(1.45843906294697,-1.,1.27156805265289));
#21512=CARTESIAN_POINT('Ctrl Pts',(1.45301422764247,-1.,1.2686778680489));
#21513=CARTESIAN_POINT('Ctrl Pts',(1.44761985001662,-1.,1.26570925118868));
#21514=CARTESIAN_POINT('Ctrl Pts',(1.44236470511303,-1.,1.26273903323859));
#21515=CARTESIAN_POINT('Ctrl Pts',(1.43734919180847,-1.,1.25983531012005));
#21516=CARTESIAN_POINT('Ctrl Pts',(1.43262645609691,-1.,1.25702687965755));
#21517=CARTESIAN_POINT('Ctrl Pts',(1.42815938799387,-1.,1.25426945222639));
#21518=CARTESIAN_POINT('Ctrl Pts',(1.42378102115575,-1.,1.2514145557001));
#21519=CARTESIAN_POINT('Ctrl Pts',(1.41923722596025,-1.,1.24824430986571));
#21520=CARTESIAN_POINT('Ctrl Pts',(1.41422913175179,-1.,1.24450600513056));
#21521=CARTESIAN_POINT('Ctrl Pts',(1.40845295531283,-1.,1.23994455029534));
#21522=CARTESIAN_POINT('Ctrl Pts',(1.40164708206106,-1.,1.23434087290423));
#21523=CARTESIAN_POINT('Ctrl Pts',(1.39361389568796,-1.,1.22752961899387));
#21524=CARTESIAN_POINT('Ctrl Pts',(1.38420564527715,-1.,1.21938737280852));
#21525=CARTESIAN_POINT('Ctrl Pts',(1.37331915607905,-1.,1.20982812925645));
#21526=CARTESIAN_POINT('Ctrl Pts',(1.36088705043885,-1.,1.1987959077932));
#21527=CARTESIAN_POINT('Ctrl Pts',(1.34687054001093,-1.,1.18625865667441));
#21528=CARTESIAN_POINT('Ctrl Pts',(1.33437539347008,-1.,1.17501305789857));
#21529=CARTESIAN_POINT('Ctrl Pts',(1.32428080721772,-1.,1.16589330093588));
#21530=CARTESIAN_POINT('Ctrl Pts',(1.31722977216397,-1.,1.15950888730809));
#21531=CARTESIAN_POINT('Ctrl Pts',(1.31362392696032,-1.,1.15624053661742));
#21532=CARTESIAN_POINT('',(1.15624053661742,-1.,1.31362392696033));
#21533=CARTESIAN_POINT('Origin',(0.,-1.,0.));
#21534=CARTESIAN_POINT('',(1.34869019493419,-1.,1.73811241238545));
#21535=CARTESIAN_POINT('Ctrl Pts',(1.15624053661742,-1.,1.31362392696033));
#21536=CARTESIAN_POINT('Ctrl Pts',(1.15950888730433,-1.,1.3172297721596));
#21537=CARTESIAN_POINT('Ctrl Pts',(1.16589330092532,-1.,1.32428080720544));
#21538=CARTESIAN_POINT('Ctrl Pts',(1.17501305787994,-1.,1.33437539344842));
#21539=CARTESIAN_POINT('Ctrl Pts',(1.18625865664915,-1.,1.34687053998157));
#21540=CARTESIAN_POINT('Ctrl Pts',(1.1987959077656,-1.,1.36088705040677));
#21541=CARTESIAN_POINT('Ctrl Pts',(1.20982812923113,-1.,1.37331915604962));
#21542=CARTESIAN_POINT('Ctrl Pts',(1.21938737278853,-1.,1.38420564525391));
#21543=CARTESIAN_POINT('Ctrl Pts',(1.22752961898063,-1.,1.39361389567257));
#21544=CARTESIAN_POINT('Ctrl Pts',(1.23434087289768,-1.,1.40164708205345));
#21545=CARTESIAN_POINT('Ctrl Pts',(1.23994455029421,-1.,1.40845295531151));
#21546=CARTESIAN_POINT('Ctrl Pts',(1.24450600513278,-1.,1.41422913175437));
#21547=CARTESIAN_POINT('Ctrl Pts',(1.24824430986911,-1.,1.41923722596421));
#21548=CARTESIAN_POINT('Ctrl Pts',(1.25141455570299,-1.,1.42378102115911));
#21549=CARTESIAN_POINT('Ctrl Pts',(1.25426945222783,-1.,1.42815938799555));
#21550=CARTESIAN_POINT('Ctrl Pts',(1.25702687965744,-1.,1.43262645609679));
#21551=CARTESIAN_POINT('Ctrl Pts',(1.25983531011894,-1.,1.43734919180719));
#21552=CARTESIAN_POINT('Ctrl Pts',(1.26273903323723,-1.,1.44236470511145));
#21553=CARTESIAN_POINT('Ctrl Pts',(1.26570925118767,-1.,1.44761985001544));
#21554=CARTESIAN_POINT('Ctrl Pts',(1.26867786804854,-1.,1.45301422764205));
#21555=CARTESIAN_POINT('Ctrl Pts',(1.27156805265312,-1.,1.45843906294725));
#21556=CARTESIAN_POINT('Ctrl Pts',(1.27433119897877,-1.,1.4638243133254));
#21557=CARTESIAN_POINT('Ctrl Pts',(1.27696414831144,-1.,1.46916035917197));
#21558=CARTESIAN_POINT('Ctrl Pts',(1.27948918248524,-1.,1.4744717526711));
#21559=CARTESIAN_POINT('Ctrl Pts',(1.28194158939522,-1.,1.47980070347102));
#21560=CARTESIAN_POINT('Ctrl Pts',(1.28435533880184,-1.,1.48518817118891));
#21561=CARTESIAN_POINT('Ctrl Pts',(1.28674676116415,-1.,1.4906522831275));
#21562=CARTESIAN_POINT('Ctrl Pts',(1.28911506584232,-1.,1.49618896881729));
#21563=CARTESIAN_POINT('Ctrl Pts',(1.29145022885171,-1.,1.50178230149764));
#21564=CARTESIAN_POINT('Ctrl Pts',(1.29373841372843,-1.,1.50741159078367));
#21565=CARTESIAN_POINT('Ctrl Pts',(1.29596850710518,-1.,1.51305994241412));
#21566=CARTESIAN_POINT('Ctrl Pts',(1.29813791800757,-1.,1.51872184912735));
#21567=CARTESIAN_POINT('Ctrl Pts',(1.30024984366334,-1.,1.5243995786107));
#21568=CARTESIAN_POINT('Ctrl Pts',(1.3023106439557,-1.,1.53009970283893));
#21569=CARTESIAN_POINT('Ctrl Pts',(1.30432735639487,-1.,1.53582981268976));
#21570=CARTESIAN_POINT('Ctrl Pts',(1.30630475189553,-1.,1.54159462645428));
#21571=CARTESIAN_POINT('Ctrl Pts',(1.30824393907471,-1.,1.54739413957183));
#21572=CARTESIAN_POINT('Ctrl Pts',(1.31014393684221,-1.,1.55322568759481));
#21573=CARTESIAN_POINT('Ctrl Pts',(1.31200264341696,-1.,1.55908521254822));
#21574=CARTESIAN_POINT('Ctrl Pts',(1.31381795281002,-1.,1.56496872402352));
#21575=CARTESIAN_POINT('Ctrl Pts',(1.31558903860015,-1.,1.57087397835721));
#21576=CARTESIAN_POINT('Ctrl Pts',(1.31731642317183,-1.,1.57680056505585));
#21577=CARTESIAN_POINT('Ctrl Pts',(1.31900135021428,-1.,1.58274907898829));
#21578=CARTESIAN_POINT('Ctrl Pts',(1.32064537110891,-1.,1.58872057258244));
#21579=CARTESIAN_POINT('Ctrl Pts',(1.32224985747686,-1.,1.59471591079408));
#21580=CARTESIAN_POINT('Ctrl Pts',(1.32381550858266,-1.,1.600735118587));
#21581=CARTESIAN_POINT('Ctrl Pts',(1.32534250785794,-1.,1.6067775829097));
#21582=CARTESIAN_POINT('Ctrl Pts',(1.32683074483365,-1.,1.61284234015762));
#21583=CARTESIAN_POINT('Ctrl Pts',(1.32828000610448,-1.,1.61892832270723));
#21584=CARTESIAN_POINT('Ctrl Pts',(1.32969019505665,-1.,1.62503464209777));
#21585=CARTESIAN_POINT('Ctrl Pts',(1.33106149345618,-1.,1.63116079730887));
#21586=CARTESIAN_POINT('Ctrl Pts',(1.33239425103694,-1.,1.6373065347505));
#21587=CARTESIAN_POINT('Ctrl Pts',(1.33368890676554,-1.,1.64347174856007));
#21588=CARTESIAN_POINT('Ctrl Pts',(1.33494590468003,-1.,1.64965637286843));
#21589=CARTESIAN_POINT('Ctrl Pts',(1.33616559745217,-1.,1.65586025952651));
#21590=CARTESIAN_POINT('Ctrl Pts',(1.33734820885331,-1.,1.66208312542073));
#21591=CARTESIAN_POINT('Ctrl Pts',(1.33849388654458,-1.,1.66832460784078));
#21592=CARTESIAN_POINT('Ctrl Pts',(1.33960273470372,-1.,1.67458429426126));
#21593=CARTESIAN_POINT('Ctrl Pts',(1.3406748518516,-1.,1.68086176030308));
#21594=CARTESIAN_POINT('Ctrl Pts',(1.34171037484673,-1.,1.68715660868602));
#21595=CARTESIAN_POINT('Ctrl Pts',(1.34270948206139,-1.,1.6934684849664));
#21596=CARTESIAN_POINT('Ctrl Pts',(1.34367237124322,-1.,1.69979707754221));
#21597=CARTESIAN_POINT('Ctrl Pts',(1.34459924533783,-1.,1.70614212266676));
#21598=CARTESIAN_POINT('Ctrl Pts',(1.34549029589563,-1.,1.71250340687011));
#21599=CARTESIAN_POINT('Ctrl Pts',(1.34634568653586,-1.,1.7188807715095));
#21600=CARTESIAN_POINT('Ctrl Pts',(1.34716554820013,-1.,1.72527410681298));
#21601=CARTESIAN_POINT('Ctrl Pts',(1.3477930915247,-1.,1.73040149654497));
#21602=CARTESIAN_POINT('Ctrl Pts',(1.34824783113158,-1.,1.73425417886255));
#21603=CARTESIAN_POINT('Ctrl Pts',(1.34854391898145,-1.,1.73682580585819));
#21604=CARTESIAN_POINT('Ctrl Pts',(1.34869019493419,-1.,1.73811241238545));
#21605=CARTESIAN_POINT('',(1.23627494547115,-1.,1.81978687191668));
#21606=CARTESIAN_POINT('',(1.34869019493419,-1.,1.73811241238545));
#21607=CARTESIAN_POINT('',(0.892032620296855,-1.,1.5055822144029));
#21608=CARTESIAN_POINT('Ctrl Pts',(1.23627494547115,-1.,1.81978687191668));
#21609=CARTESIAN_POINT('Ctrl Pts',(1.23509651170384,-1.,1.81925017193531));
#21610=CARTESIAN_POINT('Ctrl Pts',(1.23274224526804,-1.,1.81817389920914));
#21611=CARTESIAN_POINT('Ctrl Pts',(1.22921864890975,-1.,1.81655087183054));
#21612=CARTESIAN_POINT('Ctrl Pts',(1.22453613304507,-1.,1.81436959209778));
#21613=CARTESIAN_POINT('Ctrl Pts',(1.2187090610323,-1.,1.81161420806172));
#21614=CARTESIAN_POINT('Ctrl Pts',(1.2129081570818,-1.,1.80882996916931));
#21615=CARTESIAN_POINT('Ctrl Pts',(1.20713356605519,-1.,1.80601678480772));
#21616=CARTESIAN_POINT('Ctrl Pts',(1.2013854893912,-1.,1.8031745483882));
#21617=CARTESIAN_POINT('Ctrl Pts',(1.19566418930405,-1.,1.80030314370121));
#21618=CARTESIAN_POINT('Ctrl Pts',(1.1899699793456,-1.,1.79740245923649));
#21619=CARTESIAN_POINT('Ctrl Pts',(1.18430321697471,-1.,1.79447240321572));
#21620=CARTESIAN_POINT('Ctrl Pts',(1.17866429440781,-1.,1.79151291552646));
#21621=CARTESIAN_POINT('Ctrl Pts',(1.17305363177265,-1.,1.78852398877523));
#21622=CARTESIAN_POINT('Ctrl Pts',(1.16747166312239,-1.,1.78550566040349));
#21623=CARTESIAN_POINT('Ctrl Pts',(1.16191881298458,-1.,1.78245795880949));
#21624=CARTESIAN_POINT('Ctrl Pts',(1.15639547194689,-1.,1.77938085564261));
#21625=CARTESIAN_POINT('Ctrl Pts',(1.15090197841531,-1.,1.77627422557034));
#21626=CARTESIAN_POINT('Ctrl Pts',(1.14543858226948,-1.,1.77313777896234));
#21627=CARTESIAN_POINT('Ctrl Pts',(1.14000548337,-1.,1.76997111386806));
#21628=CARTESIAN_POINT('Ctrl Pts',(1.13460291804634,-1.,1.76677384551883));
#21629=CARTESIAN_POINT('Ctrl Pts',(1.12923123555076,-1.,1.76354571966171));
#21630=CARTESIAN_POINT('Ctrl Pts',(1.12389096855078,-1.,1.76028671825084));
#21631=CARTESIAN_POINT('Ctrl Pts',(1.11858293216752,-1.,1.75699720772089));
#21632=CARTESIAN_POINT('Ctrl Pts',(1.11330807582542,-1.,1.75367772094617));
#21633=CARTESIAN_POINT('Ctrl Pts',(1.10806728183003,-1.,1.75032866075914));
#21634=CARTESIAN_POINT('Ctrl Pts',(1.10286118991144,-1.,1.74695004214924));
#21635=CARTESIAN_POINT('Ctrl Pts',(1.09768999241229,-1.,1.74354119236212));
#21636=CARTESIAN_POINT('Ctrl Pts',(1.09255329056496,-1.,1.74010053962252));
#21637=CARTESIAN_POINT('Ctrl Pts',(1.08745056285429,-1.,1.73662628326093));
#21638=CARTESIAN_POINT('Ctrl Pts',(1.08238162784749,-1.,1.73311705663407));
#21639=CARTESIAN_POINT('Ctrl Pts',(1.0773470373727,-1.,1.72957248977424));
#21640=CARTESIAN_POINT('Ctrl Pts',(1.07234866990252,-1.,1.72599406198489));
#21641=CARTESIAN_POINT('Ctrl Pts',(1.06738966975463,-1.,1.72238500928456));
#21642=CARTESIAN_POINT('Ctrl Pts',(1.06247324680649,-1.,1.71874858456908));
#21643=CARTESIAN_POINT('Ctrl Pts',(1.05760163192481,-1.,1.71508654427022));
#21644=CARTESIAN_POINT('Ctrl Pts',(1.05277517202853,-1.,1.71139783543986));
#21645=CARTESIAN_POINT('Ctrl Pts',(1.0479908540499,-1.,1.70767646263641));
#21646=CARTESIAN_POINT('Ctrl Pts',(1.04324363334546,-1.,1.70391338707969));
#21647=CARTESIAN_POINT('Ctrl Pts',(1.03852922490782,-1.,1.70010052930951));
#21648=CARTESIAN_POINT('Ctrl Pts',(1.03384646003587,-1.,1.69623414782769));
#21649=CARTESIAN_POINT('Ctrl Pts',(1.02919977579155,-1.,1.69231840863471));
#21650=CARTESIAN_POINT('Ctrl Pts',(1.02460180535272,-1.,1.68836910178475));
#21651=CARTESIAN_POINT('Ctrl Pts',(1.02006795074222,-1.,1.68440578021739));
#21652=CARTESIAN_POINT('Ctrl Pts',(1.01561026162786,-1.,1.6804428989482));
#21653=CARTESIAN_POINT('Ctrl Pts',(1.01123236493507,-1.,1.67648246776457));
#21654=CARTESIAN_POINT('Ctrl Pts',(1.00692206696387,-1.,1.67250335383248));
#21655=CARTESIAN_POINT('Ctrl Pts',(1.00265091003682,-1.,1.66846059277231));
#21656=CARTESIAN_POINT('Ctrl Pts',(0.998389654952317,-1.,1.66430758030304));
#21657=CARTESIAN_POINT('Ctrl Pts',(0.994121836661115,-1.,1.66001553809916));
#21658=CARTESIAN_POINT('Ctrl Pts',(0.98985562785445,-1.,1.65559044289746));
#21659=CARTESIAN_POINT('Ctrl Pts',(0.985642622921626,-1.,1.6511001661277));
#21660=CARTESIAN_POINT('Ctrl Pts',(0.981562530940574,-1.,1.64665139190834));
#21661=CARTESIAN_POINT('Ctrl Pts',(0.977689794120296,-1.,1.64233990826831));
#21662=CARTESIAN_POINT('Ctrl Pts',(0.974066058287501,-1.,1.63820952658157));
#21663=CARTESIAN_POINT('Ctrl Pts',(0.970669715996356,-1.,1.63420665729609));
#21664=CARTESIAN_POINT('Ctrl Pts',(0.967387853228041,-1.,1.63013849959083));
#21665=CARTESIAN_POINT('Ctrl Pts',(0.964046107037821,-1.,1.6257193066974));
#21666=CARTESIAN_POINT('Ctrl Pts',(0.960438326099958,-1.,1.62061638139929));
#21667=CARTESIAN_POINT('Ctrl Pts',(0.956354422921572,-1.,1.61449324337233));
#21668=CARTESIAN_POINT('Ctrl Pts',(0.951613284361247,-1.,1.60706069897794));
#21669=CARTESIAN_POINT('Ctrl Pts',(0.946078063325795,-1.,1.59810042045408));
#21670=CARTESIAN_POINT('Ctrl Pts',(0.939646377909319,-1.,1.58744937489796));
#21671=CARTESIAN_POINT('Ctrl Pts',(0.932246680128848,-1.,1.57499388385561));
#21672=CARTESIAN_POINT('Ctrl Pts',(0.923832188966322,-1.,1.56065988582509));
#21673=CARTESIAN_POINT('Ctrl Pts',(0.914375919046579,-1.,1.54440491152808));
#21674=CARTESIAN_POINT('Ctrl Pts',(0.905967409640498,-1.,1.52984849890434));
#21675=CARTESIAN_POINT('Ctrl Pts',(0.89918504749193,-1.,1.51805569591479));
#21676=CARTESIAN_POINT('Ctrl Pts',(0.894452006967538,-1.,1.50980486807181));
#21677=CARTESIAN_POINT('Ctrl Pts',(0.892032620296855,-1.,1.5055822144029));
#21678=CARTESIAN_POINT('',(0.693717979106305,-1.,1.60662857109684));
#21679=CARTESIAN_POINT('Origin',(0.,-1.,0.));
#21680=CARTESIAN_POINT('',(0.7455743247944,-1.,2.0698113262342));
#21681=CARTESIAN_POINT('Ctrl Pts',(0.693717979106305,-1.,1.60662857109684));
#21682=CARTESIAN_POINT('Ctrl Pts',(0.69571209787897,-1.,1.61106790957619));
#21683=CARTESIAN_POINT('Ctrl Pts',(0.699605146398836,-1.,1.61974673471117));
#21684=CARTESIAN_POINT('Ctrl Pts',(0.705159151977294,-1.,1.6321654166204));
#21685=CARTESIAN_POINT('Ctrl Pts',(0.711993139340447,-1.,1.64752408828442));
#21686=CARTESIAN_POINT('Ctrl Pts',(0.719585433787949,-1.,1.66472880551777));
#21687=CARTESIAN_POINT('Ctrl Pts',(0.726235967982445,-1.,1.67996158451922));
#21688=CARTESIAN_POINT('Ctrl Pts',(0.731963238685357,-1.,1.69326921972915));
#21689=CARTESIAN_POINT('Ctrl Pts',(0.736799665716932,-1.,1.70473309004249));
#21690=CARTESIAN_POINT('Ctrl Pts',(0.74079516202821,-1.,1.71447789751001));
#21691=CARTESIAN_POINT('Ctrl Pts',(0.744021445433093,-1.,1.72268229916769));
#21692=CARTESIAN_POINT('Ctrl Pts',(0.746574710097752,-1.,1.72958533647714));
#21693=CARTESIAN_POINT('Ctrl Pts',(0.74858246295687,-1.,1.7355035168033));
#21694=CARTESIAN_POINT('Ctrl Pts',(0.750193435981249,-1.,1.74080458267114));
#21695=CARTESIAN_POINT('Ctrl Pts',(0.751555614164482,-1.,1.74585086852502));
#21696=CARTESIAN_POINT('Ctrl Pts',(0.752797683531314,-1.,1.75095139468794));
#21697=CARTESIAN_POINT('Ctrl Pts',(0.754009254027828,-1.,1.75631083600019));
#21698=CARTESIAN_POINT('Ctrl Pts',(0.755220979974461,-1.,1.76197817240128));
#21699=CARTESIAN_POINT('Ctrl Pts',(0.75642189602781,-1.,1.76789396002998));
#21700=CARTESIAN_POINT('Ctrl Pts',(0.757578264077028,-1.,1.77394167108292));
#21701=CARTESIAN_POINT('Ctrl Pts',(0.758650626677518,-1.,1.77999411220945));
#21702=CARTESIAN_POINT('Ctrl Pts',(0.759614401110189,-1.,1.78596964884604));
#21703=CARTESIAN_POINT('Ctrl Pts',(0.760469555880749,-1.,1.7918581561088));
#21704=CARTESIAN_POINT('Ctrl Pts',(0.761229695230558,-1.,1.79768986997783));
#21705=CARTESIAN_POINT('Ctrl Pts',(0.761915336443547,-1.,1.80351583877342));
#21706=CARTESIAN_POINT('Ctrl Pts',(0.762546129463938,-1.,1.80938551463965));
#21707=CARTESIAN_POINT('Ctrl Pts',(0.763132003836634,-1.,1.8153211840553));
#21708=CARTESIAN_POINT('Ctrl Pts',(0.763673465462726,-1.,1.82131873145266));
#21709=CARTESIAN_POINT('Ctrl Pts',(0.764165902605995,-1.,1.82735991200065));
#21710=CARTESIAN_POINT('Ctrl Pts',(0.764602549687853,-1.,1.83342077227142));
#21711=CARTESIAN_POINT('Ctrl Pts',(0.764978057881737,-1.,1.83948181064835));
#21712=CARTESIAN_POINT('Ctrl Pts',(0.765291664862029,-1.,1.84553698875924));
#21713=CARTESIAN_POINT('Ctrl Pts',(0.765545710619062,-1.,1.85158945130063));
#21714=CARTESIAN_POINT('Ctrl Pts',(0.765744212909318,-1.,1.85764741390394));
#21715=CARTESIAN_POINT('Ctrl Pts',(0.765891519092547,-1.,1.86372027063312));
#21716=CARTESIAN_POINT('Ctrl Pts',(0.765990708546091,-1.,1.86981398314341));
#21717=CARTESIAN_POINT('Ctrl Pts',(0.766042837036744,-1.,1.87592888967883));
#21718=CARTESIAN_POINT('Ctrl Pts',(0.766047794851864,-1.,1.88206215302561));
#21719=CARTESIAN_POINT('Ctrl Pts',(0.766004837062091,-1.,1.88820926433409));
#21720=CARTESIAN_POINT('Ctrl Pts',(0.765913193856978,-1.,1.89436577771388));
#21721=CARTESIAN_POINT('Ctrl Pts',(0.765772772593386,-1.,1.90052930393596));
#21722=CARTESIAN_POINT('Ctrl Pts',(0.765584196937919,-1.,1.90669961402356));
#21723=CARTESIAN_POINT('Ctrl Pts',(0.765348465884722,-1.,1.91287765805169));
#21724=CARTESIAN_POINT('Ctrl Pts',(0.765066729667088,-1.,1.91906491634196));
#21725=CARTESIAN_POINT('Ctrl Pts',(0.764740025488211,-1.,1.92526263537048));
#21726=CARTESIAN_POINT('Ctrl Pts',(0.76436901067394,-1.,1.93147105496382));
#21727=CARTESIAN_POINT('Ctrl Pts',(0.763954049121458,-1.,1.93768964875886));
#21728=CARTESIAN_POINT('Ctrl Pts',(0.763495333538629,-1.,1.9439174661764));
#21729=CARTESIAN_POINT('Ctrl Pts',(0.762992990878769,-1.,1.95015342590024));
#21730=CARTESIAN_POINT('Ctrl Pts',(0.762447203806178,-1.,1.95639665309869));
#21731=CARTESIAN_POINT('Ctrl Pts',(0.761858300014423,-1.,1.96264672744186));
#21732=CARTESIAN_POINT('Ctrl Pts',(0.76122669048382,-1.,1.96890351582499));
#21733=CARTESIAN_POINT('Ctrl Pts',(0.760552825409757,-1.,1.97516705321494));
#21734=CARTESIAN_POINT('Ctrl Pts',(0.75983714745219,-1.,1.98143741418172));
#21735=CARTESIAN_POINT('Ctrl Pts',(0.759080037802488,-1.,1.98771456680874));
#21736=CARTESIAN_POINT('Ctrl Pts',(0.758281796766761,-1.,1.99399831098817));
#21737=CARTESIAN_POINT('Ctrl Pts',(0.757442676862724,-1.,2.00028834739178));
#21738=CARTESIAN_POINT('Ctrl Pts',(0.75656290464667,-1.,2.0065843158773));
#21739=CARTESIAN_POINT('Ctrl Pts',(0.755642704957865,-1.,2.01288584328084));
#21740=CARTESIAN_POINT('Ctrl Pts',(0.754682330722816,-1.,2.01919259405809));
#21741=CARTESIAN_POINT('Ctrl Pts',(0.753682061112768,-1.,2.02550428623313));
#21742=CARTESIAN_POINT('Ctrl Pts',(0.75264218048721,-1.,2.03182068456221));
#21743=CARTESIAN_POINT('Ctrl Pts',(0.751562963361115,-1.,2.03814160092099));
#21744=CARTESIAN_POINT('Ctrl Pts',(0.750444657875575,-1.,2.04446689147979));
#21745=CARTESIAN_POINT('Ctrl Pts',(0.749287468665046,-1.,2.05079645592154));
#21746=CARTESIAN_POINT('Ctrl Pts',(0.748091554183802,-1.,2.05713023031007));
#21747=CARTESIAN_POINT('Ctrl Pts',(0.747103932787919,-1.,2.06220058927826));
#21748=CARTESIAN_POINT('Ctrl Pts',(0.7463458715442,-1.,2.06600523016815));
#21749=CARTESIAN_POINT('Ctrl Pts',(0.745832791378367,-1.,2.06854248895728));
#21750=CARTESIAN_POINT('Ctrl Pts',(0.7455743247944,-1.,2.0698113262342));
#21751=CARTESIAN_POINT('',(0.61342227326009,-1.,2.11275013067528));
#21752=CARTESIAN_POINT('',(0.7455743247944,-1.,2.0698113262342));
#21753=CARTESIAN_POINT('',(0.383122945602004,-1.,1.7075470150345));
#21754=CARTESIAN_POINT('Ctrl Pts',(0.61342227326009,-1.,2.11275013067528));
#21755=CARTESIAN_POINT('Ctrl Pts',(0.6124673655618,-1.,2.11187554259986));
#21756=CARTESIAN_POINT('Ctrl Pts',(0.610560911689898,-1.,2.11012443807238));
#21757=CARTESIAN_POINT('Ctrl Pts',(0.607711315454876,-1.,2.1074919961518));
#21758=CARTESIAN_POINT('Ctrl Pts',(0.60393203073603,-1.,2.10397049886949));
#21759=CARTESIAN_POINT('Ctrl Pts',(0.599241616420533,-1.,2.0995493086477));
#21760=CARTESIAN_POINT('Ctrl Pts',(0.594585006052162,-1.,2.0951087622027));
#21761=CARTESIAN_POINT('Ctrl Pts',(0.589962365403406,-1.,2.09064881812129));
#21762=CARTESIAN_POINT('Ctrl Pts',(0.585373918991617,-1.,2.08616943727951));
#21763=CARTESIAN_POINT('Ctrl Pts',(0.580819952108063,-1.,2.08167059018418));
#21764=CARTESIAN_POINT('Ctrl Pts',(0.576300797416844,-1.,2.07715226767559));
#21765=CARTESIAN_POINT('Ctrl Pts',(0.571816823242602,-1.,2.07261449292824));
#21766=CARTESIAN_POINT('Ctrl Pts',(0.567368421181087,-1.,2.06805732997334));
#21767=CARTESIAN_POINT('Ctrl Pts',(0.562955993082261,-1.,2.06348090160589));
#21768=CARTESIAN_POINT('Ctrl Pts',(0.558579940185151,-1.,2.05888537756462));
#21769=CARTESIAN_POINT('Ctrl Pts',(0.554240657463906,-1.,2.05427091604413));
#21770=CARTESIAN_POINT('Ctrl Pts',(0.549938525150295,-1.,2.04963761077958));
#21771=CARTESIAN_POINT('Ctrl Pts',(0.54567390381743,-1.,2.04498544714588));
#21772=CARTESIAN_POINT('Ctrl Pts',(0.541447120615659,-1.,2.04031422690527));
#21773=CARTESIAN_POINT('Ctrl Pts',(0.537258489833262,-1.,2.03562362954037));
#21774=CARTESIAN_POINT('Ctrl Pts',(0.533108355132976,-1.,2.03091336214426));
#21775=CARTESIAN_POINT('Ctrl Pts',(0.528997127241914,-1.,2.0261832908329));
#21776=CARTESIAN_POINT('Ctrl Pts',(0.524925318333476,-1.,2.02143356304698));
#21777=CARTESIAN_POINT('Ctrl Pts',(0.52089359039937,-1.,2.01666477917286));
#21778=CARTESIAN_POINT('Ctrl Pts',(0.516902681728687,-1.,2.01187773939242));
#21779=CARTESIAN_POINT('Ctrl Pts',(0.512953306961792,-1.,2.00707309946949));
#21780=CARTESIAN_POINT('Ctrl Pts',(0.509046069886157,-1.,2.00225107134734));
#21781=CARTESIAN_POINT('Ctrl Pts',(0.505181361323026,-1.,1.99741107463572));
#21782=CARTESIAN_POINT('Ctrl Pts',(0.501359287727146,-1.,1.99255149126155));
#21783=CARTESIAN_POINT('Ctrl Pts',(0.497579909545574,-1.,1.98767044752932));
#21784=CARTESIAN_POINT('Ctrl Pts',(0.493843476541494,-1.,1.98276658761821));
#21785=CARTESIAN_POINT('Ctrl Pts',(0.490150627860952,-1.,1.97783973019229));
#21786=CARTESIAN_POINT('Ctrl Pts',(0.486502692907658,-1.,1.97289186263272));
#21787=CARTESIAN_POINT('Ctrl Pts',(0.48290166212069,-1.,1.96792703422362));
#21788=CARTESIAN_POINT('Ctrl Pts',(0.479349583074855,-1.,1.96294933055943));
#21789=CARTESIAN_POINT('Ctrl Pts',(0.475848034683176,-1.,1.95796111148177));
#21790=CARTESIAN_POINT('Ctrl Pts',(0.472397672264072,-1.,1.95296148278133));
#21791=CARTESIAN_POINT('Ctrl Pts',(0.468997482913135,-1.,1.94794381136514));
#21792=CARTESIAN_POINT('Ctrl Pts',(0.46564546202603,-1.,1.9428979419619));
#21793=CARTESIAN_POINT('Ctrl Pts',(0.462340031009056,-1.,1.93781486640821));
#21794=CARTESIAN_POINT('Ctrl Pts',(0.459081234547926,-1.,1.93269066517934));
#21795=CARTESIAN_POINT('Ctrl Pts',(0.45587200517437,-1.,1.92753067150476));
#21796=CARTESIAN_POINT('Ctrl Pts',(0.452719478359432,-1.,1.92235380648502));
#21797=CARTESIAN_POINT('Ctrl Pts',(0.449632260106662,-1.,1.91718342555755));
#21798=CARTESIAN_POINT('Ctrl Pts',(0.446617343485711,-1.,1.9120369998112));
#21799=CARTESIAN_POINT('Ctrl Pts',(0.44367755684915,-1.,1.90691756144898));
#21800=CARTESIAN_POINT('Ctrl Pts',(0.440807833704038,-1.,1.90180124389086));
#21801=CARTESIAN_POINT('Ctrl Pts',(0.437995003948244,-1.,1.89663648956466));
#21802=CARTESIAN_POINT('Ctrl Pts',(0.435225660963383,-1.,1.89136993975504));
#21803=CARTESIAN_POINT('Ctrl Pts',(0.432493038548748,-1.,1.88596913666793));
#21804=CARTESIAN_POINT('Ctrl Pts',(0.429803062482344,-1.,1.88044229001832));
#21805=CARTESIAN_POINT('Ctrl Pts',(0.427183828519102,-1.,1.87486989291484));
#21806=CARTESIAN_POINT('Ctrl Pts',(0.424678177291358,-1.,1.86937803944323));
#21807=CARTESIAN_POINT('Ctrl Pts',(0.422327307418275,-1.,1.86408083334028));
#21808=CARTESIAN_POINT('Ctrl Pts',(0.420157287975619,-1.,1.85903281096686));
#21809=CARTESIAN_POINT('Ctrl Pts',(0.418164129143534,-1.,1.85417632856234));
#21810=CARTESIAN_POINT('Ctrl Pts',(0.416300022038864,-1.,1.84929312929882));
#21811=CARTESIAN_POINT('Ctrl Pts',(0.41448743825434,-1.,1.8440575707371));
#21812=CARTESIAN_POINT('Ctrl Pts',(0.412633125322161,-1.,1.83808953475839));
#21813=CARTESIAN_POINT('Ctrl Pts',(0.410641256301674,-1.,1.83100408895216));
#21814=CARTESIAN_POINT('Ctrl Pts',(0.408428948108533,-1.,1.8224702267854));
#21815=CARTESIAN_POINT('Ctrl Pts',(0.405933518411838,-1.,1.81223801813988));
#21816=CARTESIAN_POINT('Ctrl Pts',(0.403107976170441,-1.,1.80012077176221));
#21817=CARTESIAN_POINT('Ctrl Pts',(0.39991940378308,-1.,1.78598826347533));
#21818=CARTESIAN_POINT('Ctrl Pts',(0.39634619612042,-1.,1.7697556004756));
#21819=CARTESIAN_POINT('Ctrl Pts',(0.392375812294307,-1.,1.75137405313962));
#21820=CARTESIAN_POINT('Ctrl Pts',(0.388877023509191,-1.,1.7349317097561));
#21821=CARTESIAN_POINT('Ctrl Pts',(0.38607079032701,-1.,1.72162022246158));
#21822=CARTESIAN_POINT('Ctrl Pts',(0.384119047315541,-1.,1.71231062891958));
#21823=CARTESIAN_POINT('Ctrl Pts',(0.383122945602004,-1.,1.7075470150345));
#21824=CARTESIAN_POINT('',(0.163289472382896,-1.,1.74236521665491));
#21825=CARTESIAN_POINT('Origin',(0.,-1.,0.));
#21826=CARTESIAN_POINT('',(0.0694764450219578,-1.,2.19890268624765));
#21827=CARTESIAN_POINT('Ctrl Pts',(0.163289472382896,-1.,1.74236521665491));
#21828=CARTESIAN_POINT('Ctrl Pts',(0.163814161002002,-1.,1.7472034950333));
#21829=CARTESIAN_POINT('Ctrl Pts',(0.164834765707158,-1.,1.75666056638427));
#21830=CARTESIAN_POINT('Ctrl Pts',(0.1662793551464,-1.,1.77018771684844));
#21831=CARTESIAN_POINT('Ctrl Pts',(0.168032772805197,-1.,1.7869064998507));
#21832=CARTESIAN_POINT('Ctrl Pts',(0.169936923904608,-1.,1.80561530629706));
#21833=CARTESIAN_POINT('Ctrl Pts',(0.171554770204119,-1.,1.82215766811545));
#21834=CARTESIAN_POINT('Ctrl Pts',(0.1728894428919,-1.,1.83658380527692));
#21835=CARTESIAN_POINT('Ctrl Pts',(0.173946627587731,-1.,1.8489811319852));
#21836=CARTESIAN_POINT('Ctrl Pts',(0.17473525927603,-1.,1.85948367088837));
#21837=CARTESIAN_POINT('Ctrl Pts',(0.175268337590757,-1.,1.86828349694799));
#21838=CARTESIAN_POINT('Ctrl Pts',(0.175563480746485,-1.,1.87563767773588));
#21839=CARTESIAN_POINT('Ctrl Pts',(0.175644148889698,-1.,1.88188663145367));
#21840=CARTESIAN_POINT('Ctrl Pts',(0.175538155840648,-1.,1.88742606273259));
#21841=CARTESIAN_POINT('Ctrl Pts',(0.175274276190844,-1.,1.892646301985));
#21842=CARTESIAN_POINT('Ctrl Pts',(0.174879405091263,-1.,1.89788101117132));
#21843=CARTESIAN_POINT('Ctrl Pts',(0.174375518661085,-1.,1.90335253862834));
#21844=CARTESIAN_POINT('Ctrl Pts',(0.173776635257816,-1.,1.90911693975267));
#21845=CARTESIAN_POINT('Ctrl Pts',(0.173090695383496,-1.,1.91511429159527));
#21846=CARTESIAN_POINT('Ctrl Pts',(0.172321621259513,-1.,1.9212233439798));
#21847=CARTESIAN_POINT('Ctrl Pts',(0.171471191532988,-1.,1.92731093582036));
#21848=CARTESIAN_POINT('Ctrl Pts',(0.170541253116201,-1.,1.93329183155539));
#21849=CARTESIAN_POINT('Ctrl Pts',(0.16953490481749,-1.,1.93915639211581));
#21850=CARTESIAN_POINT('Ctrl Pts',(0.168455741607556,-1.,1.94493757756931));
#21851=CARTESIAN_POINT('Ctrl Pts',(0.167307501784475,-1.,1.95069027794294));
#21852=CARTESIAN_POINT('Ctrl Pts',(0.166093592002812,-1.,1.9564675971873));
#21853=CARTESIAN_POINT('Ctrl Pts',(0.164816568920269,-1.,1.96229379940136));
#21854=CARTESIAN_POINT('Ctrl Pts',(0.163478185457734,-1.,1.96816512677967));
#21855=CARTESIAN_POINT('Ctrl Pts',(0.162079693556288,-1.,1.97406280235188));
#21856=CARTESIAN_POINT('Ctrl Pts',(0.160622060784611,-1.,1.97996195437559));
#21857=CARTESIAN_POINT('Ctrl Pts',(0.159106226437299,-1.,1.98584238283292));
#21858=CARTESIAN_POINT('Ctrl Pts',(0.157533331459227,-1.,1.99169810931908));
#21859=CARTESIAN_POINT('Ctrl Pts',(0.155904629548783,-1.,1.99753284771497));
#21860=CARTESIAN_POINT('Ctrl Pts',(0.154221403049722,-1.,2.00335565310543));
#21861=CARTESIAN_POINT('Ctrl Pts',(0.152484883621449,-1.,2.00917680318424));
#21862=CARTESIAN_POINT('Ctrl Pts',(0.150696157673078,-1.,2.01500291940238));
#21863=CARTESIAN_POINT('Ctrl Pts',(0.148856124775337,-1.,2.02083464969894));
#21864=CARTESIAN_POINT('Ctrl Pts',(0.146965557332583,-1.,2.02666926182017));
#21865=CARTESIAN_POINT('Ctrl Pts',(0.145025140186057,-1.,2.03250223739942));
#21866=CARTESIAN_POINT('Ctrl Pts',(0.143035515058208,-1.,2.03832911025912));
#21867=CARTESIAN_POINT('Ctrl Pts',(0.140997332152546,-1.,2.04414757947916));
#21868=CARTESIAN_POINT('Ctrl Pts',(0.138911255368966,-1.,2.04995762001328));
#21869=CARTESIAN_POINT('Ctrl Pts',(0.136777941218043,-1.,2.05576044414264));
#21870=CARTESIAN_POINT('Ctrl Pts',(0.134598026192106,-1.,2.06155781517842));
#21871=CARTESIAN_POINT('Ctrl Pts',(0.13237211154771,-1.,2.06735123910326));
#21872=CARTESIAN_POINT('Ctrl Pts',(0.130100748328403,-1.,2.07314114713063));
#21873=CARTESIAN_POINT('Ctrl Pts',(0.12778444527612,-1.,2.07892715110987));
#21874=CARTESIAN_POINT('Ctrl Pts',(0.125423679412061,-1.,2.08470840653643));
#21875=CARTESIAN_POINT('Ctrl Pts',(0.123018905621083,-1.,2.09048392424825));
#21876=CARTESIAN_POINT('Ctrl Pts',(0.120570567965122,-1.,2.0962529286773));
#21877=CARTESIAN_POINT('Ctrl Pts',(0.118079107988355,-1.,2.102015121329));
#21878=CARTESIAN_POINT('Ctrl Pts',(0.115544957687926,-1.,2.10777050261309));
#21879=CARTESIAN_POINT('Ctrl Pts',(0.112968534419737,-1.,2.11351924490306));
#21880=CARTESIAN_POINT('Ctrl Pts',(0.110350236135025,-1.,2.11926155590865));
#21881=CARTESIAN_POINT('Ctrl Pts',(0.10769043523109,-1.,2.12499752307));
#21882=CARTESIAN_POINT('Ctrl Pts',(0.104989479152739,-1.,2.13072704887293));
#21883=CARTESIAN_POINT('Ctrl Pts',(0.1022477005561,-1.,2.13644992667165));
#21884=CARTESIAN_POINT('Ctrl Pts',(0.0994654261990913,-1.,2.14216588396025));
#21885=CARTESIAN_POINT('Ctrl Pts',(0.0966429852305456,-1.,2.14787463531795));
#21886=CARTESIAN_POINT('Ctrl Pts',(0.0937807218867641,-1.,2.1535759397817));
#21887=CARTESIAN_POINT('Ctrl Pts',(0.0908789888107263,-1.,2.15926961544516));
#21888=CARTESIAN_POINT('Ctrl Pts',(0.087938129138692,-1.,2.16495552645014));
#21889=CARTESIAN_POINT('Ctrl Pts',(0.084958462083537,-1.,2.17063357870952));
#21890=CARTESIAN_POINT('Ctrl Pts',(0.0819402680872763,-1.,2.176303712113));
#21891=CARTESIAN_POINT('Ctrl Pts',(0.078883772768524,-1.,2.18196589448887));
#21892=CARTESIAN_POINT('Ctrl Pts',(0.0757891465836145,-1.,2.1876201139953));
#21893=CARTESIAN_POINT('Ctrl Pts',(0.0732830357306722,-1.,2.19213712013662));
#21894=CARTESIAN_POINT('Ctrl Pts',(0.0713863779526151,-1.,2.19552129484002));
#21895=CARTESIAN_POINT('Ctrl Pts',(0.0701143536325487,-1.,2.19777582085423));
#21896=CARTESIAN_POINT('Ctrl Pts',(0.0694764450219578,-1.,2.19890268624765));
#21897=CARTESIAN_POINT('',(-0.0694764450219586,-1.,2.19890268624765));
#21898=CARTESIAN_POINT('',(0.0694764450219578,-1.,2.19890268624765));
#21899=CARTESIAN_POINT('',(-0.163289472382896,-1.,1.74236521665491));
#21900=CARTESIAN_POINT('Ctrl Pts',(-0.0694764450219586,-1.,2.19890268624765));
#21901=CARTESIAN_POINT('Ctrl Pts',(-0.0701143536324929,-1.,2.19777582085261));
#21902=CARTESIAN_POINT('Ctrl Pts',(-0.071386377952463,-1.,2.19552129483562));
#21903=CARTESIAN_POINT('Ctrl Pts',(-0.0732830357304279,-1.,2.19213712012956));
#21904=CARTESIAN_POINT('Ctrl Pts',(-0.0757891465833414,-1.,2.1876201139874));
#21905=CARTESIAN_POINT('Ctrl Pts',(-0.078883772768323,-1.,2.18196589448304));
#21906=CARTESIAN_POINT('Ctrl Pts',(-0.0819402680871942,-1.,2.1763037121106));
#21907=CARTESIAN_POINT('Ctrl Pts',(-0.0849584620835646,-1.,2.17063357871031));
#21908=CARTESIAN_POINT('Ctrl Pts',(-0.0879381291387825,-1.,2.16495552645275));
#21909=CARTESIAN_POINT('Ctrl Pts',(-0.0908789888108269,-1.,2.15926961544808));
#21910=CARTESIAN_POINT('Ctrl Pts',(-0.0937807218868348,-1.,2.15357593978377));
#21911=CARTESIAN_POINT('Ctrl Pts',(-0.0966429852305691,-1.,2.14787463531864));
#21912=CARTESIAN_POINT('Ctrl Pts',(-0.0994654261990745,-1.,2.14216588395974));
#21913=CARTESIAN_POINT('Ctrl Pts',(-0.102247700556064,-1.,2.13644992667052));
#21914=CARTESIAN_POINT('Ctrl Pts',(-0.104989479152703,-1.,2.1307270488718));
#21915=CARTESIAN_POINT('Ctrl Pts',(-0.107690435231068,-1.,2.12499752306927));
#21916=CARTESIAN_POINT('Ctrl Pts',(-0.11035023613502,-1.,2.11926155590849));
#21917=CARTESIAN_POINT('Ctrl Pts',(-0.112968534419746,-1.,2.11351924490335));
#21918=CARTESIAN_POINT('Ctrl Pts',(-0.115544957687941,-1.,2.10777050261359));
#21919=CARTESIAN_POINT('Ctrl Pts',(-0.118079107988368,-1.,2.10201512132945));
#21920=CARTESIAN_POINT('Ctrl Pts',(-0.120570567965129,-1.,2.09625292867756));
#21921=CARTESIAN_POINT('Ctrl Pts',(-0.123018905621083,-1.,2.09048392424826));
#21922=CARTESIAN_POINT('Ctrl Pts',(-0.125423679412058,-1.,2.08470840653628));
#21923=CARTESIAN_POINT('Ctrl Pts',(-0.127784445276116,-1.,2.07892715110967));
#21924=CARTESIAN_POINT('Ctrl Pts',(-0.130100748328401,-1.,2.07314114713047));
#21925=CARTESIAN_POINT('Ctrl Pts',(-0.13237211154771,-1.,2.06735123910319));
#21926=CARTESIAN_POINT('Ctrl Pts',(-0.134598026192107,-1.,2.06155781517844));
#21927=CARTESIAN_POINT('Ctrl Pts',(-0.136777941218044,-1.,2.0557604441427));
#21928=CARTESIAN_POINT('Ctrl Pts',(-0.138911255368966,-1.,2.04995762001333));
#21929=CARTESIAN_POINT('Ctrl Pts',(-0.140997332152546,-1.,2.04414757947919));
#21930=CARTESIAN_POINT('Ctrl Pts',(-0.143035515058208,-1.,2.03832911025913));
#21931=CARTESIAN_POINT('Ctrl Pts',(-0.145025140186058,-1.,2.03250223739941));
#21932=CARTESIAN_POINT('Ctrl Pts',(-0.146965557332586,-1.,2.02666926182017));
#21933=CARTESIAN_POINT('Ctrl Pts',(-0.148856124775343,-1.,2.02083464969897));
#21934=CARTESIAN_POINT('Ctrl Pts',(-0.150696157673084,-1.,2.01500291940243));
#21935=CARTESIAN_POINT('Ctrl Pts',(-0.152484883621452,-1.,2.00917680318426));
#21936=CARTESIAN_POINT('Ctrl Pts',(-0.154221403049719,-1.,2.00335565310539));
#21937=CARTESIAN_POINT('Ctrl Pts',(-0.155904629548775,-1.,1.99753284771487));
#21938=CARTESIAN_POINT('Ctrl Pts',(-0.157533331459215,-1.,1.99169810931893));
#21939=CARTESIAN_POINT('Ctrl Pts',(-0.159106226437289,-1.,1.98584238283279));
#21940=CARTESIAN_POINT('Ctrl Pts',(-0.16062206078461,-1.,1.97996195437557));
#21941=CARTESIAN_POINT('Ctrl Pts',(-0.162079693556302,-1.,1.97406280235204));
#21942=CARTESIAN_POINT('Ctrl Pts',(-0.16347818545776,-1.,1.96816512678));
#21943=CARTESIAN_POINT('Ctrl Pts',(-0.1648165689203,-1.,1.96229379940174));
#21944=CARTESIAN_POINT('Ctrl Pts',(-0.166093592002833,-1.,1.95646759718755));
#21945=CARTESIAN_POINT('Ctrl Pts',(-0.167307501784469,-1.,1.95069027794286));
#21946=CARTESIAN_POINT('Ctrl Pts',(-0.168455741607516,-1.,1.94493757756879));
#21947=CARTESIAN_POINT('Ctrl Pts',(-0.169534904817425,-1.,1.93915639211497));
#21948=CARTESIAN_POINT('Ctrl Pts',(-0.170541253116136,-1.,1.93329183155455));
#21949=CARTESIAN_POINT('Ctrl Pts',(-0.17147119153296,-1.,1.92731093582));
#21950=CARTESIAN_POINT('Ctrl Pts',(-0.172321621259557,-1.,1.92122334398034));
#21951=CARTESIAN_POINT('Ctrl Pts',(-0.173090695383619,-1.,1.91511429159681));
#21952=CARTESIAN_POINT('Ctrl Pts',(-0.173776635257984,-1.,1.90911693975475));
#21953=CARTESIAN_POINT('Ctrl Pts',(-0.174375518661222,-1.,1.90335253863003));
#21954=CARTESIAN_POINT('Ctrl Pts',(-0.174879405091277,-1.,1.89788101117148));
#21955=CARTESIAN_POINT('Ctrl Pts',(-0.175274276190664,-1.,1.89264630198279));
#21956=CARTESIAN_POINT('Ctrl Pts',(-0.175538155840286,-1.,1.88742606272818));
#21957=CARTESIAN_POINT('Ctrl Pts',(-0.175644148889271,-1.,1.88188663144846));
#21958=CARTESIAN_POINT('Ctrl Pts',(-0.175563480746206,-1.,1.87563767773249));
#21959=CARTESIAN_POINT('Ctrl Pts',(-0.175268337590901,-1.,1.86828349694972));
#21960=CARTESIAN_POINT('Ctrl Pts',(-0.174735259276856,-1.,1.85948367089838));
#21961=CARTESIAN_POINT('Ctrl Pts',(-0.173946627589401,-1.,1.84898113200543));
#21962=CARTESIAN_POINT('Ctrl Pts',(-0.17288944289442,-1.,1.83658380530747));
#21963=CARTESIAN_POINT('Ctrl Pts',(-0.171554770207306,-1.,1.82215766815414));
#21964=CARTESIAN_POINT('Ctrl Pts',(-0.169936923908078,-1.,1.80561530633924));
#21965=CARTESIAN_POINT('Ctrl Pts',(-0.16803277280837,-1.,1.78690649988931));
#21966=CARTESIAN_POINT('Ctrl Pts',(-0.166279355148738,-1.,1.77018771687692));
#21967=CARTESIAN_POINT('Ctrl Pts',(-0.164834765708484,-1.,1.75666056640041));
#21968=CARTESIAN_POINT('Ctrl Pts',(-0.163814161002474,-1.,1.74720349503904));
#21969=CARTESIAN_POINT('Ctrl Pts',(-0.163289472382896,-1.,1.74236521665491));
#21970=CARTESIAN_POINT('',(-0.383122945602004,-1.,1.7075470150345));
#21971=CARTESIAN_POINT('Origin',(0.,-1.,0.));
#21972=CARTESIAN_POINT('',(-0.61342227326009,-1.,2.11275013067528));
#21973=CARTESIAN_POINT('Ctrl Pts',(-0.383122945602004,-1.,1.7075470150345));
#21974=CARTESIAN_POINT('Ctrl Pts',(-0.384119047314215,-1.,1.71231062891398));
#21975=CARTESIAN_POINT('Ctrl Pts',(-0.386070790323281,-1.,1.72162022244582));
#21976=CARTESIAN_POINT('Ctrl Pts',(-0.388877023502615,-1.,1.73493170972829));
#21977=CARTESIAN_POINT('Ctrl Pts',(-0.392375812285395,-1.,1.75137405310193));
#21978=CARTESIAN_POINT('Ctrl Pts',(-0.396346196110688,-1.,1.76975560043442));
#21979=CARTESIAN_POINT('Ctrl Pts',(-0.399919403774155,-1.,1.78598826343754));
#21980=CARTESIAN_POINT('Ctrl Pts',(-0.403107976163396,-1.,1.80012077173238));
#21981=CARTESIAN_POINT('Ctrl Pts',(-0.405933518407175,-1.,1.81223801812013));
#21982=CARTESIAN_POINT('Ctrl Pts',(-0.408428948106227,-1.,1.82247022677562));
#21983=CARTESIAN_POINT('Ctrl Pts',(-0.410641256301276,-1.,1.83100408895047));
#21984=CARTESIAN_POINT('Ctrl Pts',(-0.412633125322945,-1.,1.8380895347617));
#21985=CARTESIAN_POINT('Ctrl Pts',(-0.414487438255542,-1.,1.84405757074218));
#21986=CARTESIAN_POINT('Ctrl Pts',(-0.416300022039885,-1.,1.84929312930314));
#21987=CARTESIAN_POINT('Ctrl Pts',(-0.418164129144045,-1.,1.8541763285645));
#21988=CARTESIAN_POINT('Ctrl Pts',(-0.420157287975583,-1.,1.8590328109667));
#21989=CARTESIAN_POINT('Ctrl Pts',(-0.422327307417885,-1.,1.86408083333863));
#21990=CARTESIAN_POINT('Ctrl Pts',(-0.424678177290876,-1.,1.8693780394412));
#21991=CARTESIAN_POINT('Ctrl Pts',(-0.427183828518743,-1.,1.87486989291333));
#21992=CARTESIAN_POINT('Ctrl Pts',(-0.429803062482217,-1.,1.88044229001778));
#21993=CARTESIAN_POINT('Ctrl Pts',(-0.432493038548833,-1.,1.88596913666828));
#21994=CARTESIAN_POINT('Ctrl Pts',(-0.43522566096358,-1.,1.89136993975585));
#21995=CARTESIAN_POINT('Ctrl Pts',(-0.437995003948443,-1.,1.89663648956549));
#21996=CARTESIAN_POINT('Ctrl Pts',(-0.440807833704161,-1.,1.90180124389137));
#21997=CARTESIAN_POINT('Ctrl Pts',(-0.44367755684917,-1.,1.90691756144906));
#21998=CARTESIAN_POINT('Ctrl Pts',(-0.446617343485651,-1.,1.91203699981095));
#21999=CARTESIAN_POINT('Ctrl Pts',(-0.449632260106572,-1.,1.91718342555717));
#22000=CARTESIAN_POINT('Ctrl Pts',(-0.452719478359356,-1.,1.9223538064847));
#22001=CARTESIAN_POINT('Ctrl Pts',(-0.455872005174335,-1.,1.92753067150461));
#22002=CARTESIAN_POINT('Ctrl Pts',(-0.459081234547931,-1.,1.93269066517936));
#22003=CARTESIAN_POINT('Ctrl Pts',(-0.462340031009087,-1.,1.93781486640834));
#22004=CARTESIAN_POINT('Ctrl Pts',(-0.465645462026065,-1.,1.94289794196205));
#22005=CARTESIAN_POINT('Ctrl Pts',(-0.468997482913158,-1.,1.94794381136524));
#22006=CARTESIAN_POINT('Ctrl Pts',(-0.47239767226408,-1.,1.95296148278136));
#22007=CARTESIAN_POINT('Ctrl Pts',(-0.475848034683172,-1.,1.95796111148175));
#22008=CARTESIAN_POINT('Ctrl Pts',(-0.479349583074846,-1.,1.96294933055938));
#22009=CARTESIAN_POINT('Ctrl Pts',(-0.482901662120687,-1.,1.96792703422358));
#22010=CARTESIAN_POINT('Ctrl Pts',(-0.486502692907661,-1.,1.97289186263272));
#22011=CARTESIAN_POINT('Ctrl Pts',(-0.490150627860955,-1.,1.97783973019229));
#22012=CARTESIAN_POINT('Ctrl Pts',(-0.493843476541492,-1.,1.9827665876182));
#22013=CARTESIAN_POINT('Ctrl Pts',(-0.497579909545564,-1.,1.98767044752929));
#22014=CARTESIAN_POINT('Ctrl Pts',(-0.501359287727129,-1.,1.9925514912615));
#22015=CARTESIAN_POINT('Ctrl Pts',(-0.505181361323011,-1.,1.99741107463567));
#22016=CARTESIAN_POINT('Ctrl Pts',(-0.509046069886152,-1.,2.00225107134733));
#22017=CARTESIAN_POINT('Ctrl Pts',(-0.512953306961814,-1.,2.00707309946955));
#22018=CARTESIAN_POINT('Ctrl Pts',(-0.516902681728733,-1.,2.01187773939257));
#22019=CARTESIAN_POINT('Ctrl Pts',(-0.520893590399428,-1.,2.01666477917305));
#22020=CARTESIAN_POINT('Ctrl Pts',(-0.524925318333518,-1.,2.02143356304712));
#22021=CARTESIAN_POINT('Ctrl Pts',(-0.528997127241911,-1.,2.02618329083289));
#22022=CARTESIAN_POINT('Ctrl Pts',(-0.533108355132905,-1.,2.03091336214401));
#22023=CARTESIAN_POINT('Ctrl Pts',(-0.537258489833134,-1.,2.03562362953993));
#22024=CARTESIAN_POINT('Ctrl Pts',(-0.54144712061552,-1.,2.0403142269048));
#22025=CARTESIAN_POINT('Ctrl Pts',(-0.545673903817348,-1.,2.0449854471456));
#22026=CARTESIAN_POINT('Ctrl Pts',(-0.549938525150342,-1.,2.04963761077974));
#22027=CARTESIAN_POINT('Ctrl Pts',(-0.55424065746411,-1.,2.05427091604482));
#22028=CARTESIAN_POINT('Ctrl Pts',(-0.558579940185467,-1.,2.05888537756571));
#22029=CARTESIAN_POINT('Ctrl Pts',(-0.562955993082574,-1.,2.06348090160697));
#22030=CARTESIAN_POINT('Ctrl Pts',(-0.567368421181229,-1.,2.06805732997383));
#22031=CARTESIAN_POINT('Ctrl Pts',(-0.571816823242411,-1.,2.07261449292757));
#22032=CARTESIAN_POINT('Ctrl Pts',(-0.576300797416275,-1.,2.07715226767361));
#22033=CARTESIAN_POINT('Ctrl Pts',(-0.580819952107257,-1.,2.08167059018138));
#22034=CARTESIAN_POINT('Ctrl Pts',(-0.585373918990895,-1.,2.086169437277));
#22035=CARTESIAN_POINT('Ctrl Pts',(-0.589962365403189,-1.,2.09064881812053));
#22036=CARTESIAN_POINT('Ctrl Pts',(-0.594585006052824,-1.,2.09510876220501));
#22037=CARTESIAN_POINT('Ctrl Pts',(-0.599241616422144,-1.,2.09954930865331));
#22038=CARTESIAN_POINT('Ctrl Pts',(-0.603932030738212,-1.,2.10397049887709));
#22039=CARTESIAN_POINT('Ctrl Pts',(-0.607711315456826,-1.,2.10749199615859));
#22040=CARTESIAN_POINT('Ctrl Pts',(-0.610560911691113,-1.,2.11012443807661));
#22041=CARTESIAN_POINT('Ctrl Pts',(-0.61246736556225,-1.,2.11187554260142));
#22042=CARTESIAN_POINT('Ctrl Pts',(-0.61342227326009,-1.,2.11275013067528));
#22043=CARTESIAN_POINT('',(-0.745574324794401,-1.,2.0698113262342));
#22044=CARTESIAN_POINT('',(-0.61342227326009,-1.,2.11275013067528));
#22045=CARTESIAN_POINT('',(-0.693717979106306,-1.,1.60662857109684));
#22046=CARTESIAN_POINT('Ctrl Pts',(-0.745574324794401,-1.,2.0698113262342));
#22047=CARTESIAN_POINT('Ctrl Pts',(-0.74583279137781,-1.,2.06854248895575));
#22048=CARTESIAN_POINT('Ctrl Pts',(-0.746345871542696,-1.,2.06600523016401));
#22049=CARTESIAN_POINT('Ctrl Pts',(-0.747103932785504,-1.,2.06220058927162));
#22050=CARTESIAN_POINT('Ctrl Pts',(-0.748091554181101,-1.,2.05713023030263));
#22051=CARTESIAN_POINT('Ctrl Pts',(-0.749287468663053,-1.,2.05079645591606));
#22052=CARTESIAN_POINT('Ctrl Pts',(-0.750444657874758,-1.,2.04446689147754));
#22053=CARTESIAN_POINT('Ctrl Pts',(-0.751562963361384,-1.,2.03814160092173));
#22054=CARTESIAN_POINT('Ctrl Pts',(-0.752642180488104,-1.,2.03182068456467));
#22055=CARTESIAN_POINT('Ctrl Pts',(-0.753682061113766,-1.,2.02550428623587));
#22056=CARTESIAN_POINT('Ctrl Pts',(-0.75468233072352,-1.,2.01919259406003));
#22057=CARTESIAN_POINT('Ctrl Pts',(-0.7556427049581,-1.,2.01288584328149));
#22058=CARTESIAN_POINT('Ctrl Pts',(-0.756562904646496,-1.,2.00658431587682));
#22059=CARTESIAN_POINT('Ctrl Pts',(-0.757442676862341,-1.,2.00028834739072));
#22060=CARTESIAN_POINT('Ctrl Pts',(-0.758281796766377,-1.,1.9939983109871));
#22061=CARTESIAN_POINT('Ctrl Pts',(-0.759080037802243,-1.,1.98771456680806));
#22062=CARTESIAN_POINT('Ctrl Pts',(-0.759837147452135,-1.,1.98143741418156));
#22063=CARTESIAN_POINT('Ctrl Pts',(-0.760552825409855,-1.,1.97516705321521));
#22064=CARTESIAN_POINT('Ctrl Pts',(-0.761226690483986,-1.,1.96890351582545));
#22065=CARTESIAN_POINT('Ctrl Pts',(-0.761858300014575,-1.,1.96264672744229));
#22066=CARTESIAN_POINT('Ctrl Pts',(-0.762447203806263,-1.,1.95639665309893));
#22067=CARTESIAN_POINT('Ctrl Pts',(-0.762992990878774,-1.,1.95015342590025));
#22068=CARTESIAN_POINT('Ctrl Pts',(-0.76349533353858,-1.,1.94391746617626));
#22069=CARTESIAN_POINT('Ctrl Pts',(-0.763954049121393,-1.,1.93768964875867));
#22070=CARTESIAN_POINT('Ctrl Pts',(-0.764369010673889,-1.,1.93147105496367));
#22071=CARTESIAN_POINT('Ctrl Pts',(-0.764740025488189,-1.,1.92526263537041));
#22072=CARTESIAN_POINT('Ctrl Pts',(-0.765066729667095,-1.,1.91906491634197));
#22073=CARTESIAN_POINT('Ctrl Pts',(-0.765348465884739,-1.,1.91287765805174));
#22074=CARTESIAN_POINT('Ctrl Pts',(-0.765584196937936,-1.,1.90669961402362));
#22075=CARTESIAN_POINT('Ctrl Pts',(-0.765772772593395,-1.,1.90052930393599));
#22076=CARTESIAN_POINT('Ctrl Pts',(-0.765913193856979,-1.,1.89436577771389));
#22077=CARTESIAN_POINT('Ctrl Pts',(-0.76600483706209,-1.,1.88820926433409));
#22078=CARTESIAN_POINT('Ctrl Pts',(-0.766047794851869,-1.,1.88206215302561));
#22079=CARTESIAN_POINT('Ctrl Pts',(-0.766042837036759,-1.,1.87592888967886));
#22080=CARTESIAN_POINT('Ctrl Pts',(-0.765990708546111,-1.,1.86981398314345));
#22081=CARTESIAN_POINT('Ctrl Pts',(-0.765891519092557,-1.,1.86372027063314));
#22082=CARTESIAN_POINT('Ctrl Pts',(-0.765744212909305,-1.,1.85764741390391));
#22083=CARTESIAN_POINT('Ctrl Pts',(-0.765545710619023,-1.,1.85158945130054));
#22084=CARTESIAN_POINT('Ctrl Pts',(-0.765291664861971,-1.,1.8455369887591));
#22085=CARTESIAN_POINT('Ctrl Pts',(-0.764978057881687,-1.,1.83948181064823));
#22086=CARTESIAN_POINT('Ctrl Pts',(-0.764602549687845,-1.,1.8334207722714));
#22087=CARTESIAN_POINT('Ctrl Pts',(-0.764165902606055,-1.,1.8273599120008));
#22088=CARTESIAN_POINT('Ctrl Pts',(-0.763673465462854,-1.,1.82131873145297));
#22089=CARTESIAN_POINT('Ctrl Pts',(-0.763132003836783,-1.,1.81532118405566));
#22090=CARTESIAN_POINT('Ctrl Pts',(-0.762546129464036,-1.,1.80938551463989));
#22091=CARTESIAN_POINT('Ctrl Pts',(-0.761915336443516,-1.,1.80351583877334));
#22092=CARTESIAN_POINT('Ctrl Pts',(-0.761229695230359,-1.,1.79768986997735));
#22093=CARTESIAN_POINT('Ctrl Pts',(-0.760469555880425,-1.,1.79185815610802));
#22094=CARTESIAN_POINT('Ctrl Pts',(-0.759614401109868,-1.,1.78596964884526));
#22095=CARTESIAN_POINT('Ctrl Pts',(-0.75865062667738,-1.,1.77999411220912));
#22096=CARTESIAN_POINT('Ctrl Pts',(-0.757578264077238,-1.,1.77394167108342));
#22097=CARTESIAN_POINT('Ctrl Pts',(-0.756421896028403,-1.,1.76789396003141));
#22098=CARTESIAN_POINT('Ctrl Pts',(-0.755220979975262,-1.,1.7619781724032));
#22099=CARTESIAN_POINT('Ctrl Pts',(-0.75400925402848,-1.,1.75631083600175));
#22100=CARTESIAN_POINT('Ctrl Pts',(-0.752797683531377,-1.,1.75095139468809));
#22101=CARTESIAN_POINT('Ctrl Pts',(-0.751555614163629,-1.,1.74585086852298));
#22102=CARTESIAN_POINT('Ctrl Pts',(-0.75019343597954,-1.,1.74080458266705));
#22103=CARTESIAN_POINT('Ctrl Pts',(-0.748582462954855,-1.,1.73550351679848));
#22104=CARTESIAN_POINT('Ctrl Pts',(-0.746574710096436,-1.,1.72958533647399));
#22105=CARTESIAN_POINT('Ctrl Pts',(-0.744021445433764,-1.,1.7226822991693));
#22106=CARTESIAN_POINT('Ctrl Pts',(-0.740795162032088,-1.,1.71447789751927));
#22107=CARTESIAN_POINT('Ctrl Pts',(-0.736799665724771,-1.,1.70473309006121));
#22108=CARTESIAN_POINT('Ctrl Pts',(-0.731963238697195,-1.,1.69326921975743));
#22109=CARTESIAN_POINT('Ctrl Pts',(-0.726235967997433,-1.,1.67996158455503));
#22110=CARTESIAN_POINT('Ctrl Pts',(-0.719585433804282,-1.,1.6647288055568));
#22111=CARTESIAN_POINT('Ctrl Pts',(-0.711993139355394,-1.,1.64752408832016));
#22112=CARTESIAN_POINT('Ctrl Pts',(-0.705159151988319,-1.,1.63216541664676));
#22113=CARTESIAN_POINT('Ctrl Pts',(-0.699605146405088,-1.,1.61974673472612));
#22114=CARTESIAN_POINT('Ctrl Pts',(-0.695712097881194,-1.,1.61106790958151));
#22115=CARTESIAN_POINT('Ctrl Pts',(-0.693717979106306,-1.,1.60662857109684));
#22116=CARTESIAN_POINT('',(-0.892032620296855,-1.,1.5055822144029));
#22117=CARTESIAN_POINT('Origin',(0.,-1.,0.));
#22118=CARTESIAN_POINT('',(-1.23627494547115,-1.,1.81978687191668));
#22119=CARTESIAN_POINT('Ctrl Pts',(-0.892032620296855,-1.,1.5055822144029));
#22120=CARTESIAN_POINT('Ctrl Pts',(-0.894452006964543,-1.,1.50980486806688));
#22121=CARTESIAN_POINT('Ctrl Pts',(-0.899185047483511,-1.,1.51805569590094));
#22122=CARTESIAN_POINT('Ctrl Pts',(-0.905967409625651,-1.,1.52984849887993));
#22123=CARTESIAN_POINT('Ctrl Pts',(-0.914375919026456,-1.,1.54440491149498));
#22124=CARTESIAN_POINT('Ctrl Pts',(-0.923832188944341,-1.,1.56065988578893));
#22125=CARTESIAN_POINT('Ctrl Pts',(-0.932246680108685,-1.,1.57499388382243));
#22126=CARTESIAN_POINT('Ctrl Pts',(-0.939646377893399,-1.,1.58744937487176));
#22127=CARTESIAN_POINT('Ctrl Pts',(-0.946078063315257,-1.,1.59810042043673));
#22128=CARTESIAN_POINT('Ctrl Pts',(-0.951613284356035,-1.,1.60706069896936));
#22129=CARTESIAN_POINT('Ctrl Pts',(-0.956354422920671,-1.,1.61449324337085));
#22130=CARTESIAN_POINT('Ctrl Pts',(-0.960438326101729,-1.,1.62061638140221));
#22131=CARTESIAN_POINT('Ctrl Pts',(-0.964046107040536,-1.,1.62571930670187));
#22132=CARTESIAN_POINT('Ctrl Pts',(-0.967387853230345,-1.,1.63013849959461));
#22133=CARTESIAN_POINT('Ctrl Pts',(-0.970669715997509,-1.,1.63420665729798));
#22134=CARTESIAN_POINT('Ctrl Pts',(-0.974066058287418,-1.,1.63820952658144));
#22135=CARTESIAN_POINT('Ctrl Pts',(-0.977689794119416,-1.,1.64233990826687));
#22136=CARTESIAN_POINT('Ctrl Pts',(-0.981562530939489,-1.,1.64665139190656));
#22137=CARTESIAN_POINT('Ctrl Pts',(-0.985642622920821,-1.,1.65110016612638));
#22138=CARTESIAN_POINT('Ctrl Pts',(-0.989855627854165,-1.,1.65559044289699));
#22139=CARTESIAN_POINT('Ctrl Pts',(-0.994121836661306,-1.,1.66001553809947));
#22140=CARTESIAN_POINT('Ctrl Pts',(-0.998389654952758,-1.,1.66430758030376));
#22141=CARTESIAN_POINT('Ctrl Pts',(-1.00265091003727,-1.,1.66846059277303));
#22142=CARTESIAN_POINT('Ctrl Pts',(-1.00692206696414,-1.,1.67250335383293));
#22143=CARTESIAN_POINT('Ctrl Pts',(-1.01123236493511,-1.,1.67648246776464));
#22144=CARTESIAN_POINT('Ctrl Pts',(-1.01561026162773,-1.,1.68044289894798));
#22145=CARTESIAN_POINT('Ctrl Pts',(-1.02006795074201,-1.,1.68440578021706));
#22146=CARTESIAN_POINT('Ctrl Pts',(-1.02460180535255,-1.,1.68836910178447));
#22147=CARTESIAN_POINT('Ctrl Pts',(-1.02919977579147,-1.,1.69231840863458));
#22148=CARTESIAN_POINT('Ctrl Pts',(-1.03384646003588,-1.,1.69623414782771));
#22149=CARTESIAN_POINT('Ctrl Pts',(-1.03852922490789,-1.,1.70010052930962));
#22150=CARTESIAN_POINT('Ctrl Pts',(-1.04324363334554,-1.,1.70391338707982));
#22151=CARTESIAN_POINT('Ctrl Pts',(-1.04799085404995,-1.,1.70767646263649));
#22152=CARTESIAN_POINT('Ctrl Pts',(-1.05277517202855,-1.,1.71139783543989));
#22153=CARTESIAN_POINT('Ctrl Pts',(-1.05760163192479,-1.,1.7150865442702));
#22154=CARTESIAN_POINT('Ctrl Pts',(-1.06247324680647,-1.,1.71874858456904));
#22155=CARTESIAN_POINT('Ctrl Pts',(-1.06738966975462,-1.,1.72238500928453));
#22156=CARTESIAN_POINT('Ctrl Pts',(-1.07234866990252,-1.,1.72599406198488));
#22157=CARTESIAN_POINT('Ctrl Pts',(-1.0773470373727,-1.,1.72957248977424));
#22158=CARTESIAN_POINT('Ctrl Pts',(-1.08238162784749,-1.,1.73311705663407));
#22159=CARTESIAN_POINT('Ctrl Pts',(-1.08745056285427,-1.,1.73662628326091));
#22160=CARTESIAN_POINT('Ctrl Pts',(-1.09255329056493,-1.,1.74010053962247));
#22161=CARTESIAN_POINT('Ctrl Pts',(-1.09768999241225,-1.,1.74354119236208));
#22162=CARTESIAN_POINT('Ctrl Pts',(-1.10286118991143,-1.,1.74695004214923));
#22163=CARTESIAN_POINT('Ctrl Pts',(-1.10806728183007,-1.,1.7503286607592));
#22164=CARTESIAN_POINT('Ctrl Pts',(-1.11330807582551,-1.,1.7536777209463));
#22165=CARTESIAN_POINT('Ctrl Pts',(-1.11858293216763,-1.,1.75699720772105));
#22166=CARTESIAN_POINT('Ctrl Pts',(-1.12389096855086,-1.,1.76028671825096));
#22167=CARTESIAN_POINT('Ctrl Pts',(-1.12923123555075,-1.,1.7635457196617));
#22168=CARTESIAN_POINT('Ctrl Pts',(-1.1346029180462,-1.,1.76677384551862));
#22169=CARTESIAN_POINT('Ctrl Pts',(-1.14000548336975,-1.,1.76997111386769));
#22170=CARTESIAN_POINT('Ctrl Pts',(-1.1454385822692,-1.,1.77313777896194));
#22171=CARTESIAN_POINT('Ctrl Pts',(-1.15090197841515,-1.,1.7762742255701));
#22172=CARTESIAN_POINT('Ctrl Pts',(-1.15639547194698,-1.,1.77938085564275));
#22173=CARTESIAN_POINT('Ctrl Pts',(-1.16191881298499,-1.,1.78245795881009));
#22174=CARTESIAN_POINT('Ctrl Pts',(-1.16747166312303,-1.,1.78550566040443));
#22175=CARTESIAN_POINT('Ctrl Pts',(-1.17305363177328,-1.,1.78852398877616));
#22176=CARTESIAN_POINT('Ctrl Pts',(-1.17866429440809,-1.,1.79151291552689));
#22177=CARTESIAN_POINT('Ctrl Pts',(-1.18430321697432,-1.,1.79447240321515));
#22178=CARTESIAN_POINT('Ctrl Pts',(-1.18996997934445,-1.,1.79740245923478));
#22179=CARTESIAN_POINT('Ctrl Pts',(-1.19566418930242,-1.,1.80030314369879));
#22180=CARTESIAN_POINT('Ctrl Pts',(-1.20138548938974,-1.,1.80317454838603));
#22181=CARTESIAN_POINT('Ctrl Pts',(-1.20713356605475,-1.,1.80601678480707));
#22182=CARTESIAN_POINT('Ctrl Pts',(-1.21290815708314,-1.,1.80882996917129));
#22183=CARTESIAN_POINT('Ctrl Pts',(-1.21870906103557,-1.,1.81161420806656));
#22184=CARTESIAN_POINT('Ctrl Pts',(-1.2245361330495,-1.,1.81436959210434));
#22185=CARTESIAN_POINT('Ctrl Pts',(-1.2292186489137,-1.,1.8165508718364));
#22186=CARTESIAN_POINT('Ctrl Pts',(-1.2327422452705,-1.,1.81817389921279));
#22187=CARTESIAN_POINT('Ctrl Pts',(-1.23509651170476,-1.,1.81925017193666));
#22188=CARTESIAN_POINT('Ctrl Pts',(-1.23627494547115,-1.,1.81978687191668));
#22189=CARTESIAN_POINT('',(-1.34869019493419,-1.,1.73811241238545));
#22190=CARTESIAN_POINT('',(-1.23627494547115,-1.,1.81978687191668));
#22191=CARTESIAN_POINT('',(-1.15624053661742,-1.,1.31362392696032));
#22192=CARTESIAN_POINT('Ctrl Pts',(-1.34869019493419,-1.,1.73811241238545));
#22193=CARTESIAN_POINT('Ctrl Pts',(-1.34854391898045,-1.,1.73682580585691));
#22194=CARTESIAN_POINT('Ctrl Pts',(-1.34824783112887,-1.,1.73425417885907));
#22195=CARTESIAN_POINT('Ctrl Pts',(-1.34779309152035,-1.,1.7304014965394));
#22196=CARTESIAN_POINT('Ctrl Pts',(-1.34716554819527,-1.,1.72527410680674));
#22197=CARTESIAN_POINT('Ctrl Pts',(-1.34634568653227,-1.,1.7188807715049));
#22198=CARTESIAN_POINT('Ctrl Pts',(-1.34549029589416,-1.,1.71250340686822));
#22199=CARTESIAN_POINT('Ctrl Pts',(-1.34459924533831,-1.,1.70614212266738));
#22200=CARTESIAN_POINT('Ctrl Pts',(-1.34367237124483,-1.,1.69979707754427));
#22201=CARTESIAN_POINT('Ctrl Pts',(-1.34270948206319,-1.,1.6934684849687));
#22202=CARTESIAN_POINT('Ctrl Pts',(-1.341710374848,-1.,1.68715660868764));
#22203=CARTESIAN_POINT('Ctrl Pts',(-1.34067485185203,-1.,1.68086176030362));
#22204=CARTESIAN_POINT('Ctrl Pts',(-1.3396027347034,-1.,1.67458429426086));
#22205=CARTESIAN_POINT('Ctrl Pts',(-1.33849388654388,-1.,1.66832460783989));
#22206=CARTESIAN_POINT('Ctrl Pts',(-1.33734820885262,-1.,1.66208312541983));
#22207=CARTESIAN_POINT('Ctrl Pts',(-1.33616559745172,-1.,1.65586025952593));
#22208=CARTESIAN_POINT('Ctrl Pts',(-1.33494590467993,-1.,1.6496563728683));
#22209=CARTESIAN_POINT('Ctrl Pts',(-1.33368890676572,-1.,1.6434717485603));
#22210=CARTESIAN_POINT('Ctrl Pts',(-1.33239425103724,-1.,1.63730653475089));
#22211=CARTESIAN_POINT('Ctrl Pts',(-1.33106149345645,-1.,1.63116079730923));
#22212=CARTESIAN_POINT('Ctrl Pts',(-1.3296901950568,-1.,1.62503464209797));
#22213=CARTESIAN_POINT('Ctrl Pts',(-1.32828000610449,-1.,1.61892832270724));
#22214=CARTESIAN_POINT('Ctrl Pts',(-1.32683074483356,-1.,1.6128423401575));
#22215=CARTESIAN_POINT('Ctrl Pts',(-1.32534250785782,-1.,1.60677758290954));
#22216=CARTESIAN_POINT('Ctrl Pts',(-1.32381550858256,-1.,1.60073511858687));
#22217=CARTESIAN_POINT('Ctrl Pts',(-1.32224985747682,-1.,1.59471591079403));
#22218=CARTESIAN_POINT('Ctrl Pts',(-1.32064537110892,-1.,1.58872057258245));
#22219=CARTESIAN_POINT('Ctrl Pts',(-1.31900135021432,-1.,1.58274907898834));
#22220=CARTESIAN_POINT('Ctrl Pts',(-1.31731642317187,-1.,1.5768005650559));
#22221=CARTESIAN_POINT('Ctrl Pts',(-1.31558903860016,-1.,1.57087397835723));
#22222=CARTESIAN_POINT('Ctrl Pts',(-1.31381795281002,-1.,1.56496872402353));
#22223=CARTESIAN_POINT('Ctrl Pts',(-1.31200264341696,-1.,1.55908521254821));
#22224=CARTESIAN_POINT('Ctrl Pts',(-1.31014393684222,-1.,1.55322568759481));
#22225=CARTESIAN_POINT('Ctrl Pts',(-1.30824393907473,-1.,1.54739413957185));
#22226=CARTESIAN_POINT('Ctrl Pts',(-1.30630475189556,-1.,1.54159462645432));
#22227=CARTESIAN_POINT('Ctrl Pts',(-1.30432735639489,-1.,1.53582981268977));
#22228=CARTESIAN_POINT('Ctrl Pts',(-1.30231064395568,-1.,1.53009970283891));
#22229=CARTESIAN_POINT('Ctrl Pts',(-1.30024984366328,-1.,1.52439957861062));
#22230=CARTESIAN_POINT('Ctrl Pts',(-1.29813791800747,-1.,1.51872184912724));
#22231=CARTESIAN_POINT('Ctrl Pts',(-1.29596850710509,-1.,1.51305994241402));
#22232=CARTESIAN_POINT('Ctrl Pts',(-1.29373841372842,-1.,1.50741159078365));
#22233=CARTESIAN_POINT('Ctrl Pts',(-1.29145022885181,-1.,1.50178230149776));
#22234=CARTESIAN_POINT('Ctrl Pts',(-1.28911506584254,-1.,1.49618896881754));
#22235=CARTESIAN_POINT('Ctrl Pts',(-1.2867467611644,-1.,1.4906522831278));
#22236=CARTESIAN_POINT('Ctrl Pts',(-1.28435533880201,-1.,1.4851881711891));
#22237=CARTESIAN_POINT('Ctrl Pts',(-1.28194158939517,-1.,1.47980070347095));
#22238=CARTESIAN_POINT('Ctrl Pts',(-1.2794891824849,-1.,1.4744717526707));
#22239=CARTESIAN_POINT('Ctrl Pts',(-1.27696414831089,-1.,1.46916035917133));
#22240=CARTESIAN_POINT('Ctrl Pts',(-1.27433119897822,-1.,1.46382431332476));
#22241=CARTESIAN_POINT('Ctrl Pts',(-1.27156805265289,-1.,1.45843906294697));
#22242=CARTESIAN_POINT('Ctrl Pts',(-1.2686778680489,-1.,1.45301422764247));
#22243=CARTESIAN_POINT('Ctrl Pts',(-1.26570925118868,-1.,1.44761985001662));
#22244=CARTESIAN_POINT('Ctrl Pts',(-1.26273903323859,-1.,1.44236470511303));
#22245=CARTESIAN_POINT('Ctrl Pts',(-1.25983531012005,-1.,1.43734919180848));
#22246=CARTESIAN_POINT('Ctrl Pts',(-1.25702687965755,-1.,1.43262645609691));
#22247=CARTESIAN_POINT('Ctrl Pts',(-1.25426945222639,-1.,1.42815938799387));
#22248=CARTESIAN_POINT('Ctrl Pts',(-1.2514145557001,-1.,1.42378102115575));
#22249=CARTESIAN_POINT('Ctrl Pts',(-1.24824430986571,-1.,1.41923722596025));
#22250=CARTESIAN_POINT('Ctrl Pts',(-1.24450600513056,-1.,1.41422913175179));
#22251=CARTESIAN_POINT('Ctrl Pts',(-1.23994455029534,-1.,1.40845295531283));
#22252=CARTESIAN_POINT('Ctrl Pts',(-1.23434087290423,-1.,1.40164708206106));
#22253=CARTESIAN_POINT('Ctrl Pts',(-1.22752961899387,-1.,1.39361389568796));
#22254=CARTESIAN_POINT('Ctrl Pts',(-1.21938737280852,-1.,1.38420564527715));
#22255=CARTESIAN_POINT('Ctrl Pts',(-1.20982812925645,-1.,1.37331915607905));
#22256=CARTESIAN_POINT('Ctrl Pts',(-1.1987959077932,-1.,1.36088705043885));
#22257=CARTESIAN_POINT('Ctrl Pts',(-1.18625865667441,-1.,1.34687054001093));
#22258=CARTESIAN_POINT('Ctrl Pts',(-1.17501305789857,-1.,1.33437539347008));
#22259=CARTESIAN_POINT('Ctrl Pts',(-1.16589330093588,-1.,1.32428080721772));
#22260=CARTESIAN_POINT('Ctrl Pts',(-1.15950888730809,-1.,1.31722977216397));
#22261=CARTESIAN_POINT('Ctrl Pts',(-1.15624053661742,-1.,1.31362392696032));
#22262=CARTESIAN_POINT('',(-1.31362392696033,-1.,1.15624053661742));
#22263=CARTESIAN_POINT('Origin',(0.,-1.,0.));
#22264=CARTESIAN_POINT('',(-1.73811241238545,-1.,1.34869019493419));
#22265=CARTESIAN_POINT('Ctrl Pts',(-1.31362392696033,-1.,1.15624053661742));
#22266=CARTESIAN_POINT('Ctrl Pts',(-1.3172297721596,-1.,1.15950888730433));
#22267=CARTESIAN_POINT('Ctrl Pts',(-1.32428080720544,-1.,1.16589330092532));
#22268=CARTESIAN_POINT('Ctrl Pts',(-1.33437539344842,-1.,1.17501305787994));
#22269=CARTESIAN_POINT('Ctrl Pts',(-1.34687053998157,-1.,1.18625865664915));
#22270=CARTESIAN_POINT('Ctrl Pts',(-1.36088705040677,-1.,1.1987959077656));
#22271=CARTESIAN_POINT('Ctrl Pts',(-1.37331915604962,-1.,1.20982812923113));
#22272=CARTESIAN_POINT('Ctrl Pts',(-1.38420564525391,-1.,1.21938737278853));
#22273=CARTESIAN_POINT('Ctrl Pts',(-1.39361389567257,-1.,1.22752961898063));
#22274=CARTESIAN_POINT('Ctrl Pts',(-1.40164708205345,-1.,1.23434087289768));
#22275=CARTESIAN_POINT('Ctrl Pts',(-1.40845295531151,-1.,1.23994455029421));
#22276=CARTESIAN_POINT('Ctrl Pts',(-1.41422913175437,-1.,1.24450600513278));
#22277=CARTESIAN_POINT('Ctrl Pts',(-1.41923722596421,-1.,1.24824430986911));
#22278=CARTESIAN_POINT('Ctrl Pts',(-1.42378102115911,-1.,1.25141455570299));
#22279=CARTESIAN_POINT('Ctrl Pts',(-1.42815938799555,-1.,1.25426945222783));
#22280=CARTESIAN_POINT('Ctrl Pts',(-1.43262645609679,-1.,1.25702687965744));
#22281=CARTESIAN_POINT('Ctrl Pts',(-1.43734919180719,-1.,1.25983531011894));
#22282=CARTESIAN_POINT('Ctrl Pts',(-1.44236470511145,-1.,1.26273903323723));
#22283=CARTESIAN_POINT('Ctrl Pts',(-1.44761985001544,-1.,1.26570925118767));
#22284=CARTESIAN_POINT('Ctrl Pts',(-1.45301422764205,-1.,1.26867786804854));
#22285=CARTESIAN_POINT('Ctrl Pts',(-1.45843906294725,-1.,1.27156805265312));
#22286=CARTESIAN_POINT('Ctrl Pts',(-1.4638243133254,-1.,1.27433119897877));
#22287=CARTESIAN_POINT('Ctrl Pts',(-1.46916035917197,-1.,1.27696414831144));
#22288=CARTESIAN_POINT('Ctrl Pts',(-1.4744717526711,-1.,1.27948918248524));
#22289=CARTESIAN_POINT('Ctrl Pts',(-1.47980070347102,-1.,1.28194158939522));
#22290=CARTESIAN_POINT('Ctrl Pts',(-1.48518817118891,-1.,1.28435533880184));
#22291=CARTESIAN_POINT('Ctrl Pts',(-1.4906522831275,-1.,1.28674676116415));
#22292=CARTESIAN_POINT('Ctrl Pts',(-1.49618896881729,-1.,1.28911506584232));
#22293=CARTESIAN_POINT('Ctrl Pts',(-1.50178230149764,-1.,1.29145022885171));
#22294=CARTESIAN_POINT('Ctrl Pts',(-1.50741159078367,-1.,1.29373841372843));
#22295=CARTESIAN_POINT('Ctrl Pts',(-1.51305994241412,-1.,1.29596850710518));
#22296=CARTESIAN_POINT('Ctrl Pts',(-1.51872184912735,-1.,1.29813791800757));
#22297=CARTESIAN_POINT('Ctrl Pts',(-1.5243995786107,-1.,1.30024984366334));
#22298=CARTESIAN_POINT('Ctrl Pts',(-1.53009970283893,-1.,1.3023106439557));
#22299=CARTESIAN_POINT('Ctrl Pts',(-1.53582981268976,-1.,1.30432735639487));
#22300=CARTESIAN_POINT('Ctrl Pts',(-1.54159462645428,-1.,1.30630475189553));
#22301=CARTESIAN_POINT('Ctrl Pts',(-1.54739413957183,-1.,1.30824393907471));
#22302=CARTESIAN_POINT('Ctrl Pts',(-1.55322568759481,-1.,1.31014393684221));
#22303=CARTESIAN_POINT('Ctrl Pts',(-1.55908521254822,-1.,1.31200264341696));
#22304=CARTESIAN_POINT('Ctrl Pts',(-1.56496872402352,-1.,1.31381795281002));
#22305=CARTESIAN_POINT('Ctrl Pts',(-1.57087397835721,-1.,1.31558903860015));
#22306=CARTESIAN_POINT('Ctrl Pts',(-1.57680056505585,-1.,1.31731642317183));
#22307=CARTESIAN_POINT('Ctrl Pts',(-1.58274907898829,-1.,1.31900135021428));
#22308=CARTESIAN_POINT('Ctrl Pts',(-1.58872057258244,-1.,1.32064537110891));
#22309=CARTESIAN_POINT('Ctrl Pts',(-1.59471591079408,-1.,1.32224985747686));
#22310=CARTESIAN_POINT('Ctrl Pts',(-1.600735118587,-1.,1.32381550858266));
#22311=CARTESIAN_POINT('Ctrl Pts',(-1.6067775829097,-1.,1.32534250785794));
#22312=CARTESIAN_POINT('Ctrl Pts',(-1.61284234015762,-1.,1.32683074483365));
#22313=CARTESIAN_POINT('Ctrl Pts',(-1.61892832270723,-1.,1.32828000610448));
#22314=CARTESIAN_POINT('Ctrl Pts',(-1.62503464209777,-1.,1.32969019505665));
#22315=CARTESIAN_POINT('Ctrl Pts',(-1.63116079730887,-1.,1.33106149345618));
#22316=CARTESIAN_POINT('Ctrl Pts',(-1.6373065347505,-1.,1.33239425103694));
#22317=CARTESIAN_POINT('Ctrl Pts',(-1.64347174856007,-1.,1.33368890676554));
#22318=CARTESIAN_POINT('Ctrl Pts',(-1.64965637286843,-1.,1.33494590468003));
#22319=CARTESIAN_POINT('Ctrl Pts',(-1.65586025952651,-1.,1.33616559745217));
#22320=CARTESIAN_POINT('Ctrl Pts',(-1.66208312542073,-1.,1.33734820885331));
#22321=CARTESIAN_POINT('Ctrl Pts',(-1.66832460784078,-1.,1.33849388654458));
#22322=CARTESIAN_POINT('Ctrl Pts',(-1.67458429426126,-1.,1.33960273470372));
#22323=CARTESIAN_POINT('Ctrl Pts',(-1.68086176030308,-1.,1.3406748518516));
#22324=CARTESIAN_POINT('Ctrl Pts',(-1.68715660868602,-1.,1.34171037484673));
#22325=CARTESIAN_POINT('Ctrl Pts',(-1.6934684849664,-1.,1.34270948206139));
#22326=CARTESIAN_POINT('Ctrl Pts',(-1.69979707754221,-1.,1.34367237124322));
#22327=CARTESIAN_POINT('Ctrl Pts',(-1.70614212266676,-1.,1.34459924533783));
#22328=CARTESIAN_POINT('Ctrl Pts',(-1.71250340687011,-1.,1.34549029589563));
#22329=CARTESIAN_POINT('Ctrl Pts',(-1.7188807715095,-1.,1.34634568653586));
#22330=CARTESIAN_POINT('Ctrl Pts',(-1.72527410681298,-1.,1.34716554820013));
#22331=CARTESIAN_POINT('Ctrl Pts',(-1.73040149654497,-1.,1.3477930915247));
#22332=CARTESIAN_POINT('Ctrl Pts',(-1.73425417886255,-1.,1.34824783113158));
#22333=CARTESIAN_POINT('Ctrl Pts',(-1.73682580585819,-1.,1.34854391898145));
#22334=CARTESIAN_POINT('Ctrl Pts',(-1.73811241238545,-1.,1.34869019493419));
#22335=CARTESIAN_POINT('',(-1.81978687191668,-1.,1.23627494547115));
#22336=CARTESIAN_POINT('',(-1.73811241238545,-1.,1.34869019493419));
#22337=CARTESIAN_POINT('',(-1.5055822144029,-1.,0.892032620296855));
#22338=CARTESIAN_POINT('Ctrl Pts',(-1.81978687191668,-1.,1.23627494547115));
#22339=CARTESIAN_POINT('Ctrl Pts',(-1.81925017193531,-1.,1.23509651170384));
#22340=CARTESIAN_POINT('Ctrl Pts',(-1.81817389920914,-1.,1.23274224526804));
#22341=CARTESIAN_POINT('Ctrl Pts',(-1.81655087183054,-1.,1.22921864890975));
#22342=CARTESIAN_POINT('Ctrl Pts',(-1.81436959209778,-1.,1.22453613304507));
#22343=CARTESIAN_POINT('Ctrl Pts',(-1.81161420806172,-1.,1.2187090610323));
#22344=CARTESIAN_POINT('Ctrl Pts',(-1.80882996916931,-1.,1.2129081570818));
#22345=CARTESIAN_POINT('Ctrl Pts',(-1.80601678480772,-1.,1.20713356605519));
#22346=CARTESIAN_POINT('Ctrl Pts',(-1.8031745483882,-1.,1.2013854893912));
#22347=CARTESIAN_POINT('Ctrl Pts',(-1.80030314370121,-1.,1.19566418930405));
#22348=CARTESIAN_POINT('Ctrl Pts',(-1.79740245923649,-1.,1.1899699793456));
#22349=CARTESIAN_POINT('Ctrl Pts',(-1.79447240321572,-1.,1.18430321697471));
#22350=CARTESIAN_POINT('Ctrl Pts',(-1.79151291552646,-1.,1.17866429440781));
#22351=CARTESIAN_POINT('Ctrl Pts',(-1.78852398877523,-1.,1.17305363177265));
#22352=CARTESIAN_POINT('Ctrl Pts',(-1.78550566040349,-1.,1.16747166312239));
#22353=CARTESIAN_POINT('Ctrl Pts',(-1.78245795880949,-1.,1.16191881298458));
#22354=CARTESIAN_POINT('Ctrl Pts',(-1.77938085564261,-1.,1.15639547194689));
#22355=CARTESIAN_POINT('Ctrl Pts',(-1.77627422557034,-1.,1.15090197841531));
#22356=CARTESIAN_POINT('Ctrl Pts',(-1.77313777896234,-1.,1.14543858226948));
#22357=CARTESIAN_POINT('Ctrl Pts',(-1.76997111386806,-1.,1.14000548337));
#22358=CARTESIAN_POINT('Ctrl Pts',(-1.76677384551883,-1.,1.13460291804635));
#22359=CARTESIAN_POINT('Ctrl Pts',(-1.76354571966171,-1.,1.12923123555076));
#22360=CARTESIAN_POINT('Ctrl Pts',(-1.76028671825084,-1.,1.12389096855078));
#22361=CARTESIAN_POINT('Ctrl Pts',(-1.75699720772089,-1.,1.11858293216752));
#22362=CARTESIAN_POINT('Ctrl Pts',(-1.75367772094617,-1.,1.11330807582542));
#22363=CARTESIAN_POINT('Ctrl Pts',(-1.75032866075914,-1.,1.10806728183003));
#22364=CARTESIAN_POINT('Ctrl Pts',(-1.74695004214924,-1.,1.10286118991144));
#22365=CARTESIAN_POINT('Ctrl Pts',(-1.74354119236212,-1.,1.09768999241229));
#22366=CARTESIAN_POINT('Ctrl Pts',(-1.74010053962252,-1.,1.09255329056496));
#22367=CARTESIAN_POINT('Ctrl Pts',(-1.73662628326093,-1.,1.08745056285429));
#22368=CARTESIAN_POINT('Ctrl Pts',(-1.73311705663407,-1.,1.08238162784749));
#22369=CARTESIAN_POINT('Ctrl Pts',(-1.72957248977424,-1.,1.0773470373727));
#22370=CARTESIAN_POINT('Ctrl Pts',(-1.72599406198489,-1.,1.07234866990252));
#22371=CARTESIAN_POINT('Ctrl Pts',(-1.72238500928456,-1.,1.06738966975463));
#22372=CARTESIAN_POINT('Ctrl Pts',(-1.71874858456908,-1.,1.0624732468065));
#22373=CARTESIAN_POINT('Ctrl Pts',(-1.71508654427022,-1.,1.05760163192481));
#22374=CARTESIAN_POINT('Ctrl Pts',(-1.71139783543986,-1.,1.05277517202854));
#22375=CARTESIAN_POINT('Ctrl Pts',(-1.70767646263641,-1.,1.0479908540499));
#22376=CARTESIAN_POINT('Ctrl Pts',(-1.70391338707969,-1.,1.04324363334546));
#22377=CARTESIAN_POINT('Ctrl Pts',(-1.70010052930951,-1.,1.03852922490782));
#22378=CARTESIAN_POINT('Ctrl Pts',(-1.69623414782769,-1.,1.03384646003587));
#22379=CARTESIAN_POINT('Ctrl Pts',(-1.69231840863471,-1.,1.02919977579155));
#22380=CARTESIAN_POINT('Ctrl Pts',(-1.68836910178475,-1.,1.02460180535272));
#22381=CARTESIAN_POINT('Ctrl Pts',(-1.68440578021739,-1.,1.02006795074222));
#22382=CARTESIAN_POINT('Ctrl Pts',(-1.6804428989482,-1.,1.01561026162787));
#22383=CARTESIAN_POINT('Ctrl Pts',(-1.67648246776457,-1.,1.01123236493507));
#22384=CARTESIAN_POINT('Ctrl Pts',(-1.67250335383248,-1.,1.00692206696387));
#22385=CARTESIAN_POINT('Ctrl Pts',(-1.66846059277231,-1.,1.00265091003682));
#22386=CARTESIAN_POINT('Ctrl Pts',(-1.66430758030304,-1.,0.998389654952317));
#22387=CARTESIAN_POINT('Ctrl Pts',(-1.66001553809916,-1.,0.994121836661116));
#22388=CARTESIAN_POINT('Ctrl Pts',(-1.65559044289746,-1.,0.98985562785445));
#22389=CARTESIAN_POINT('Ctrl Pts',(-1.6511001661277,-1.,0.985642622921626));
#22390=CARTESIAN_POINT('Ctrl Pts',(-1.64665139190834,-1.,0.981562530940574));
#22391=CARTESIAN_POINT('Ctrl Pts',(-1.64233990826831,-1.,0.977689794120297));
#22392=CARTESIAN_POINT('Ctrl Pts',(-1.63820952658157,-1.,0.974066058287501));
#22393=CARTESIAN_POINT('Ctrl Pts',(-1.63420665729609,-1.,0.970669715996356));
#22394=CARTESIAN_POINT('Ctrl Pts',(-1.63013849959083,-1.,0.967387853228041));
#22395=CARTESIAN_POINT('Ctrl Pts',(-1.6257193066974,-1.,0.964046107037821));
#22396=CARTESIAN_POINT('Ctrl Pts',(-1.62061638139929,-1.,0.960438326099958));
#22397=CARTESIAN_POINT('Ctrl Pts',(-1.61449324337233,-1.,0.956354422921573));
#22398=CARTESIAN_POINT('Ctrl Pts',(-1.60706069897794,-1.,0.951613284361248));
#22399=CARTESIAN_POINT('Ctrl Pts',(-1.59810042045408,-1.,0.946078063325796));
#22400=CARTESIAN_POINT('Ctrl Pts',(-1.58744937489796,-1.,0.939646377909319));
#22401=CARTESIAN_POINT('Ctrl Pts',(-1.57499388385561,-1.,0.932246680128849));
#22402=CARTESIAN_POINT('Ctrl Pts',(-1.56065988582509,-1.,0.923832188966322));
#22403=CARTESIAN_POINT('Ctrl Pts',(-1.54440491152808,-1.,0.91437591904658));
#22404=CARTESIAN_POINT('Ctrl Pts',(-1.52984849890434,-1.,0.905967409640499));
#22405=CARTESIAN_POINT('Ctrl Pts',(-1.51805569591479,-1.,0.89918504749193));
#22406=CARTESIAN_POINT('Ctrl Pts',(-1.50980486807181,-1.,0.894452006967538));
#22407=CARTESIAN_POINT('Ctrl Pts',(-1.5055822144029,-1.,0.892032620296855));
#22408=CARTESIAN_POINT('',(-1.60662857109684,-1.,0.693717979106305));
#22409=CARTESIAN_POINT('Origin',(0.,-1.,0.));
#22410=CARTESIAN_POINT('',(-2.0698113262342,-1.,0.7455743247944));
#22411=CARTESIAN_POINT('Ctrl Pts',(-1.60662857109684,-1.,0.693717979106305));
#22412=CARTESIAN_POINT('Ctrl Pts',(-1.61106790957619,-1.,0.69571209787897));
#22413=CARTESIAN_POINT('Ctrl Pts',(-1.61974673471117,-1.,0.699605146398837));
#22414=CARTESIAN_POINT('Ctrl Pts',(-1.6321654166204,-1.,0.705159151977294));
#22415=CARTESIAN_POINT('Ctrl Pts',(-1.64752408828442,-1.,0.711993139340447));
#22416=CARTESIAN_POINT('Ctrl Pts',(-1.66472880551777,-1.,0.71958543378795));
#22417=CARTESIAN_POINT('Ctrl Pts',(-1.67996158451922,-1.,0.726235967982445));
#22418=CARTESIAN_POINT('Ctrl Pts',(-1.69326921972915,-1.,0.731963238685357));
#22419=CARTESIAN_POINT('Ctrl Pts',(-1.70473309004249,-1.,0.736799665716932));
#22420=CARTESIAN_POINT('Ctrl Pts',(-1.71447789751001,-1.,0.74079516202821));
#22421=CARTESIAN_POINT('Ctrl Pts',(-1.72268229916769,-1.,0.744021445433093));
#22422=CARTESIAN_POINT('Ctrl Pts',(-1.72958533647714,-1.,0.746574710097752));
#22423=CARTESIAN_POINT('Ctrl Pts',(-1.7355035168033,-1.,0.74858246295687));
#22424=CARTESIAN_POINT('Ctrl Pts',(-1.74080458267114,-1.,0.750193435981249));
#22425=CARTESIAN_POINT('Ctrl Pts',(-1.74585086852502,-1.,0.751555614164482));
#22426=CARTESIAN_POINT('Ctrl Pts',(-1.75095139468794,-1.,0.752797683531314));
#22427=CARTESIAN_POINT('Ctrl Pts',(-1.75631083600019,-1.,0.754009254027829));
#22428=CARTESIAN_POINT('Ctrl Pts',(-1.76197817240128,-1.,0.755220979974461));
#22429=CARTESIAN_POINT('Ctrl Pts',(-1.76789396002998,-1.,0.75642189602781));
#22430=CARTESIAN_POINT('Ctrl Pts',(-1.77394167108292,-1.,0.757578264077029));
#22431=CARTESIAN_POINT('Ctrl Pts',(-1.77999411220945,-1.,0.758650626677518));
#22432=CARTESIAN_POINT('Ctrl Pts',(-1.78596964884604,-1.,0.759614401110189));
#22433=CARTESIAN_POINT('Ctrl Pts',(-1.7918581561088,-1.,0.760469555880749));
#22434=CARTESIAN_POINT('Ctrl Pts',(-1.79768986997783,-1.,0.761229695230558));
#22435=CARTESIAN_POINT('Ctrl Pts',(-1.80351583877342,-1.,0.761915336443547));
#22436=CARTESIAN_POINT('Ctrl Pts',(-1.80938551463965,-1.,0.762546129463938));
#22437=CARTESIAN_POINT('Ctrl Pts',(-1.8153211840553,-1.,0.763132003836634));
#22438=CARTESIAN_POINT('Ctrl Pts',(-1.82131873145266,-1.,0.763673465462726));
#22439=CARTESIAN_POINT('Ctrl Pts',(-1.82735991200065,-1.,0.764165902605995));
#22440=CARTESIAN_POINT('Ctrl Pts',(-1.83342077227142,-1.,0.764602549687853));
#22441=CARTESIAN_POINT('Ctrl Pts',(-1.83948181064835,-1.,0.764978057881737));
#22442=CARTESIAN_POINT('Ctrl Pts',(-1.84553698875924,-1.,0.765291664862029));
#22443=CARTESIAN_POINT('Ctrl Pts',(-1.85158945130063,-1.,0.765545710619062));
#22444=CARTESIAN_POINT('Ctrl Pts',(-1.85764741390394,-1.,0.765744212909318));
#22445=CARTESIAN_POINT('Ctrl Pts',(-1.86372027063312,-1.,0.765891519092547));
#22446=CARTESIAN_POINT('Ctrl Pts',(-1.86981398314341,-1.,0.765990708546091));
#22447=CARTESIAN_POINT('Ctrl Pts',(-1.87592888967883,-1.,0.766042837036744));
#22448=CARTESIAN_POINT('Ctrl Pts',(-1.88206215302561,-1.,0.766047794851864));
#22449=CARTESIAN_POINT('Ctrl Pts',(-1.88820926433409,-1.,0.766004837062091));
#22450=CARTESIAN_POINT('Ctrl Pts',(-1.89436577771388,-1.,0.765913193856978));
#22451=CARTESIAN_POINT('Ctrl Pts',(-1.90052930393596,-1.,0.765772772593386));
#22452=CARTESIAN_POINT('Ctrl Pts',(-1.90669961402356,-1.,0.765584196937919));
#22453=CARTESIAN_POINT('Ctrl Pts',(-1.91287765805169,-1.,0.765348465884722));
#22454=CARTESIAN_POINT('Ctrl Pts',(-1.91906491634196,-1.,0.765066729667088));
#22455=CARTESIAN_POINT('Ctrl Pts',(-1.92526263537048,-1.,0.764740025488211));
#22456=CARTESIAN_POINT('Ctrl Pts',(-1.93147105496382,-1.,0.76436901067394));
#22457=CARTESIAN_POINT('Ctrl Pts',(-1.93768964875886,-1.,0.763954049121458));
#22458=CARTESIAN_POINT('Ctrl Pts',(-1.9439174661764,-1.,0.763495333538629));
#22459=CARTESIAN_POINT('Ctrl Pts',(-1.95015342590024,-1.,0.762992990878769));
#22460=CARTESIAN_POINT('Ctrl Pts',(-1.95639665309869,-1.,0.762447203806179));
#22461=CARTESIAN_POINT('Ctrl Pts',(-1.96264672744186,-1.,0.761858300014423));
#22462=CARTESIAN_POINT('Ctrl Pts',(-1.96890351582499,-1.,0.76122669048382));
#22463=CARTESIAN_POINT('Ctrl Pts',(-1.97516705321494,-1.,0.760552825409757));
#22464=CARTESIAN_POINT('Ctrl Pts',(-1.98143741418172,-1.,0.75983714745219));
#22465=CARTESIAN_POINT('Ctrl Pts',(-1.98771456680874,-1.,0.759080037802488));
#22466=CARTESIAN_POINT('Ctrl Pts',(-1.99399831098817,-1.,0.758281796766761));
#22467=CARTESIAN_POINT('Ctrl Pts',(-2.00028834739178,-1.,0.757442676862724));
#22468=CARTESIAN_POINT('Ctrl Pts',(-2.0065843158773,-1.,0.75656290464667));
#22469=CARTESIAN_POINT('Ctrl Pts',(-2.01288584328084,-1.,0.755642704957865));
#22470=CARTESIAN_POINT('Ctrl Pts',(-2.01919259405809,-1.,0.754682330722816));
#22471=CARTESIAN_POINT('Ctrl Pts',(-2.02550428623313,-1.,0.753682061112768));
#22472=CARTESIAN_POINT('Ctrl Pts',(-2.03182068456221,-1.,0.752642180487211));
#22473=CARTESIAN_POINT('Ctrl Pts',(-2.03814160092099,-1.,0.751562963361115));
#22474=CARTESIAN_POINT('Ctrl Pts',(-2.04446689147979,-1.,0.750444657875576));
#22475=CARTESIAN_POINT('Ctrl Pts',(-2.05079645592154,-1.,0.749287468665046));
#22476=CARTESIAN_POINT('Ctrl Pts',(-2.05713023031006,-1.,0.748091554183802));
#22477=CARTESIAN_POINT('Ctrl Pts',(-2.06220058927826,-1.,0.747103932787919));
#22478=CARTESIAN_POINT('Ctrl Pts',(-2.06600523016815,-1.,0.7463458715442));
#22479=CARTESIAN_POINT('Ctrl Pts',(-2.06854248895728,-1.,0.745832791378367));
#22480=CARTESIAN_POINT('Ctrl Pts',(-2.0698113262342,-1.,0.7455743247944));
#22481=CARTESIAN_POINT('',(-2.11275013067528,-1.,0.61342227326009));
#22482=CARTESIAN_POINT('',(-2.0698113262342,-1.,0.7455743247944));
#22483=CARTESIAN_POINT('',(-1.7075470150345,-1.,0.383122945602004));
#22484=CARTESIAN_POINT('Ctrl Pts',(-2.11275013067528,-1.,0.61342227326009));
#22485=CARTESIAN_POINT('Ctrl Pts',(-2.11187554259986,-1.,0.6124673655618));
#22486=CARTESIAN_POINT('Ctrl Pts',(-2.11012443807238,-1.,0.610560911689899));
#22487=CARTESIAN_POINT('Ctrl Pts',(-2.1074919961518,-1.,0.607711315454876));
#22488=CARTESIAN_POINT('Ctrl Pts',(-2.10397049886949,-1.,0.60393203073603));
#22489=CARTESIAN_POINT('Ctrl Pts',(-2.0995493086477,-1.,0.599241616420533));
#22490=CARTESIAN_POINT('Ctrl Pts',(-2.0951087622027,-1.,0.594585006052162));
#22491=CARTESIAN_POINT('Ctrl Pts',(-2.09064881812129,-1.,0.589962365403406));
#22492=CARTESIAN_POINT('Ctrl Pts',(-2.08616943727951,-1.,0.585373918991617));
#22493=CARTESIAN_POINT('Ctrl Pts',(-2.08167059018418,-1.,0.580819952108063));
#22494=CARTESIAN_POINT('Ctrl Pts',(-2.07715226767559,-1.,0.576300797416844));
#22495=CARTESIAN_POINT('Ctrl Pts',(-2.07261449292824,-1.,0.571816823242603));
#22496=CARTESIAN_POINT('Ctrl Pts',(-2.06805732997334,-1.,0.567368421181087));
#22497=CARTESIAN_POINT('Ctrl Pts',(-2.06348090160589,-1.,0.562955993082261));
#22498=CARTESIAN_POINT('Ctrl Pts',(-2.05888537756462,-1.,0.558579940185151));
#22499=CARTESIAN_POINT('Ctrl Pts',(-2.05427091604413,-1.,0.554240657463906));
#22500=CARTESIAN_POINT('Ctrl Pts',(-2.04963761077958,-1.,0.549938525150295));
#22501=CARTESIAN_POINT('Ctrl Pts',(-2.04498544714588,-1.,0.54567390381743));
#22502=CARTESIAN_POINT('Ctrl Pts',(-2.04031422690527,-1.,0.541447120615659));
#22503=CARTESIAN_POINT('Ctrl Pts',(-2.03562362954037,-1.,0.537258489833262));
#22504=CARTESIAN_POINT('Ctrl Pts',(-2.03091336214426,-1.,0.533108355132976));
#22505=CARTESIAN_POINT('Ctrl Pts',(-2.0261832908329,-1.,0.528997127241914));
#22506=CARTESIAN_POINT('Ctrl Pts',(-2.02143356304698,-1.,0.524925318333476));
#22507=CARTESIAN_POINT('Ctrl Pts',(-2.01666477917286,-1.,0.52089359039937));
#22508=CARTESIAN_POINT('Ctrl Pts',(-2.01187773939242,-1.,0.516902681728687));
#22509=CARTESIAN_POINT('Ctrl Pts',(-2.00707309946949,-1.,0.512953306961792));
#22510=CARTESIAN_POINT('Ctrl Pts',(-2.00225107134734,-1.,0.509046069886157));
#22511=CARTESIAN_POINT('Ctrl Pts',(-1.99741107463572,-1.,0.505181361323026));
#22512=CARTESIAN_POINT('Ctrl Pts',(-1.99255149126155,-1.,0.501359287727146));
#22513=CARTESIAN_POINT('Ctrl Pts',(-1.98767044752932,-1.,0.497579909545574));
#22514=CARTESIAN_POINT('Ctrl Pts',(-1.98276658761821,-1.,0.493843476541494));
#22515=CARTESIAN_POINT('Ctrl Pts',(-1.97783973019229,-1.,0.490150627860952));
#22516=CARTESIAN_POINT('Ctrl Pts',(-1.97289186263272,-1.,0.486502692907659));
#22517=CARTESIAN_POINT('Ctrl Pts',(-1.96792703422362,-1.,0.48290166212069));
#22518=CARTESIAN_POINT('Ctrl Pts',(-1.96294933055943,-1.,0.479349583074855));
#22519=CARTESIAN_POINT('Ctrl Pts',(-1.95796111148177,-1.,0.475848034683176));
#22520=CARTESIAN_POINT('Ctrl Pts',(-1.95296148278133,-1.,0.472397672264072));
#22521=CARTESIAN_POINT('Ctrl Pts',(-1.94794381136514,-1.,0.468997482913135));
#22522=CARTESIAN_POINT('Ctrl Pts',(-1.9428979419619,-1.,0.46564546202603));
#22523=CARTESIAN_POINT('Ctrl Pts',(-1.93781486640821,-1.,0.462340031009056));
#22524=CARTESIAN_POINT('Ctrl Pts',(-1.93269066517934,-1.,0.459081234547926));
#22525=CARTESIAN_POINT('Ctrl Pts',(-1.92753067150476,-1.,0.455872005174371));
#22526=CARTESIAN_POINT('Ctrl Pts',(-1.92235380648502,-1.,0.452719478359432));
#22527=CARTESIAN_POINT('Ctrl Pts',(-1.91718342555755,-1.,0.449632260106662));
#22528=CARTESIAN_POINT('Ctrl Pts',(-1.9120369998112,-1.,0.446617343485711));
#22529=CARTESIAN_POINT('Ctrl Pts',(-1.90691756144898,-1.,0.44367755684915));
#22530=CARTESIAN_POINT('Ctrl Pts',(-1.90180124389086,-1.,0.440807833704038));
#22531=CARTESIAN_POINT('Ctrl Pts',(-1.89663648956466,-1.,0.437995003948244));
#22532=CARTESIAN_POINT('Ctrl Pts',(-1.89136993975504,-1.,0.435225660963383));
#22533=CARTESIAN_POINT('Ctrl Pts',(-1.88596913666793,-1.,0.432493038548748));
#22534=CARTESIAN_POINT('Ctrl Pts',(-1.88044229001832,-1.,0.429803062482344));
#22535=CARTESIAN_POINT('Ctrl Pts',(-1.87486989291484,-1.,0.427183828519102));
#22536=CARTESIAN_POINT('Ctrl Pts',(-1.86937803944323,-1.,0.424678177291359));
#22537=CARTESIAN_POINT('Ctrl Pts',(-1.86408083334028,-1.,0.422327307418275));
#22538=CARTESIAN_POINT('Ctrl Pts',(-1.85903281096686,-1.,0.420157287975619));
#22539=CARTESIAN_POINT('Ctrl Pts',(-1.85417632856234,-1.,0.418164129143534));
#22540=CARTESIAN_POINT('Ctrl Pts',(-1.84929312929882,-1.,0.416300022038864));
#22541=CARTESIAN_POINT('Ctrl Pts',(-1.8440575707371,-1.,0.41448743825434));
#22542=CARTESIAN_POINT('Ctrl Pts',(-1.83808953475839,-1.,0.412633125322161));
#22543=CARTESIAN_POINT('Ctrl Pts',(-1.83100408895216,-1.,0.410641256301675));
#22544=CARTESIAN_POINT('Ctrl Pts',(-1.8224702267854,-1.,0.408428948108533));
#22545=CARTESIAN_POINT('Ctrl Pts',(-1.81223801813988,-1.,0.405933518411838));
#22546=CARTESIAN_POINT('Ctrl Pts',(-1.80012077176221,-1.,0.403107976170441));
#22547=CARTESIAN_POINT('Ctrl Pts',(-1.78598826347533,-1.,0.39991940378308));
#22548=CARTESIAN_POINT('Ctrl Pts',(-1.7697556004756,-1.,0.39634619612042));
#22549=CARTESIAN_POINT('Ctrl Pts',(-1.75137405313962,-1.,0.392375812294307));
#22550=CARTESIAN_POINT('Ctrl Pts',(-1.7349317097561,-1.,0.388877023509191));
#22551=CARTESIAN_POINT('Ctrl Pts',(-1.72162022246158,-1.,0.38607079032701));
#22552=CARTESIAN_POINT('Ctrl Pts',(-1.71231062891958,-1.,0.384119047315542));
#22553=CARTESIAN_POINT('Ctrl Pts',(-1.7075470150345,-1.,0.383122945602004));
#22554=CARTESIAN_POINT('',(-1.74236521665491,-1.,0.163289472382896));
#22555=CARTESIAN_POINT('Origin',(0.,-1.,0.));
#22556=CARTESIAN_POINT('',(-2.19890268624765,-1.,0.069476445021958));
#22557=CARTESIAN_POINT('Ctrl Pts',(-1.74236521665491,-1.,0.163289472382896));
#22558=CARTESIAN_POINT('Ctrl Pts',(-1.7472034950333,-1.,0.163814161002002));
#22559=CARTESIAN_POINT('Ctrl Pts',(-1.75666056638427,-1.,0.164834765707158));
#22560=CARTESIAN_POINT('Ctrl Pts',(-1.77018771684844,-1.,0.1662793551464));
#22561=CARTESIAN_POINT('Ctrl Pts',(-1.7869064998507,-1.,0.168032772805197));
#22562=CARTESIAN_POINT('Ctrl Pts',(-1.80561530629706,-1.,0.169936923904608));
#22563=CARTESIAN_POINT('Ctrl Pts',(-1.82215766811545,-1.,0.171554770204119));
#22564=CARTESIAN_POINT('Ctrl Pts',(-1.83658380527692,-1.,0.1728894428919));
#22565=CARTESIAN_POINT('Ctrl Pts',(-1.8489811319852,-1.,0.173946627587731));
#22566=CARTESIAN_POINT('Ctrl Pts',(-1.85948367088837,-1.,0.17473525927603));
#22567=CARTESIAN_POINT('Ctrl Pts',(-1.86828349694799,-1.,0.175268337590758));
#22568=CARTESIAN_POINT('Ctrl Pts',(-1.87563767773588,-1.,0.175563480746485));
#22569=CARTESIAN_POINT('Ctrl Pts',(-1.88188663145367,-1.,0.175644148889698));
#22570=CARTESIAN_POINT('Ctrl Pts',(-1.88742606273259,-1.,0.175538155840648));
#22571=CARTESIAN_POINT('Ctrl Pts',(-1.892646301985,-1.,0.175274276190844));
#22572=CARTESIAN_POINT('Ctrl Pts',(-1.89788101117132,-1.,0.174879405091263));
#22573=CARTESIAN_POINT('Ctrl Pts',(-1.90335253862834,-1.,0.174375518661085));
#22574=CARTESIAN_POINT('Ctrl Pts',(-1.90911693975267,-1.,0.173776635257817));
#22575=CARTESIAN_POINT('Ctrl Pts',(-1.91511429159527,-1.,0.173090695383496));
#22576=CARTESIAN_POINT('Ctrl Pts',(-1.9212233439798,-1.,0.172321621259514));
#22577=CARTESIAN_POINT('Ctrl Pts',(-1.92731093582036,-1.,0.171471191532988));
#22578=CARTESIAN_POINT('Ctrl Pts',(-1.93329183155539,-1.,0.170541253116201));
#22579=CARTESIAN_POINT('Ctrl Pts',(-1.93915639211581,-1.,0.169534904817491));
#22580=CARTESIAN_POINT('Ctrl Pts',(-1.94493757756931,-1.,0.168455741607556));
#22581=CARTESIAN_POINT('Ctrl Pts',(-1.95069027794294,-1.,0.167307501784475));
#22582=CARTESIAN_POINT('Ctrl Pts',(-1.9564675971873,-1.,0.166093592002812));
#22583=CARTESIAN_POINT('Ctrl Pts',(-1.96229379940136,-1.,0.164816568920269));
#22584=CARTESIAN_POINT('Ctrl Pts',(-1.96816512677967,-1.,0.163478185457734));
#22585=CARTESIAN_POINT('Ctrl Pts',(-1.97406280235188,-1.,0.162079693556288));
#22586=CARTESIAN_POINT('Ctrl Pts',(-1.97996195437559,-1.,0.160622060784611));
#22587=CARTESIAN_POINT('Ctrl Pts',(-1.98584238283292,-1.,0.159106226437299));
#22588=CARTESIAN_POINT('Ctrl Pts',(-1.99169810931908,-1.,0.157533331459227));
#22589=CARTESIAN_POINT('Ctrl Pts',(-1.99753284771497,-1.,0.155904629548783));
#22590=CARTESIAN_POINT('Ctrl Pts',(-2.00335565310543,-1.,0.154221403049722));
#22591=CARTESIAN_POINT('Ctrl Pts',(-2.00917680318424,-1.,0.15248488362145));
#22592=CARTESIAN_POINT('Ctrl Pts',(-2.01500291940238,-1.,0.150696157673078));
#22593=CARTESIAN_POINT('Ctrl Pts',(-2.02083464969894,-1.,0.148856124775337));
#22594=CARTESIAN_POINT('Ctrl Pts',(-2.02666926182017,-1.,0.146965557332583));
#22595=CARTESIAN_POINT('Ctrl Pts',(-2.03250223739942,-1.,0.145025140186057));
#22596=CARTESIAN_POINT('Ctrl Pts',(-2.03832911025912,-1.,0.143035515058209));
#22597=CARTESIAN_POINT('Ctrl Pts',(-2.04414757947916,-1.,0.140997332152546));
#22598=CARTESIAN_POINT('Ctrl Pts',(-2.04995762001328,-1.,0.138911255368966));
#22599=CARTESIAN_POINT('Ctrl Pts',(-2.05576044414264,-1.,0.136777941218043));
#22600=CARTESIAN_POINT('Ctrl Pts',(-2.06155781517842,-1.,0.134598026192106));
#22601=CARTESIAN_POINT('Ctrl Pts',(-2.06735123910326,-1.,0.13237211154771));
#22602=CARTESIAN_POINT('Ctrl Pts',(-2.07314114713063,-1.,0.130100748328403));
#22603=CARTESIAN_POINT('Ctrl Pts',(-2.07892715110987,-1.,0.12778444527612));
#22604=CARTESIAN_POINT('Ctrl Pts',(-2.08470840653643,-1.,0.125423679412061));
#22605=CARTESIAN_POINT('Ctrl Pts',(-2.09048392424825,-1.,0.123018905621083));
#22606=CARTESIAN_POINT('Ctrl Pts',(-2.0962529286773,-1.,0.120570567965122));
#22607=CARTESIAN_POINT('Ctrl Pts',(-2.102015121329,-1.,0.118079107988355));
#22608=CARTESIAN_POINT('Ctrl Pts',(-2.10777050261309,-1.,0.115544957687926));
#22609=CARTESIAN_POINT('Ctrl Pts',(-2.11351924490306,-1.,0.112968534419737));
#22610=CARTESIAN_POINT('Ctrl Pts',(-2.11926155590865,-1.,0.110350236135025));
#22611=CARTESIAN_POINT('Ctrl Pts',(-2.12499752307,-1.,0.10769043523109));
#22612=CARTESIAN_POINT('Ctrl Pts',(-2.13072704887293,-1.,0.104989479152739));
#22613=CARTESIAN_POINT('Ctrl Pts',(-2.13644992667165,-1.,0.1022477005561));
#22614=CARTESIAN_POINT('Ctrl Pts',(-2.14216588396025,-1.,0.0994654261990914));
#22615=CARTESIAN_POINT('Ctrl Pts',(-2.14787463531795,-1.,0.0966429852305457));
#22616=CARTESIAN_POINT('Ctrl Pts',(-2.1535759397817,-1.,0.0937807218867642));
#22617=CARTESIAN_POINT('Ctrl Pts',(-2.15926961544516,-1.,0.0908789888107264));
#22618=CARTESIAN_POINT('Ctrl Pts',(-2.16495552645014,-1.,0.0879381291386921));
#22619=CARTESIAN_POINT('Ctrl Pts',(-2.17063357870952,-1.,0.0849584620835371));
#22620=CARTESIAN_POINT('Ctrl Pts',(-2.176303712113,-1.,0.0819402680872764));
#22621=CARTESIAN_POINT('Ctrl Pts',(-2.18196589448887,-1.,0.0788837727685241));
#22622=CARTESIAN_POINT('Ctrl Pts',(-2.1876201139953,-1.,0.0757891465836146));
#22623=CARTESIAN_POINT('Ctrl Pts',(-2.19213712013662,-1.,0.0732830357306724));
#22624=CARTESIAN_POINT('Ctrl Pts',(-2.19552129484002,-1.,0.0713863779526153));
#22625=CARTESIAN_POINT('Ctrl Pts',(-2.19777582085423,-1.,0.0701143536325489));
#22626=CARTESIAN_POINT('Ctrl Pts',(-2.19890268624765,-1.,0.069476445021958));
#22627=CARTESIAN_POINT('',(-2.19890268624765,-1.,-0.0694764450219585));
#22628=CARTESIAN_POINT('',(-2.19890268624765,-1.,0.069476445021958));
#22629=CARTESIAN_POINT('',(-1.74236521665491,-1.,-0.163289472382896));
#22630=CARTESIAN_POINT('Ctrl Pts',(-2.19890268624765,-1.,-0.0694764450219585));
#22631=CARTESIAN_POINT('Ctrl Pts',(-2.19777582085261,-1.,-0.0701143536324927));
#22632=CARTESIAN_POINT('Ctrl Pts',(-2.19552129483562,-1.,-0.0713863779524629));
#22633=CARTESIAN_POINT('Ctrl Pts',(-2.19213712012956,-1.,-0.0732830357304277));
#22634=CARTESIAN_POINT('Ctrl Pts',(-2.1876201139874,-1.,-0.0757891465833413));
#22635=CARTESIAN_POINT('Ctrl Pts',(-2.18196589448304,-1.,-0.0788837727683229));
#22636=CARTESIAN_POINT('Ctrl Pts',(-2.1763037121106,-1.,-0.0819402680871941));
#22637=CARTESIAN_POINT('Ctrl Pts',(-2.17063357871031,-1.,-0.0849584620835644));
#22638=CARTESIAN_POINT('Ctrl Pts',(-2.16495552645275,-1.,-0.0879381291387824));
#22639=CARTESIAN_POINT('Ctrl Pts',(-2.15926961544808,-1.,-0.0908789888108267));
#22640=CARTESIAN_POINT('Ctrl Pts',(-2.15357593978377,-1.,-0.0937807218868346));
#22641=CARTESIAN_POINT('Ctrl Pts',(-2.14787463531864,-1.,-0.096642985230569));
#22642=CARTESIAN_POINT('Ctrl Pts',(-2.14216588395974,-1.,-0.0994654261990744));
#22643=CARTESIAN_POINT('Ctrl Pts',(-2.13644992667052,-1.,-0.102247700556064));
#22644=CARTESIAN_POINT('Ctrl Pts',(-2.1307270488718,-1.,-0.104989479152703));
#22645=CARTESIAN_POINT('Ctrl Pts',(-2.12499752306927,-1.,-0.107690435231068));
#22646=CARTESIAN_POINT('Ctrl Pts',(-2.11926155590849,-1.,-0.11035023613502));
#22647=CARTESIAN_POINT('Ctrl Pts',(-2.11351924490335,-1.,-0.112968534419746));
#22648=CARTESIAN_POINT('Ctrl Pts',(-2.10777050261359,-1.,-0.11554495768794));
#22649=CARTESIAN_POINT('Ctrl Pts',(-2.10201512132945,-1.,-0.118079107988368));
#22650=CARTESIAN_POINT('Ctrl Pts',(-2.09625292867756,-1.,-0.120570567965129));
#22651=CARTESIAN_POINT('Ctrl Pts',(-2.09048392424826,-1.,-0.123018905621083));
#22652=CARTESIAN_POINT('Ctrl Pts',(-2.08470840653628,-1.,-0.125423679412058));
#22653=CARTESIAN_POINT('Ctrl Pts',(-2.07892715110967,-1.,-0.127784445276116));
#22654=CARTESIAN_POINT('Ctrl Pts',(-2.07314114713047,-1.,-0.130100748328401));
#22655=CARTESIAN_POINT('Ctrl Pts',(-2.06735123910319,-1.,-0.13237211154771));
#22656=CARTESIAN_POINT('Ctrl Pts',(-2.06155781517844,-1.,-0.134598026192107));
#22657=CARTESIAN_POINT('Ctrl Pts',(-2.0557604441427,-1.,-0.136777941218044));
#22658=CARTESIAN_POINT('Ctrl Pts',(-2.04995762001333,-1.,-0.138911255368966));
#22659=CARTESIAN_POINT('Ctrl Pts',(-2.04414757947919,-1.,-0.140997332152545));
#22660=CARTESIAN_POINT('Ctrl Pts',(-2.03832911025913,-1.,-0.143035515058208));
#22661=CARTESIAN_POINT('Ctrl Pts',(-2.03250223739941,-1.,-0.145025140186058));
#22662=CARTESIAN_POINT('Ctrl Pts',(-2.02666926182017,-1.,-0.146965557332586));
#22663=CARTESIAN_POINT('Ctrl Pts',(-2.02083464969897,-1.,-0.148856124775343));
#22664=CARTESIAN_POINT('Ctrl Pts',(-2.01500291940243,-1.,-0.150696157673084));
#22665=CARTESIAN_POINT('Ctrl Pts',(-2.00917680318426,-1.,-0.152484883621452));
#22666=CARTESIAN_POINT('Ctrl Pts',(-2.00335565310539,-1.,-0.154221403049719));
#22667=CARTESIAN_POINT('Ctrl Pts',(-1.99753284771487,-1.,-0.155904629548775));
#22668=CARTESIAN_POINT('Ctrl Pts',(-1.99169810931893,-1.,-0.157533331459215));
#22669=CARTESIAN_POINT('Ctrl Pts',(-1.98584238283279,-1.,-0.159106226437289));
#22670=CARTESIAN_POINT('Ctrl Pts',(-1.97996195437557,-1.,-0.16062206078461));
#22671=CARTESIAN_POINT('Ctrl Pts',(-1.97406280235204,-1.,-0.162079693556302));
#22672=CARTESIAN_POINT('Ctrl Pts',(-1.96816512678,-1.,-0.16347818545776));
#22673=CARTESIAN_POINT('Ctrl Pts',(-1.96229379940174,-1.,-0.1648165689203));
#22674=CARTESIAN_POINT('Ctrl Pts',(-1.95646759718755,-1.,-0.166093592002833));
#22675=CARTESIAN_POINT('Ctrl Pts',(-1.95069027794286,-1.,-0.167307501784469));
#22676=CARTESIAN_POINT('Ctrl Pts',(-1.94493757756879,-1.,-0.168455741607516));
#22677=CARTESIAN_POINT('Ctrl Pts',(-1.93915639211497,-1.,-0.169534904817425));
#22678=CARTESIAN_POINT('Ctrl Pts',(-1.93329183155455,-1.,-0.170541253116136));
#22679=CARTESIAN_POINT('Ctrl Pts',(-1.92731093582,-1.,-0.17147119153296));
#22680=CARTESIAN_POINT('Ctrl Pts',(-1.92122334398034,-1.,-0.172321621259557));
#22681=CARTESIAN_POINT('Ctrl Pts',(-1.91511429159681,-1.,-0.173090695383619));
#22682=CARTESIAN_POINT('Ctrl Pts',(-1.90911693975475,-1.,-0.173776635257984));
#22683=CARTESIAN_POINT('Ctrl Pts',(-1.90335253863003,-1.,-0.174375518661222));
#22684=CARTESIAN_POINT('Ctrl Pts',(-1.89788101117148,-1.,-0.174879405091277));
#22685=CARTESIAN_POINT('Ctrl Pts',(-1.89264630198279,-1.,-0.175274276190664));
#22686=CARTESIAN_POINT('Ctrl Pts',(-1.88742606272818,-1.,-0.175538155840286));
#22687=CARTESIAN_POINT('Ctrl Pts',(-1.88188663144846,-1.,-0.175644148889271));
#22688=CARTESIAN_POINT('Ctrl Pts',(-1.87563767773249,-1.,-0.175563480746205));
#22689=CARTESIAN_POINT('Ctrl Pts',(-1.86828349694972,-1.,-0.175268337590901));
#22690=CARTESIAN_POINT('Ctrl Pts',(-1.85948367089838,-1.,-0.174735259276856));
#22691=CARTESIAN_POINT('Ctrl Pts',(-1.84898113200543,-1.,-0.173946627589401));
#22692=CARTESIAN_POINT('Ctrl Pts',(-1.83658380530747,-1.,-0.17288944289442));
#22693=CARTESIAN_POINT('Ctrl Pts',(-1.82215766815414,-1.,-0.171554770207306));
#22694=CARTESIAN_POINT('Ctrl Pts',(-1.80561530633924,-1.,-0.169936923908078));
#22695=CARTESIAN_POINT('Ctrl Pts',(-1.78690649988931,-1.,-0.16803277280837));
#22696=CARTESIAN_POINT('Ctrl Pts',(-1.77018771687692,-1.,-0.166279355148738));
#22697=CARTESIAN_POINT('Ctrl Pts',(-1.75666056640041,-1.,-0.164834765708484));
#22698=CARTESIAN_POINT('Ctrl Pts',(-1.74720349503904,-1.,-0.163814161002474));
#22699=CARTESIAN_POINT('Ctrl Pts',(-1.74236521665491,-1.,-0.163289472382896));
#22700=CARTESIAN_POINT('',(-1.7075470150345,-1.,-0.383122945602004));
#22701=CARTESIAN_POINT('Origin',(0.,-1.,0.));
#22702=CARTESIAN_POINT('',(-2.11275013067528,-1.,-0.61342227326009));
#22703=CARTESIAN_POINT('Ctrl Pts',(-1.7075470150345,-1.,-0.383122945602004));
#22704=CARTESIAN_POINT('Ctrl Pts',(-1.71231062891398,-1.,-0.384119047314215));
#22705=CARTESIAN_POINT('Ctrl Pts',(-1.72162022244582,-1.,-0.386070790323281));
#22706=CARTESIAN_POINT('Ctrl Pts',(-1.73493170972829,-1.,-0.388877023502615));
#22707=CARTESIAN_POINT('Ctrl Pts',(-1.75137405310193,-1.,-0.392375812285395));
#22708=CARTESIAN_POINT('Ctrl Pts',(-1.76975560043442,-1.,-0.396346196110688));
#22709=CARTESIAN_POINT('Ctrl Pts',(-1.78598826343754,-1.,-0.399919403774155));
#22710=CARTESIAN_POINT('Ctrl Pts',(-1.80012077173238,-1.,-0.403107976163396));
#22711=CARTESIAN_POINT('Ctrl Pts',(-1.81223801812013,-1.,-0.405933518407175));
#22712=CARTESIAN_POINT('Ctrl Pts',(-1.82247022677562,-1.,-0.408428948106227));
#22713=CARTESIAN_POINT('Ctrl Pts',(-1.83100408895047,-1.,-0.410641256301276));
#22714=CARTESIAN_POINT('Ctrl Pts',(-1.8380895347617,-1.,-0.412633125322945));
#22715=CARTESIAN_POINT('Ctrl Pts',(-1.84405757074218,-1.,-0.414487438255542));
#22716=CARTESIAN_POINT('Ctrl Pts',(-1.84929312930314,-1.,-0.416300022039885));
#22717=CARTESIAN_POINT('Ctrl Pts',(-1.8541763285645,-1.,-0.418164129144045));
#22718=CARTESIAN_POINT('Ctrl Pts',(-1.8590328109667,-1.,-0.420157287975583));
#22719=CARTESIAN_POINT('Ctrl Pts',(-1.86408083333863,-1.,-0.422327307417884));
#22720=CARTESIAN_POINT('Ctrl Pts',(-1.8693780394412,-1.,-0.424678177290876));
#22721=CARTESIAN_POINT('Ctrl Pts',(-1.87486989291333,-1.,-0.427183828518743));
#22722=CARTESIAN_POINT('Ctrl Pts',(-1.88044229001778,-1.,-0.429803062482217));
#22723=CARTESIAN_POINT('Ctrl Pts',(-1.88596913666828,-1.,-0.432493038548833));
#22724=CARTESIAN_POINT('Ctrl Pts',(-1.89136993975585,-1.,-0.43522566096358));
#22725=CARTESIAN_POINT('Ctrl Pts',(-1.89663648956549,-1.,-0.437995003948443));
#22726=CARTESIAN_POINT('Ctrl Pts',(-1.90180124389137,-1.,-0.44080783370416));
#22727=CARTESIAN_POINT('Ctrl Pts',(-1.90691756144906,-1.,-0.44367755684917));
#22728=CARTESIAN_POINT('Ctrl Pts',(-1.91203699981095,-1.,-0.446617343485651));
#22729=CARTESIAN_POINT('Ctrl Pts',(-1.91718342555717,-1.,-0.449632260106572));
#22730=CARTESIAN_POINT('Ctrl Pts',(-1.9223538064847,-1.,-0.452719478359356));
#22731=CARTESIAN_POINT('Ctrl Pts',(-1.92753067150461,-1.,-0.455872005174335));
#22732=CARTESIAN_POINT('Ctrl Pts',(-1.93269066517936,-1.,-0.459081234547931));
#22733=CARTESIAN_POINT('Ctrl Pts',(-1.93781486640834,-1.,-0.462340031009087));
#22734=CARTESIAN_POINT('Ctrl Pts',(-1.94289794196205,-1.,-0.465645462026064));
#22735=CARTESIAN_POINT('Ctrl Pts',(-1.94794381136524,-1.,-0.468997482913158));
#22736=CARTESIAN_POINT('Ctrl Pts',(-1.95296148278136,-1.,-0.472397672264079));
#22737=CARTESIAN_POINT('Ctrl Pts',(-1.95796111148175,-1.,-0.475848034683171));
#22738=CARTESIAN_POINT('Ctrl Pts',(-1.96294933055938,-1.,-0.479349583074846));
#22739=CARTESIAN_POINT('Ctrl Pts',(-1.96792703422358,-1.,-0.482901662120686));
#22740=CARTESIAN_POINT('Ctrl Pts',(-1.97289186263272,-1.,-0.486502692907661));
#22741=CARTESIAN_POINT('Ctrl Pts',(-1.97783973019229,-1.,-0.490150627860955));
#22742=CARTESIAN_POINT('Ctrl Pts',(-1.9827665876182,-1.,-0.493843476541492));
#22743=CARTESIAN_POINT('Ctrl Pts',(-1.98767044752929,-1.,-0.497579909545564));
#22744=CARTESIAN_POINT('Ctrl Pts',(-1.9925514912615,-1.,-0.501359287727129));
#22745=CARTESIAN_POINT('Ctrl Pts',(-1.99741107463567,-1.,-0.505181361323011));
#22746=CARTESIAN_POINT('Ctrl Pts',(-2.00225107134733,-1.,-0.509046069886152));
#22747=CARTESIAN_POINT('Ctrl Pts',(-2.00707309946955,-1.,-0.512953306961813));
#22748=CARTESIAN_POINT('Ctrl Pts',(-2.01187773939257,-1.,-0.516902681728733));
#22749=CARTESIAN_POINT('Ctrl Pts',(-2.01666477917305,-1.,-0.520893590399428));
#22750=CARTESIAN_POINT('Ctrl Pts',(-2.02143356304712,-1.,-0.524925318333518));
#22751=CARTESIAN_POINT('Ctrl Pts',(-2.02618329083289,-1.,-0.52899712724191));
#22752=CARTESIAN_POINT('Ctrl Pts',(-2.03091336214401,-1.,-0.533108355132905));
#22753=CARTESIAN_POINT('Ctrl Pts',(-2.03562362953993,-1.,-0.537258489833134));
#22754=CARTESIAN_POINT('Ctrl Pts',(-2.0403142269048,-1.,-0.54144712061552));
#22755=CARTESIAN_POINT('Ctrl Pts',(-2.0449854471456,-1.,-0.545673903817348));
#22756=CARTESIAN_POINT('Ctrl Pts',(-2.04963761077974,-1.,-0.549938525150342));
#22757=CARTESIAN_POINT('Ctrl Pts',(-2.05427091604482,-1.,-0.554240657464109));
#22758=CARTESIAN_POINT('Ctrl Pts',(-2.05888537756571,-1.,-0.558579940185467));
#22759=CARTESIAN_POINT('Ctrl Pts',(-2.06348090160697,-1.,-0.562955993082574));
#22760=CARTESIAN_POINT('Ctrl Pts',(-2.06805732997383,-1.,-0.567368421181229));
#22761=CARTESIAN_POINT('Ctrl Pts',(-2.07261449292757,-1.,-0.571816823242411));
#22762=CARTESIAN_POINT('Ctrl Pts',(-2.07715226767361,-1.,-0.576300797416274));
#22763=CARTESIAN_POINT('Ctrl Pts',(-2.08167059018138,-1.,-0.580819952107257));
#22764=CARTESIAN_POINT('Ctrl Pts',(-2.086169437277,-1.,-0.585373918990895));
#22765=CARTESIAN_POINT('Ctrl Pts',(-2.09064881812053,-1.,-0.589962365403189));
#22766=CARTESIAN_POINT('Ctrl Pts',(-2.09510876220501,-1.,-0.594585006052823));
#22767=CARTESIAN_POINT('Ctrl Pts',(-2.09954930865331,-1.,-0.599241616422144));
#22768=CARTESIAN_POINT('Ctrl Pts',(-2.10397049887709,-1.,-0.603932030738212));
#22769=CARTESIAN_POINT('Ctrl Pts',(-2.10749199615859,-1.,-0.607711315456826));
#22770=CARTESIAN_POINT('Ctrl Pts',(-2.11012443807661,-1.,-0.610560911691113));
#22771=CARTESIAN_POINT('Ctrl Pts',(-2.11187554260142,-1.,-0.61246736556225));
#22772=CARTESIAN_POINT('Ctrl Pts',(-2.11275013067528,-1.,-0.61342227326009));
#22773=CARTESIAN_POINT('',(-2.0698113262342,-1.,-0.745574324794401));
#22774=CARTESIAN_POINT('',(-2.11275013067528,-1.,-0.61342227326009));
#22775=CARTESIAN_POINT('',(-1.60662857109684,-1.,-0.693717979106306));
#22776=CARTESIAN_POINT('Ctrl Pts',(-2.0698113262342,-1.,-0.745574324794401));
#22777=CARTESIAN_POINT('Ctrl Pts',(-2.06854248895575,-1.,-0.74583279137781));
#22778=CARTESIAN_POINT('Ctrl Pts',(-2.06600523016401,-1.,-0.746345871542695));
#22779=CARTESIAN_POINT('Ctrl Pts',(-2.06220058927162,-1.,-0.747103932785504));
#22780=CARTESIAN_POINT('Ctrl Pts',(-2.05713023030263,-1.,-0.748091554181101));
#22781=CARTESIAN_POINT('Ctrl Pts',(-2.05079645591606,-1.,-0.749287468663053));
#22782=CARTESIAN_POINT('Ctrl Pts',(-2.04446689147754,-1.,-0.750444657874758));
#22783=CARTESIAN_POINT('Ctrl Pts',(-2.03814160092173,-1.,-0.751562963361383));
#22784=CARTESIAN_POINT('Ctrl Pts',(-2.03182068456467,-1.,-0.752642180488104));
#22785=CARTESIAN_POINT('Ctrl Pts',(-2.02550428623587,-1.,-0.753682061113765));
#22786=CARTESIAN_POINT('Ctrl Pts',(-2.01919259406003,-1.,-0.75468233072352));
#22787=CARTESIAN_POINT('Ctrl Pts',(-2.01288584328149,-1.,-0.7556427049581));
#22788=CARTESIAN_POINT('Ctrl Pts',(-2.00658431587682,-1.,-0.756562904646496));
#22789=CARTESIAN_POINT('Ctrl Pts',(-2.00028834739072,-1.,-0.757442676862341));
#22790=CARTESIAN_POINT('Ctrl Pts',(-1.9939983109871,-1.,-0.758281796766377));
#22791=CARTESIAN_POINT('Ctrl Pts',(-1.98771456680806,-1.,-0.759080037802242));
#22792=CARTESIAN_POINT('Ctrl Pts',(-1.98143741418156,-1.,-0.759837147452135));
#22793=CARTESIAN_POINT('Ctrl Pts',(-1.97516705321521,-1.,-0.760552825409855));
#22794=CARTESIAN_POINT('Ctrl Pts',(-1.96890351582545,-1.,-0.761226690483986));
#22795=CARTESIAN_POINT('Ctrl Pts',(-1.96264672744229,-1.,-0.761858300014575));
#22796=CARTESIAN_POINT('Ctrl Pts',(-1.95639665309893,-1.,-0.762447203806263));
#22797=CARTESIAN_POINT('Ctrl Pts',(-1.95015342590025,-1.,-0.762992990878774));
#22798=CARTESIAN_POINT('Ctrl Pts',(-1.94391746617626,-1.,-0.76349533353858));
#22799=CARTESIAN_POINT('Ctrl Pts',(-1.93768964875867,-1.,-0.763954049121393));
#22800=CARTESIAN_POINT('Ctrl Pts',(-1.93147105496367,-1.,-0.764369010673889));
#22801=CARTESIAN_POINT('Ctrl Pts',(-1.92526263537041,-1.,-0.764740025488189));
#22802=CARTESIAN_POINT('Ctrl Pts',(-1.91906491634197,-1.,-0.765066729667095));
#22803=CARTESIAN_POINT('Ctrl Pts',(-1.91287765805174,-1.,-0.765348465884739));
#22804=CARTESIAN_POINT('Ctrl Pts',(-1.90669961402362,-1.,-0.765584196937936));
#22805=CARTESIAN_POINT('Ctrl Pts',(-1.90052930393599,-1.,-0.765772772593395));
#22806=CARTESIAN_POINT('Ctrl Pts',(-1.89436577771389,-1.,-0.765913193856979));
#22807=CARTESIAN_POINT('Ctrl Pts',(-1.88820926433409,-1.,-0.76600483706209));
#22808=CARTESIAN_POINT('Ctrl Pts',(-1.88206215302561,-1.,-0.766047794851868));
#22809=CARTESIAN_POINT('Ctrl Pts',(-1.87592888967886,-1.,-0.766042837036759));
#22810=CARTESIAN_POINT('Ctrl Pts',(-1.86981398314345,-1.,-0.765990708546111));
#22811=CARTESIAN_POINT('Ctrl Pts',(-1.86372027063314,-1.,-0.765891519092557));
#22812=CARTESIAN_POINT('Ctrl Pts',(-1.85764741390391,-1.,-0.765744212909305));
#22813=CARTESIAN_POINT('Ctrl Pts',(-1.85158945130054,-1.,-0.765545710619023));
#22814=CARTESIAN_POINT('Ctrl Pts',(-1.8455369887591,-1.,-0.765291664861971));
#22815=CARTESIAN_POINT('Ctrl Pts',(-1.83948181064823,-1.,-0.764978057881687));
#22816=CARTESIAN_POINT('Ctrl Pts',(-1.8334207722714,-1.,-0.764602549687845));
#22817=CARTESIAN_POINT('Ctrl Pts',(-1.8273599120008,-1.,-0.764165902606055));
#22818=CARTESIAN_POINT('Ctrl Pts',(-1.82131873145297,-1.,-0.763673465462854));
#22819=CARTESIAN_POINT('Ctrl Pts',(-1.81532118405566,-1.,-0.763132003836783));
#22820=CARTESIAN_POINT('Ctrl Pts',(-1.80938551463989,-1.,-0.762546129464036));
#22821=CARTESIAN_POINT('Ctrl Pts',(-1.80351583877334,-1.,-0.761915336443515));
#22822=CARTESIAN_POINT('Ctrl Pts',(-1.79768986997735,-1.,-0.761229695230359));
#22823=CARTESIAN_POINT('Ctrl Pts',(-1.79185815610802,-1.,-0.760469555880425));
#22824=CARTESIAN_POINT('Ctrl Pts',(-1.78596964884526,-1.,-0.759614401109868));
#22825=CARTESIAN_POINT('Ctrl Pts',(-1.77999411220912,-1.,-0.75865062667738));
#22826=CARTESIAN_POINT('Ctrl Pts',(-1.77394167108342,-1.,-0.757578264077238));
#22827=CARTESIAN_POINT('Ctrl Pts',(-1.76789396003141,-1.,-0.756421896028403));
#22828=CARTESIAN_POINT('Ctrl Pts',(-1.7619781724032,-1.,-0.755220979975262));
#22829=CARTESIAN_POINT('Ctrl Pts',(-1.75631083600175,-1.,-0.75400925402848));
#22830=CARTESIAN_POINT('Ctrl Pts',(-1.75095139468809,-1.,-0.752797683531377));
#22831=CARTESIAN_POINT('Ctrl Pts',(-1.74585086852298,-1.,-0.751555614163629));
#22832=CARTESIAN_POINT('Ctrl Pts',(-1.74080458266705,-1.,-0.75019343597954));
#22833=CARTESIAN_POINT('Ctrl Pts',(-1.73550351679848,-1.,-0.748582462954854));
#22834=CARTESIAN_POINT('Ctrl Pts',(-1.72958533647399,-1.,-0.746574710096436));
#22835=CARTESIAN_POINT('Ctrl Pts',(-1.7226822991693,-1.,-0.744021445433764));
#22836=CARTESIAN_POINT('Ctrl Pts',(-1.71447789751927,-1.,-0.740795162032087));
#22837=CARTESIAN_POINT('Ctrl Pts',(-1.70473309006121,-1.,-0.736799665724771));
#22838=CARTESIAN_POINT('Ctrl Pts',(-1.69326921975743,-1.,-0.731963238697195));
#22839=CARTESIAN_POINT('Ctrl Pts',(-1.67996158455503,-1.,-0.726235967997433));
#22840=CARTESIAN_POINT('Ctrl Pts',(-1.6647288055568,-1.,-0.719585433804282));
#22841=CARTESIAN_POINT('Ctrl Pts',(-1.64752408832016,-1.,-0.711993139355394));
#22842=CARTESIAN_POINT('Ctrl Pts',(-1.63216541664676,-1.,-0.705159151988319));
#22843=CARTESIAN_POINT('Ctrl Pts',(-1.61974673472612,-1.,-0.699605146405088));
#22844=CARTESIAN_POINT('Ctrl Pts',(-1.61106790958151,-1.,-0.695712097881194));
#22845=CARTESIAN_POINT('Ctrl Pts',(-1.60662857109684,-1.,-0.693717979106306));
#22846=CARTESIAN_POINT('',(-1.5055822144029,-1.,-0.892032620296855));
#22847=CARTESIAN_POINT('Origin',(0.,-1.,0.));
#22848=CARTESIAN_POINT('',(-1.81978687191668,-1.,-1.23627494547115));
#22849=CARTESIAN_POINT('Ctrl Pts',(-1.5055822144029,-1.,-0.892032620296855));
#22850=CARTESIAN_POINT('Ctrl Pts',(-1.50980486806688,-1.,-0.894452006964543));
#22851=CARTESIAN_POINT('Ctrl Pts',(-1.51805569590094,-1.,-0.899185047483511));
#22852=CARTESIAN_POINT('Ctrl Pts',(-1.52984849887993,-1.,-0.905967409625651));
#22853=CARTESIAN_POINT('Ctrl Pts',(-1.54440491149498,-1.,-0.914375919026456));
#22854=CARTESIAN_POINT('Ctrl Pts',(-1.56065988578893,-1.,-0.923832188944341));
#22855=CARTESIAN_POINT('Ctrl Pts',(-1.57499388382243,-1.,-0.932246680108685));
#22856=CARTESIAN_POINT('Ctrl Pts',(-1.58744937487176,-1.,-0.939646377893399));
#22857=CARTESIAN_POINT('Ctrl Pts',(-1.59810042043673,-1.,-0.946078063315257));
#22858=CARTESIAN_POINT('Ctrl Pts',(-1.60706069896936,-1.,-0.951613284356035));
#22859=CARTESIAN_POINT('Ctrl Pts',(-1.61449324337085,-1.,-0.956354422920671));
#22860=CARTESIAN_POINT('Ctrl Pts',(-1.62061638140221,-1.,-0.960438326101729));
#22861=CARTESIAN_POINT('Ctrl Pts',(-1.62571930670187,-1.,-0.964046107040536));
#22862=CARTESIAN_POINT('Ctrl Pts',(-1.63013849959461,-1.,-0.967387853230345));
#22863=CARTESIAN_POINT('Ctrl Pts',(-1.63420665729798,-1.,-0.970669715997509));
#22864=CARTESIAN_POINT('Ctrl Pts',(-1.63820952658144,-1.,-0.974066058287418));
#22865=CARTESIAN_POINT('Ctrl Pts',(-1.64233990826687,-1.,-0.977689794119416));
#22866=CARTESIAN_POINT('Ctrl Pts',(-1.64665139190656,-1.,-0.981562530939489));
#22867=CARTESIAN_POINT('Ctrl Pts',(-1.65110016612638,-1.,-0.985642622920821));
#22868=CARTESIAN_POINT('Ctrl Pts',(-1.65559044289699,-1.,-0.989855627854165));
#22869=CARTESIAN_POINT('Ctrl Pts',(-1.66001553809947,-1.,-0.994121836661306));
#22870=CARTESIAN_POINT('Ctrl Pts',(-1.66430758030376,-1.,-0.998389654952758));
#22871=CARTESIAN_POINT('Ctrl Pts',(-1.66846059277303,-1.,-1.00265091003727));
#22872=CARTESIAN_POINT('Ctrl Pts',(-1.67250335383293,-1.,-1.00692206696414));
#22873=CARTESIAN_POINT('Ctrl Pts',(-1.67648246776464,-1.,-1.01123236493511));
#22874=CARTESIAN_POINT('Ctrl Pts',(-1.68044289894798,-1.,-1.01561026162773));
#22875=CARTESIAN_POINT('Ctrl Pts',(-1.68440578021706,-1.,-1.02006795074201));
#22876=CARTESIAN_POINT('Ctrl Pts',(-1.68836910178447,-1.,-1.02460180535255));
#22877=CARTESIAN_POINT('Ctrl Pts',(-1.69231840863458,-1.,-1.02919977579147));
#22878=CARTESIAN_POINT('Ctrl Pts',(-1.69623414782771,-1.,-1.03384646003588));
#22879=CARTESIAN_POINT('Ctrl Pts',(-1.70010052930962,-1.,-1.03852922490789));
#22880=CARTESIAN_POINT('Ctrl Pts',(-1.70391338707982,-1.,-1.04324363334554));
#22881=CARTESIAN_POINT('Ctrl Pts',(-1.70767646263649,-1.,-1.04799085404995));
#22882=CARTESIAN_POINT('Ctrl Pts',(-1.71139783543989,-1.,-1.05277517202855));
#22883=CARTESIAN_POINT('Ctrl Pts',(-1.7150865442702,-1.,-1.05760163192479));
#22884=CARTESIAN_POINT('Ctrl Pts',(-1.71874858456904,-1.,-1.06247324680647));
#22885=CARTESIAN_POINT('Ctrl Pts',(-1.72238500928453,-1.,-1.06738966975462));
#22886=CARTESIAN_POINT('Ctrl Pts',(-1.72599406198488,-1.,-1.07234866990252));
#22887=CARTESIAN_POINT('Ctrl Pts',(-1.72957248977424,-1.,-1.0773470373727));
#22888=CARTESIAN_POINT('Ctrl Pts',(-1.73311705663407,-1.,-1.08238162784749));
#22889=CARTESIAN_POINT('Ctrl Pts',(-1.73662628326091,-1.,-1.08745056285427));
#22890=CARTESIAN_POINT('Ctrl Pts',(-1.74010053962247,-1.,-1.09255329056493));
#22891=CARTESIAN_POINT('Ctrl Pts',(-1.74354119236208,-1.,-1.09768999241225));
#22892=CARTESIAN_POINT('Ctrl Pts',(-1.74695004214923,-1.,-1.10286118991143));
#22893=CARTESIAN_POINT('Ctrl Pts',(-1.7503286607592,-1.,-1.10806728183007));
#22894=CARTESIAN_POINT('Ctrl Pts',(-1.7536777209463,-1.,-1.11330807582551));
#22895=CARTESIAN_POINT('Ctrl Pts',(-1.75699720772105,-1.,-1.11858293216763));
#22896=CARTESIAN_POINT('Ctrl Pts',(-1.76028671825096,-1.,-1.12389096855086));
#22897=CARTESIAN_POINT('Ctrl Pts',(-1.7635457196617,-1.,-1.12923123555075));
#22898=CARTESIAN_POINT('Ctrl Pts',(-1.76677384551862,-1.,-1.1346029180462));
#22899=CARTESIAN_POINT('Ctrl Pts',(-1.76997111386769,-1.,-1.14000548336975));
#22900=CARTESIAN_POINT('Ctrl Pts',(-1.77313777896194,-1.,-1.1454385822692));
#22901=CARTESIAN_POINT('Ctrl Pts',(-1.7762742255701,-1.,-1.15090197841515));
#22902=CARTESIAN_POINT('Ctrl Pts',(-1.77938085564275,-1.,-1.15639547194698));
#22903=CARTESIAN_POINT('Ctrl Pts',(-1.78245795881009,-1.,-1.16191881298499));
#22904=CARTESIAN_POINT('Ctrl Pts',(-1.78550566040443,-1.,-1.16747166312303));
#22905=CARTESIAN_POINT('Ctrl Pts',(-1.78852398877616,-1.,-1.17305363177328));
#22906=CARTESIAN_POINT('Ctrl Pts',(-1.79151291552689,-1.,-1.17866429440809));
#22907=CARTESIAN_POINT('Ctrl Pts',(-1.79447240321515,-1.,-1.18430321697432));
#22908=CARTESIAN_POINT('Ctrl Pts',(-1.79740245923478,-1.,-1.18996997934445));
#22909=CARTESIAN_POINT('Ctrl Pts',(-1.80030314369879,-1.,-1.19566418930242));
#22910=CARTESIAN_POINT('Ctrl Pts',(-1.80317454838603,-1.,-1.20138548938974));
#22911=CARTESIAN_POINT('Ctrl Pts',(-1.80601678480707,-1.,-1.20713356605475));
#22912=CARTESIAN_POINT('Ctrl Pts',(-1.80882996917129,-1.,-1.21290815708314));
#22913=CARTESIAN_POINT('Ctrl Pts',(-1.81161420806656,-1.,-1.21870906103557));
#22914=CARTESIAN_POINT('Ctrl Pts',(-1.81436959210434,-1.,-1.2245361330495));
#22915=CARTESIAN_POINT('Ctrl Pts',(-1.8165508718364,-1.,-1.2292186489137));
#22916=CARTESIAN_POINT('Ctrl Pts',(-1.81817389921279,-1.,-1.2327422452705));
#22917=CARTESIAN_POINT('Ctrl Pts',(-1.81925017193666,-1.,-1.23509651170476));
#22918=CARTESIAN_POINT('Ctrl Pts',(-1.81978687191668,-1.,-1.23627494547115));
#22919=CARTESIAN_POINT('',(-1.73811241238545,-1.,-1.34869019493419));
#22920=CARTESIAN_POINT('',(-1.81978687191668,-1.,-1.23627494547115));
#22921=CARTESIAN_POINT('',(-1.31362392696032,-1.,-1.15624053661742));
#22922=CARTESIAN_POINT('Ctrl Pts',(-1.73811241238545,-1.,-1.34869019493419));
#22923=CARTESIAN_POINT('Ctrl Pts',(-1.73682580585691,-1.,-1.34854391898045));
#22924=CARTESIAN_POINT('Ctrl Pts',(-1.73425417885907,-1.,-1.34824783112887));
#22925=CARTESIAN_POINT('Ctrl Pts',(-1.7304014965394,-1.,-1.34779309152035));
#22926=CARTESIAN_POINT('Ctrl Pts',(-1.72527410680674,-1.,-1.34716554819527));
#22927=CARTESIAN_POINT('Ctrl Pts',(-1.7188807715049,-1.,-1.34634568653227));
#22928=CARTESIAN_POINT('Ctrl Pts',(-1.71250340686822,-1.,-1.34549029589416));
#22929=CARTESIAN_POINT('Ctrl Pts',(-1.70614212266738,-1.,-1.34459924533831));
#22930=CARTESIAN_POINT('Ctrl Pts',(-1.69979707754427,-1.,-1.34367237124483));
#22931=CARTESIAN_POINT('Ctrl Pts',(-1.6934684849687,-1.,-1.34270948206319));
#22932=CARTESIAN_POINT('Ctrl Pts',(-1.68715660868764,-1.,-1.341710374848));
#22933=CARTESIAN_POINT('Ctrl Pts',(-1.68086176030362,-1.,-1.34067485185203));
#22934=CARTESIAN_POINT('Ctrl Pts',(-1.67458429426086,-1.,-1.3396027347034));
#22935=CARTESIAN_POINT('Ctrl Pts',(-1.66832460783989,-1.,-1.33849388654388));
#22936=CARTESIAN_POINT('Ctrl Pts',(-1.66208312541983,-1.,-1.33734820885262));
#22937=CARTESIAN_POINT('Ctrl Pts',(-1.65586025952593,-1.,-1.33616559745172));
#22938=CARTESIAN_POINT('Ctrl Pts',(-1.6496563728683,-1.,-1.33494590467993));
#22939=CARTESIAN_POINT('Ctrl Pts',(-1.6434717485603,-1.,-1.33368890676572));
#22940=CARTESIAN_POINT('Ctrl Pts',(-1.63730653475089,-1.,-1.33239425103724));
#22941=CARTESIAN_POINT('Ctrl Pts',(-1.63116079730923,-1.,-1.33106149345645));
#22942=CARTESIAN_POINT('Ctrl Pts',(-1.62503464209797,-1.,-1.3296901950568));
#22943=CARTESIAN_POINT('Ctrl Pts',(-1.61892832270724,-1.,-1.32828000610449));
#22944=CARTESIAN_POINT('Ctrl Pts',(-1.6128423401575,-1.,-1.32683074483356));
#22945=CARTESIAN_POINT('Ctrl Pts',(-1.60677758290954,-1.,-1.32534250785782));
#22946=CARTESIAN_POINT('Ctrl Pts',(-1.60073511858687,-1.,-1.32381550858256));
#22947=CARTESIAN_POINT('Ctrl Pts',(-1.59471591079403,-1.,-1.32224985747682));
#22948=CARTESIAN_POINT('Ctrl Pts',(-1.58872057258245,-1.,-1.32064537110892));
#22949=CARTESIAN_POINT('Ctrl Pts',(-1.58274907898834,-1.,-1.31900135021432));
#22950=CARTESIAN_POINT('Ctrl Pts',(-1.5768005650559,-1.,-1.31731642317187));
#22951=CARTESIAN_POINT('Ctrl Pts',(-1.57087397835723,-1.,-1.31558903860016));
#22952=CARTESIAN_POINT('Ctrl Pts',(-1.56496872402353,-1.,-1.31381795281002));
#22953=CARTESIAN_POINT('Ctrl Pts',(-1.55908521254821,-1.,-1.31200264341696));
#22954=CARTESIAN_POINT('Ctrl Pts',(-1.55322568759481,-1.,-1.31014393684222));
#22955=CARTESIAN_POINT('Ctrl Pts',(-1.54739413957185,-1.,-1.30824393907473));
#22956=CARTESIAN_POINT('Ctrl Pts',(-1.54159462645432,-1.,-1.30630475189556));
#22957=CARTESIAN_POINT('Ctrl Pts',(-1.53582981268977,-1.,-1.30432735639489));
#22958=CARTESIAN_POINT('Ctrl Pts',(-1.53009970283891,-1.,-1.30231064395568));
#22959=CARTESIAN_POINT('Ctrl Pts',(-1.52439957861062,-1.,-1.30024984366328));
#22960=CARTESIAN_POINT('Ctrl Pts',(-1.51872184912724,-1.,-1.29813791800747));
#22961=CARTESIAN_POINT('Ctrl Pts',(-1.51305994241402,-1.,-1.29596850710509));
#22962=CARTESIAN_POINT('Ctrl Pts',(-1.50741159078365,-1.,-1.29373841372842));
#22963=CARTESIAN_POINT('Ctrl Pts',(-1.50178230149776,-1.,-1.29145022885181));
#22964=CARTESIAN_POINT('Ctrl Pts',(-1.49618896881754,-1.,-1.28911506584254));
#22965=CARTESIAN_POINT('Ctrl Pts',(-1.4906522831278,-1.,-1.2867467611644));
#22966=CARTESIAN_POINT('Ctrl Pts',(-1.4851881711891,-1.,-1.28435533880201));
#22967=CARTESIAN_POINT('Ctrl Pts',(-1.47980070347095,-1.,-1.28194158939517));
#22968=CARTESIAN_POINT('Ctrl Pts',(-1.4744717526707,-1.,-1.2794891824849));
#22969=CARTESIAN_POINT('Ctrl Pts',(-1.46916035917133,-1.,-1.27696414831089));
#22970=CARTESIAN_POINT('Ctrl Pts',(-1.46382431332476,-1.,-1.27433119897822));
#22971=CARTESIAN_POINT('Ctrl Pts',(-1.45843906294697,-1.,-1.27156805265289));
#22972=CARTESIAN_POINT('Ctrl Pts',(-1.45301422764247,-1.,-1.2686778680489));
#22973=CARTESIAN_POINT('Ctrl Pts',(-1.44761985001662,-1.,-1.26570925118868));
#22974=CARTESIAN_POINT('Ctrl Pts',(-1.44236470511303,-1.,-1.26273903323859));
#22975=CARTESIAN_POINT('Ctrl Pts',(-1.43734919180848,-1.,-1.25983531012005));
#22976=CARTESIAN_POINT('Ctrl Pts',(-1.43262645609691,-1.,-1.25702687965755));
#22977=CARTESIAN_POINT('Ctrl Pts',(-1.42815938799387,-1.,-1.25426945222639));
#22978=CARTESIAN_POINT('Ctrl Pts',(-1.42378102115575,-1.,-1.2514145557001));
#22979=CARTESIAN_POINT('Ctrl Pts',(-1.41923722596025,-1.,-1.24824430986571));
#22980=CARTESIAN_POINT('Ctrl Pts',(-1.41422913175179,-1.,-1.24450600513056));
#22981=CARTESIAN_POINT('Ctrl Pts',(-1.40845295531283,-1.,-1.23994455029534));
#22982=CARTESIAN_POINT('Ctrl Pts',(-1.40164708206106,-1.,-1.23434087290423));
#22983=CARTESIAN_POINT('Ctrl Pts',(-1.39361389568796,-1.,-1.22752961899387));
#22984=CARTESIAN_POINT('Ctrl Pts',(-1.38420564527715,-1.,-1.21938737280852));
#22985=CARTESIAN_POINT('Ctrl Pts',(-1.37331915607905,-1.,-1.20982812925645));
#22986=CARTESIAN_POINT('Ctrl Pts',(-1.36088705043885,-1.,-1.1987959077932));
#22987=CARTESIAN_POINT('Ctrl Pts',(-1.34687054001093,-1.,-1.18625865667441));
#22988=CARTESIAN_POINT('Ctrl Pts',(-1.33437539347008,-1.,-1.17501305789857));
#22989=CARTESIAN_POINT('Ctrl Pts',(-1.32428080721772,-1.,-1.16589330093588));
#22990=CARTESIAN_POINT('Ctrl Pts',(-1.31722977216397,-1.,-1.15950888730809));
#22991=CARTESIAN_POINT('Ctrl Pts',(-1.31362392696032,-1.,-1.15624053661742));
#22992=CARTESIAN_POINT('',(-1.15624053661742,-1.,-1.31362392696033));
#22993=CARTESIAN_POINT('Origin',(0.,-1.,0.));
#22994=CARTESIAN_POINT('',(-1.34869019493419,-1.,-1.73811241238545));
#22995=CARTESIAN_POINT('Ctrl Pts',(-1.15624053661742,-1.,-1.31362392696033));
#22996=CARTESIAN_POINT('Ctrl Pts',(-1.15950888730433,-1.,-1.3172297721596));
#22997=CARTESIAN_POINT('Ctrl Pts',(-1.16589330092532,-1.,-1.32428080720544));
#22998=CARTESIAN_POINT('Ctrl Pts',(-1.17501305787994,-1.,-1.33437539344842));
#22999=CARTESIAN_POINT('Ctrl Pts',(-1.18625865664915,-1.,-1.34687053998157));
#23000=CARTESIAN_POINT('Ctrl Pts',(-1.1987959077656,-1.,-1.36088705040677));
#23001=CARTESIAN_POINT('Ctrl Pts',(-1.20982812923113,-1.,-1.37331915604962));
#23002=CARTESIAN_POINT('Ctrl Pts',(-1.21938737278853,-1.,-1.38420564525391));
#23003=CARTESIAN_POINT('Ctrl Pts',(-1.22752961898063,-1.,-1.39361389567257));
#23004=CARTESIAN_POINT('Ctrl Pts',(-1.23434087289768,-1.,-1.40164708205345));
#23005=CARTESIAN_POINT('Ctrl Pts',(-1.23994455029421,-1.,-1.40845295531151));
#23006=CARTESIAN_POINT('Ctrl Pts',(-1.24450600513278,-1.,-1.41422913175437));
#23007=CARTESIAN_POINT('Ctrl Pts',(-1.24824430986911,-1.,-1.41923722596421));
#23008=CARTESIAN_POINT('Ctrl Pts',(-1.25141455570299,-1.,-1.42378102115911));
#23009=CARTESIAN_POINT('Ctrl Pts',(-1.25426945222783,-1.,-1.42815938799555));
#23010=CARTESIAN_POINT('Ctrl Pts',(-1.25702687965744,-1.,-1.43262645609679));
#23011=CARTESIAN_POINT('Ctrl Pts',(-1.25983531011894,-1.,-1.43734919180719));
#23012=CARTESIAN_POINT('Ctrl Pts',(-1.26273903323723,-1.,-1.44236470511145));
#23013=CARTESIAN_POINT('Ctrl Pts',(-1.26570925118767,-1.,-1.44761985001544));
#23014=CARTESIAN_POINT('Ctrl Pts',(-1.26867786804854,-1.,-1.45301422764205));
#23015=CARTESIAN_POINT('Ctrl Pts',(-1.27156805265312,-1.,-1.45843906294725));
#23016=CARTESIAN_POINT('Ctrl Pts',(-1.27433119897877,-1.,-1.4638243133254));
#23017=CARTESIAN_POINT('Ctrl Pts',(-1.27696414831144,-1.,-1.46916035917197));
#23018=CARTESIAN_POINT('Ctrl Pts',(-1.27948918248524,-1.,-1.4744717526711));
#23019=CARTESIAN_POINT('Ctrl Pts',(-1.28194158939522,-1.,-1.47980070347102));
#23020=CARTESIAN_POINT('Ctrl Pts',(-1.28435533880184,-1.,-1.48518817118891));
#23021=CARTESIAN_POINT('Ctrl Pts',(-1.28674676116415,-1.,-1.4906522831275));
#23022=CARTESIAN_POINT('Ctrl Pts',(-1.28911506584232,-1.,-1.49618896881729));
#23023=CARTESIAN_POINT('Ctrl Pts',(-1.29145022885171,-1.,-1.50178230149764));
#23024=CARTESIAN_POINT('Ctrl Pts',(-1.29373841372843,-1.,-1.50741159078367));
#23025=CARTESIAN_POINT('Ctrl Pts',(-1.29596850710518,-1.,-1.51305994241412));
#23026=CARTESIAN_POINT('Ctrl Pts',(-1.29813791800757,-1.,-1.51872184912735));
#23027=CARTESIAN_POINT('Ctrl Pts',(-1.30024984366334,-1.,-1.5243995786107));
#23028=CARTESIAN_POINT('Ctrl Pts',(-1.3023106439557,-1.,-1.53009970283893));
#23029=CARTESIAN_POINT('Ctrl Pts',(-1.30432735639487,-1.,-1.53582981268976));
#23030=CARTESIAN_POINT('Ctrl Pts',(-1.30630475189553,-1.,-1.54159462645428));
#23031=CARTESIAN_POINT('Ctrl Pts',(-1.30824393907471,-1.,-1.54739413957183));
#23032=CARTESIAN_POINT('Ctrl Pts',(-1.31014393684221,-1.,-1.55322568759481));
#23033=CARTESIAN_POINT('Ctrl Pts',(-1.31200264341696,-1.,-1.55908521254822));
#23034=CARTESIAN_POINT('Ctrl Pts',(-1.31381795281002,-1.,-1.56496872402352));
#23035=CARTESIAN_POINT('Ctrl Pts',(-1.31558903860015,-1.,-1.57087397835721));
#23036=CARTESIAN_POINT('Ctrl Pts',(-1.31731642317183,-1.,-1.57680056505585));
#23037=CARTESIAN_POINT('Ctrl Pts',(-1.31900135021428,-1.,-1.58274907898829));
#23038=CARTESIAN_POINT('Ctrl Pts',(-1.32064537110891,-1.,-1.58872057258244));
#23039=CARTESIAN_POINT('Ctrl Pts',(-1.32224985747686,-1.,-1.59471591079408));
#23040=CARTESIAN_POINT('Ctrl Pts',(-1.32381550858266,-1.,-1.600735118587));
#23041=CARTESIAN_POINT('Ctrl Pts',(-1.32534250785794,-1.,-1.6067775829097));
#23042=CARTESIAN_POINT('Ctrl Pts',(-1.32683074483365,-1.,-1.61284234015762));
#23043=CARTESIAN_POINT('Ctrl Pts',(-1.32828000610448,-1.,-1.61892832270723));
#23044=CARTESIAN_POINT('Ctrl Pts',(-1.32969019505665,-1.,-1.62503464209777));
#23045=CARTESIAN_POINT('Ctrl Pts',(-1.33106149345618,-1.,-1.63116079730887));
#23046=CARTESIAN_POINT('Ctrl Pts',(-1.33239425103694,-1.,-1.6373065347505));
#23047=CARTESIAN_POINT('Ctrl Pts',(-1.33368890676554,-1.,-1.64347174856007));
#23048=CARTESIAN_POINT('Ctrl Pts',(-1.33494590468003,-1.,-1.64965637286843));
#23049=CARTESIAN_POINT('Ctrl Pts',(-1.33616559745217,-1.,-1.65586025952651));
#23050=CARTESIAN_POINT('Ctrl Pts',(-1.33734820885331,-1.,-1.66208312542073));
#23051=CARTESIAN_POINT('Ctrl Pts',(-1.33849388654458,-1.,-1.66832460784078));
#23052=CARTESIAN_POINT('Ctrl Pts',(-1.33960273470372,-1.,-1.67458429426126));
#23053=CARTESIAN_POINT('Ctrl Pts',(-1.3406748518516,-1.,-1.68086176030308));
#23054=CARTESIAN_POINT('Ctrl Pts',(-1.34171037484673,-1.,-1.68715660868602));
#23055=CARTESIAN_POINT('Ctrl Pts',(-1.34270948206139,-1.,-1.6934684849664));
#23056=CARTESIAN_POINT('Ctrl Pts',(-1.34367237124322,-1.,-1.69979707754221));
#23057=CARTESIAN_POINT('Ctrl Pts',(-1.34459924533783,-1.,-1.70614212266676));
#23058=CARTESIAN_POINT('Ctrl Pts',(-1.34549029589563,-1.,-1.71250340687011));
#23059=CARTESIAN_POINT('Ctrl Pts',(-1.34634568653586,-1.,-1.7188807715095));
#23060=CARTESIAN_POINT('Ctrl Pts',(-1.34716554820013,-1.,-1.72527410681298));
#23061=CARTESIAN_POINT('Ctrl Pts',(-1.3477930915247,-1.,-1.73040149654497));
#23062=CARTESIAN_POINT('Ctrl Pts',(-1.34824783113158,-1.,-1.73425417886255));
#23063=CARTESIAN_POINT('Ctrl Pts',(-1.34854391898145,-1.,-1.73682580585819));
#23064=CARTESIAN_POINT('Ctrl Pts',(-1.34869019493419,-1.,-1.73811241238545));
#23065=CARTESIAN_POINT('',(-1.23627494547115,-1.,-1.81978687191668));
#23066=CARTESIAN_POINT('',(-1.34869019493419,-1.,-1.73811241238545));
#23067=CARTESIAN_POINT('',(-0.892032620296855,-1.,-1.5055822144029));
#23068=CARTESIAN_POINT('Ctrl Pts',(-1.23627494547115,-1.,-1.81978687191668));
#23069=CARTESIAN_POINT('Ctrl Pts',(-1.23509651170384,-1.,-1.81925017193531));
#23070=CARTESIAN_POINT('Ctrl Pts',(-1.23274224526804,-1.,-1.81817389920914));
#23071=CARTESIAN_POINT('Ctrl Pts',(-1.22921864890975,-1.,-1.81655087183054));
#23072=CARTESIAN_POINT('Ctrl Pts',(-1.22453613304507,-1.,-1.81436959209778));
#23073=CARTESIAN_POINT('Ctrl Pts',(-1.2187090610323,-1.,-1.81161420806172));
#23074=CARTESIAN_POINT('Ctrl Pts',(-1.2129081570818,-1.,-1.80882996916931));
#23075=CARTESIAN_POINT('Ctrl Pts',(-1.20713356605519,-1.,-1.80601678480772));
#23076=CARTESIAN_POINT('Ctrl Pts',(-1.2013854893912,-1.,-1.8031745483882));
#23077=CARTESIAN_POINT('Ctrl Pts',(-1.19566418930405,-1.,-1.80030314370121));
#23078=CARTESIAN_POINT('Ctrl Pts',(-1.1899699793456,-1.,-1.79740245923649));
#23079=CARTESIAN_POINT('Ctrl Pts',(-1.18430321697471,-1.,-1.79447240321572));
#23080=CARTESIAN_POINT('Ctrl Pts',(-1.17866429440781,-1.,-1.79151291552646));
#23081=CARTESIAN_POINT('Ctrl Pts',(-1.17305363177265,-1.,-1.78852398877523));
#23082=CARTESIAN_POINT('Ctrl Pts',(-1.16747166312239,-1.,-1.78550566040349));
#23083=CARTESIAN_POINT('Ctrl Pts',(-1.16191881298458,-1.,-1.78245795880949));
#23084=CARTESIAN_POINT('Ctrl Pts',(-1.15639547194689,-1.,-1.77938085564261));
#23085=CARTESIAN_POINT('Ctrl Pts',(-1.15090197841531,-1.,-1.77627422557034));
#23086=CARTESIAN_POINT('Ctrl Pts',(-1.14543858226948,-1.,-1.77313777896234));
#23087=CARTESIAN_POINT('Ctrl Pts',(-1.14000548337,-1.,-1.76997111386806));
#23088=CARTESIAN_POINT('Ctrl Pts',(-1.13460291804635,-1.,-1.76677384551883));
#23089=CARTESIAN_POINT('Ctrl Pts',(-1.12923123555076,-1.,-1.76354571966171));
#23090=CARTESIAN_POINT('Ctrl Pts',(-1.12389096855078,-1.,-1.76028671825084));
#23091=CARTESIAN_POINT('Ctrl Pts',(-1.11858293216752,-1.,-1.75699720772089));
#23092=CARTESIAN_POINT('Ctrl Pts',(-1.11330807582542,-1.,-1.75367772094617));
#23093=CARTESIAN_POINT('Ctrl Pts',(-1.10806728183003,-1.,-1.75032866075914));
#23094=CARTESIAN_POINT('Ctrl Pts',(-1.10286118991144,-1.,-1.74695004214924));
#23095=CARTESIAN_POINT('Ctrl Pts',(-1.09768999241229,-1.,-1.74354119236212));
#23096=CARTESIAN_POINT('Ctrl Pts',(-1.09255329056496,-1.,-1.74010053962252));
#23097=CARTESIAN_POINT('Ctrl Pts',(-1.08745056285429,-1.,-1.73662628326093));
#23098=CARTESIAN_POINT('Ctrl Pts',(-1.08238162784749,-1.,-1.73311705663407));
#23099=CARTESIAN_POINT('Ctrl Pts',(-1.0773470373727,-1.,-1.72957248977424));
#23100=CARTESIAN_POINT('Ctrl Pts',(-1.07234866990252,-1.,-1.72599406198489));
#23101=CARTESIAN_POINT('Ctrl Pts',(-1.06738966975463,-1.,-1.72238500928456));
#23102=CARTESIAN_POINT('Ctrl Pts',(-1.0624732468065,-1.,-1.71874858456908));
#23103=CARTESIAN_POINT('Ctrl Pts',(-1.05760163192481,-1.,-1.71508654427022));
#23104=CARTESIAN_POINT('Ctrl Pts',(-1.05277517202854,-1.,-1.71139783543986));
#23105=CARTESIAN_POINT('Ctrl Pts',(-1.0479908540499,-1.,-1.70767646263641));
#23106=CARTESIAN_POINT('Ctrl Pts',(-1.04324363334546,-1.,-1.70391338707969));
#23107=CARTESIAN_POINT('Ctrl Pts',(-1.03852922490782,-1.,-1.70010052930951));
#23108=CARTESIAN_POINT('Ctrl Pts',(-1.03384646003587,-1.,-1.69623414782769));
#23109=CARTESIAN_POINT('Ctrl Pts',(-1.02919977579155,-1.,-1.69231840863471));
#23110=CARTESIAN_POINT('Ctrl Pts',(-1.02460180535272,-1.,-1.68836910178475));
#23111=CARTESIAN_POINT('Ctrl Pts',(-1.02006795074222,-1.,-1.68440578021739));
#23112=CARTESIAN_POINT('Ctrl Pts',(-1.01561026162787,-1.,-1.6804428989482));
#23113=CARTESIAN_POINT('Ctrl Pts',(-1.01123236493507,-1.,-1.67648246776457));
#23114=CARTESIAN_POINT('Ctrl Pts',(-1.00692206696387,-1.,-1.67250335383248));
#23115=CARTESIAN_POINT('Ctrl Pts',(-1.00265091003682,-1.,-1.66846059277231));
#23116=CARTESIAN_POINT('Ctrl Pts',(-0.998389654952317,-1.,-1.66430758030304));
#23117=CARTESIAN_POINT('Ctrl Pts',(-0.994121836661116,-1.,-1.66001553809916));
#23118=CARTESIAN_POINT('Ctrl Pts',(-0.98985562785445,-1.,-1.65559044289746));
#23119=CARTESIAN_POINT('Ctrl Pts',(-0.985642622921626,-1.,-1.6511001661277));
#23120=CARTESIAN_POINT('Ctrl Pts',(-0.981562530940574,-1.,-1.64665139190834));
#23121=CARTESIAN_POINT('Ctrl Pts',(-0.977689794120297,-1.,-1.64233990826831));
#23122=CARTESIAN_POINT('Ctrl Pts',(-0.974066058287501,-1.,-1.63820952658157));
#23123=CARTESIAN_POINT('Ctrl Pts',(-0.970669715996356,-1.,-1.63420665729609));
#23124=CARTESIAN_POINT('Ctrl Pts',(-0.967387853228041,-1.,-1.63013849959083));
#23125=CARTESIAN_POINT('Ctrl Pts',(-0.964046107037821,-1.,-1.6257193066974));
#23126=CARTESIAN_POINT('Ctrl Pts',(-0.960438326099958,-1.,-1.62061638139929));
#23127=CARTESIAN_POINT('Ctrl Pts',(-0.956354422921573,-1.,-1.61449324337233));
#23128=CARTESIAN_POINT('Ctrl Pts',(-0.951613284361248,-1.,-1.60706069897794));
#23129=CARTESIAN_POINT('Ctrl Pts',(-0.946078063325796,-1.,-1.59810042045408));
#23130=CARTESIAN_POINT('Ctrl Pts',(-0.939646377909319,-1.,-1.58744937489796));
#23131=CARTESIAN_POINT('Ctrl Pts',(-0.932246680128849,-1.,-1.57499388385561));
#23132=CARTESIAN_POINT('Ctrl Pts',(-0.923832188966322,-1.,-1.56065988582509));
#23133=CARTESIAN_POINT('Ctrl Pts',(-0.91437591904658,-1.,-1.54440491152808));
#23134=CARTESIAN_POINT('Ctrl Pts',(-0.905967409640499,-1.,-1.52984849890434));
#23135=CARTESIAN_POINT('Ctrl Pts',(-0.89918504749193,-1.,-1.51805569591479));
#23136=CARTESIAN_POINT('Ctrl Pts',(-0.894452006967538,-1.,-1.50980486807181));
#23137=CARTESIAN_POINT('Ctrl Pts',(-0.892032620296855,-1.,-1.5055822144029));
#23138=CARTESIAN_POINT('',(-0.693717979106305,-1.,-1.60662857109684));
#23139=CARTESIAN_POINT('Origin',(0.,-1.,0.));
#23140=CARTESIAN_POINT('',(-0.745574324794401,-1.,-2.0698113262342));
#23141=CARTESIAN_POINT('Ctrl Pts',(-0.693717979106305,-1.,-1.60662857109684));
#23142=CARTESIAN_POINT('Ctrl Pts',(-0.69571209787897,-1.,-1.61106790957619));
#23143=CARTESIAN_POINT('Ctrl Pts',(-0.699605146398837,-1.,-1.61974673471117));
#23144=CARTESIAN_POINT('Ctrl Pts',(-0.705159151977294,-1.,-1.6321654166204));
#23145=CARTESIAN_POINT('Ctrl Pts',(-0.711993139340447,-1.,-1.64752408828442));
#23146=CARTESIAN_POINT('Ctrl Pts',(-0.71958543378795,-1.,-1.66472880551777));
#23147=CARTESIAN_POINT('Ctrl Pts',(-0.726235967982445,-1.,-1.67996158451922));
#23148=CARTESIAN_POINT('Ctrl Pts',(-0.731963238685357,-1.,-1.69326921972915));
#23149=CARTESIAN_POINT('Ctrl Pts',(-0.736799665716932,-1.,-1.70473309004249));
#23150=CARTESIAN_POINT('Ctrl Pts',(-0.74079516202821,-1.,-1.71447789751001));
#23151=CARTESIAN_POINT('Ctrl Pts',(-0.744021445433093,-1.,-1.72268229916769));
#23152=CARTESIAN_POINT('Ctrl Pts',(-0.746574710097752,-1.,-1.72958533647714));
#23153=CARTESIAN_POINT('Ctrl Pts',(-0.74858246295687,-1.,-1.7355035168033));
#23154=CARTESIAN_POINT('Ctrl Pts',(-0.750193435981249,-1.,-1.74080458267114));
#23155=CARTESIAN_POINT('Ctrl Pts',(-0.751555614164482,-1.,-1.74585086852502));
#23156=CARTESIAN_POINT('Ctrl Pts',(-0.752797683531314,-1.,-1.75095139468794));
#23157=CARTESIAN_POINT('Ctrl Pts',(-0.754009254027829,-1.,-1.75631083600019));
#23158=CARTESIAN_POINT('Ctrl Pts',(-0.755220979974461,-1.,-1.76197817240128));
#23159=CARTESIAN_POINT('Ctrl Pts',(-0.75642189602781,-1.,-1.76789396002998));
#23160=CARTESIAN_POINT('Ctrl Pts',(-0.757578264077029,-1.,-1.77394167108292));
#23161=CARTESIAN_POINT('Ctrl Pts',(-0.758650626677518,-1.,-1.77999411220945));
#23162=CARTESIAN_POINT('Ctrl Pts',(-0.759614401110189,-1.,-1.78596964884604));
#23163=CARTESIAN_POINT('Ctrl Pts',(-0.760469555880749,-1.,-1.7918581561088));
#23164=CARTESIAN_POINT('Ctrl Pts',(-0.761229695230558,-1.,-1.79768986997783));
#23165=CARTESIAN_POINT('Ctrl Pts',(-0.761915336443547,-1.,-1.80351583877342));
#23166=CARTESIAN_POINT('Ctrl Pts',(-0.762546129463938,-1.,-1.80938551463965));
#23167=CARTESIAN_POINT('Ctrl Pts',(-0.763132003836634,-1.,-1.8153211840553));
#23168=CARTESIAN_POINT('Ctrl Pts',(-0.763673465462726,-1.,-1.82131873145266));
#23169=CARTESIAN_POINT('Ctrl Pts',(-0.764165902605995,-1.,-1.82735991200065));
#23170=CARTESIAN_POINT('Ctrl Pts',(-0.764602549687853,-1.,-1.83342077227142));
#23171=CARTESIAN_POINT('Ctrl Pts',(-0.764978057881737,-1.,-1.83948181064835));
#23172=CARTESIAN_POINT('Ctrl Pts',(-0.765291664862029,-1.,-1.84553698875924));
#23173=CARTESIAN_POINT('Ctrl Pts',(-0.765545710619062,-1.,-1.85158945130063));
#23174=CARTESIAN_POINT('Ctrl Pts',(-0.765744212909318,-1.,-1.85764741390394));
#23175=CARTESIAN_POINT('Ctrl Pts',(-0.765891519092547,-1.,-1.86372027063312));
#23176=CARTESIAN_POINT('Ctrl Pts',(-0.765990708546091,-1.,-1.86981398314341));
#23177=CARTESIAN_POINT('Ctrl Pts',(-0.766042837036744,-1.,-1.87592888967883));
#23178=CARTESIAN_POINT('Ctrl Pts',(-0.766047794851865,-1.,-1.88206215302561));
#23179=CARTESIAN_POINT('Ctrl Pts',(-0.766004837062091,-1.,-1.88820926433409));
#23180=CARTESIAN_POINT('Ctrl Pts',(-0.765913193856978,-1.,-1.89436577771388));
#23181=CARTESIAN_POINT('Ctrl Pts',(-0.765772772593386,-1.,-1.90052930393596));
#23182=CARTESIAN_POINT('Ctrl Pts',(-0.765584196937919,-1.,-1.90669961402356));
#23183=CARTESIAN_POINT('Ctrl Pts',(-0.765348465884722,-1.,-1.91287765805169));
#23184=CARTESIAN_POINT('Ctrl Pts',(-0.765066729667088,-1.,-1.91906491634196));
#23185=CARTESIAN_POINT('Ctrl Pts',(-0.764740025488211,-1.,-1.92526263537048));
#23186=CARTESIAN_POINT('Ctrl Pts',(-0.764369010673941,-1.,-1.93147105496382));
#23187=CARTESIAN_POINT('Ctrl Pts',(-0.763954049121458,-1.,-1.93768964875886));
#23188=CARTESIAN_POINT('Ctrl Pts',(-0.763495333538629,-1.,-1.9439174661764));
#23189=CARTESIAN_POINT('Ctrl Pts',(-0.762992990878769,-1.,-1.95015342590024));
#23190=CARTESIAN_POINT('Ctrl Pts',(-0.762447203806179,-1.,-1.95639665309869));
#23191=CARTESIAN_POINT('Ctrl Pts',(-0.761858300014423,-1.,-1.96264672744186));
#23192=CARTESIAN_POINT('Ctrl Pts',(-0.76122669048382,-1.,-1.96890351582499));
#23193=CARTESIAN_POINT('Ctrl Pts',(-0.760552825409757,-1.,-1.97516705321494));
#23194=CARTESIAN_POINT('Ctrl Pts',(-0.75983714745219,-1.,-1.98143741418172));
#23195=CARTESIAN_POINT('Ctrl Pts',(-0.759080037802488,-1.,-1.98771456680874));
#23196=CARTESIAN_POINT('Ctrl Pts',(-0.758281796766761,-1.,-1.99399831098817));
#23197=CARTESIAN_POINT('Ctrl Pts',(-0.757442676862724,-1.,-2.00028834739178));
#23198=CARTESIAN_POINT('Ctrl Pts',(-0.75656290464667,-1.,-2.0065843158773));
#23199=CARTESIAN_POINT('Ctrl Pts',(-0.755642704957865,-1.,-2.01288584328084));
#23200=CARTESIAN_POINT('Ctrl Pts',(-0.754682330722816,-1.,-2.01919259405809));
#23201=CARTESIAN_POINT('Ctrl Pts',(-0.753682061112768,-1.,-2.02550428623313));
#23202=CARTESIAN_POINT('Ctrl Pts',(-0.752642180487211,-1.,-2.03182068456221));
#23203=CARTESIAN_POINT('Ctrl Pts',(-0.751562963361115,-1.,-2.03814160092099));
#23204=CARTESIAN_POINT('Ctrl Pts',(-0.750444657875576,-1.,-2.04446689147979));
#23205=CARTESIAN_POINT('Ctrl Pts',(-0.749287468665046,-1.,-2.05079645592154));
#23206=CARTESIAN_POINT('Ctrl Pts',(-0.748091554183802,-1.,-2.05713023031006));
#23207=CARTESIAN_POINT('Ctrl Pts',(-0.747103932787919,-1.,-2.06220058927826));
#23208=CARTESIAN_POINT('Ctrl Pts',(-0.7463458715442,-1.,-2.06600523016815));
#23209=CARTESIAN_POINT('Ctrl Pts',(-0.745832791378367,-1.,-2.06854248895728));
#23210=CARTESIAN_POINT('Ctrl Pts',(-0.745574324794401,-1.,-2.0698113262342));
#23211=CARTESIAN_POINT('',(-0.61342227326009,-1.,-2.11275013067528));
#23212=CARTESIAN_POINT('',(-0.745574324794401,-1.,-2.0698113262342));
#23213=CARTESIAN_POINT('',(-0.383122945602004,-1.,-1.7075470150345));
#23214=CARTESIAN_POINT('Ctrl Pts',(-0.61342227326009,-1.,-2.11275013067528));
#23215=CARTESIAN_POINT('Ctrl Pts',(-0.6124673655618,-1.,-2.11187554259986));
#23216=CARTESIAN_POINT('Ctrl Pts',(-0.610560911689899,-1.,-2.11012443807238));
#23217=CARTESIAN_POINT('Ctrl Pts',(-0.607711315454876,-1.,-2.1074919961518));
#23218=CARTESIAN_POINT('Ctrl Pts',(-0.60393203073603,-1.,-2.10397049886949));
#23219=CARTESIAN_POINT('Ctrl Pts',(-0.599241616420533,-1.,-2.0995493086477));
#23220=CARTESIAN_POINT('Ctrl Pts',(-0.594585006052162,-1.,-2.0951087622027));
#23221=CARTESIAN_POINT('Ctrl Pts',(-0.589962365403406,-1.,-2.09064881812129));
#23222=CARTESIAN_POINT('Ctrl Pts',(-0.585373918991617,-1.,-2.08616943727951));
#23223=CARTESIAN_POINT('Ctrl Pts',(-0.580819952108063,-1.,-2.08167059018418));
#23224=CARTESIAN_POINT('Ctrl Pts',(-0.576300797416844,-1.,-2.07715226767559));
#23225=CARTESIAN_POINT('Ctrl Pts',(-0.571816823242603,-1.,-2.07261449292824));
#23226=CARTESIAN_POINT('Ctrl Pts',(-0.567368421181087,-1.,-2.06805732997334));
#23227=CARTESIAN_POINT('Ctrl Pts',(-0.562955993082261,-1.,-2.06348090160589));
#23228=CARTESIAN_POINT('Ctrl Pts',(-0.558579940185151,-1.,-2.05888537756462));
#23229=CARTESIAN_POINT('Ctrl Pts',(-0.554240657463906,-1.,-2.05427091604413));
#23230=CARTESIAN_POINT('Ctrl Pts',(-0.549938525150295,-1.,-2.04963761077958));
#23231=CARTESIAN_POINT('Ctrl Pts',(-0.54567390381743,-1.,-2.04498544714588));
#23232=CARTESIAN_POINT('Ctrl Pts',(-0.541447120615659,-1.,-2.04031422690527));
#23233=CARTESIAN_POINT('Ctrl Pts',(-0.537258489833262,-1.,-2.03562362954037));
#23234=CARTESIAN_POINT('Ctrl Pts',(-0.533108355132977,-1.,-2.03091336214426));
#23235=CARTESIAN_POINT('Ctrl Pts',(-0.528997127241914,-1.,-2.0261832908329));
#23236=CARTESIAN_POINT('Ctrl Pts',(-0.524925318333476,-1.,-2.02143356304698));
#23237=CARTESIAN_POINT('Ctrl Pts',(-0.52089359039937,-1.,-2.01666477917286));
#23238=CARTESIAN_POINT('Ctrl Pts',(-0.516902681728687,-1.,-2.01187773939242));
#23239=CARTESIAN_POINT('Ctrl Pts',(-0.512953306961792,-1.,-2.00707309946949));
#23240=CARTESIAN_POINT('Ctrl Pts',(-0.509046069886157,-1.,-2.00225107134734));
#23241=CARTESIAN_POINT('Ctrl Pts',(-0.505181361323026,-1.,-1.99741107463572));
#23242=CARTESIAN_POINT('Ctrl Pts',(-0.501359287727146,-1.,-1.99255149126155));
#23243=CARTESIAN_POINT('Ctrl Pts',(-0.497579909545574,-1.,-1.98767044752932));
#23244=CARTESIAN_POINT('Ctrl Pts',(-0.493843476541495,-1.,-1.98276658761821));
#23245=CARTESIAN_POINT('Ctrl Pts',(-0.490150627860952,-1.,-1.97783973019229));
#23246=CARTESIAN_POINT('Ctrl Pts',(-0.486502692907659,-1.,-1.97289186263272));
#23247=CARTESIAN_POINT('Ctrl Pts',(-0.482901662120691,-1.,-1.96792703422362));
#23248=CARTESIAN_POINT('Ctrl Pts',(-0.479349583074855,-1.,-1.96294933055943));
#23249=CARTESIAN_POINT('Ctrl Pts',(-0.475848034683176,-1.,-1.95796111148177));
#23250=CARTESIAN_POINT('Ctrl Pts',(-0.472397672264072,-1.,-1.95296148278133));
#23251=CARTESIAN_POINT('Ctrl Pts',(-0.468997482913135,-1.,-1.94794381136514));
#23252=CARTESIAN_POINT('Ctrl Pts',(-0.46564546202603,-1.,-1.9428979419619));
#23253=CARTESIAN_POINT('Ctrl Pts',(-0.462340031009056,-1.,-1.93781486640821));
#23254=CARTESIAN_POINT('Ctrl Pts',(-0.459081234547926,-1.,-1.93269066517934));
#23255=CARTESIAN_POINT('Ctrl Pts',(-0.455872005174371,-1.,-1.92753067150476));
#23256=CARTESIAN_POINT('Ctrl Pts',(-0.452719478359432,-1.,-1.92235380648502));
#23257=CARTESIAN_POINT('Ctrl Pts',(-0.449632260106662,-1.,-1.91718342555755));
#23258=CARTESIAN_POINT('Ctrl Pts',(-0.446617343485711,-1.,-1.9120369998112));
#23259=CARTESIAN_POINT('Ctrl Pts',(-0.443677556849151,-1.,-1.90691756144898));
#23260=CARTESIAN_POINT('Ctrl Pts',(-0.440807833704038,-1.,-1.90180124389086));
#23261=CARTESIAN_POINT('Ctrl Pts',(-0.437995003948244,-1.,-1.89663648956466));
#23262=CARTESIAN_POINT('Ctrl Pts',(-0.435225660963383,-1.,-1.89136993975504));
#23263=CARTESIAN_POINT('Ctrl Pts',(-0.432493038548748,-1.,-1.88596913666793));
#23264=CARTESIAN_POINT('Ctrl Pts',(-0.429803062482344,-1.,-1.88044229001832));
#23265=CARTESIAN_POINT('Ctrl Pts',(-0.427183828519102,-1.,-1.87486989291484));
#23266=CARTESIAN_POINT('Ctrl Pts',(-0.424678177291359,-1.,-1.86937803944323));
#23267=CARTESIAN_POINT('Ctrl Pts',(-0.422327307418275,-1.,-1.86408083334028));
#23268=CARTESIAN_POINT('Ctrl Pts',(-0.420157287975619,-1.,-1.85903281096686));
#23269=CARTESIAN_POINT('Ctrl Pts',(-0.418164129143534,-1.,-1.85417632856234));
#23270=CARTESIAN_POINT('Ctrl Pts',(-0.416300022038864,-1.,-1.84929312929882));
#23271=CARTESIAN_POINT('Ctrl Pts',(-0.41448743825434,-1.,-1.8440575707371));
#23272=CARTESIAN_POINT('Ctrl Pts',(-0.412633125322162,-1.,-1.83808953475839));
#23273=CARTESIAN_POINT('Ctrl Pts',(-0.410641256301675,-1.,-1.83100408895216));
#23274=CARTESIAN_POINT('Ctrl Pts',(-0.408428948108533,-1.,-1.8224702267854));
#23275=CARTESIAN_POINT('Ctrl Pts',(-0.405933518411838,-1.,-1.81223801813988));
#23276=CARTESIAN_POINT('Ctrl Pts',(-0.403107976170441,-1.,-1.80012077176221));
#23277=CARTESIAN_POINT('Ctrl Pts',(-0.39991940378308,-1.,-1.78598826347533));
#23278=CARTESIAN_POINT('Ctrl Pts',(-0.39634619612042,-1.,-1.7697556004756));
#23279=CARTESIAN_POINT('Ctrl Pts',(-0.392375812294307,-1.,-1.75137405313962));
#23280=CARTESIAN_POINT('Ctrl Pts',(-0.388877023509191,-1.,-1.7349317097561));
#23281=CARTESIAN_POINT('Ctrl Pts',(-0.38607079032701,-1.,-1.72162022246158));
#23282=CARTESIAN_POINT('Ctrl Pts',(-0.384119047315542,-1.,-1.71231062891958));
#23283=CARTESIAN_POINT('Ctrl Pts',(-0.383122945602004,-1.,-1.7075470150345));
#23284=CARTESIAN_POINT('',(-0.163289472382896,-1.,-1.74236521665491));
#23285=CARTESIAN_POINT('Origin',(0.,-1.,0.));
#23286=CARTESIAN_POINT('',(-0.0694764450219581,-1.,-2.19890268624765));
#23287=CARTESIAN_POINT('Ctrl Pts',(-0.163289472382896,-1.,-1.74236521665491));
#23288=CARTESIAN_POINT('Ctrl Pts',(-0.163814161002002,-1.,-1.7472034950333));
#23289=CARTESIAN_POINT('Ctrl Pts',(-0.164834765707158,-1.,-1.75666056638427));
#23290=CARTESIAN_POINT('Ctrl Pts',(-0.1662793551464,-1.,-1.77018771684844));
#23291=CARTESIAN_POINT('Ctrl Pts',(-0.168032772805197,-1.,-1.7869064998507));
#23292=CARTESIAN_POINT('Ctrl Pts',(-0.169936923904608,-1.,-1.80561530629706));
#23293=CARTESIAN_POINT('Ctrl Pts',(-0.171554770204119,-1.,-1.82215766811545));
#23294=CARTESIAN_POINT('Ctrl Pts',(-0.1728894428919,-1.,-1.83658380527692));
#23295=CARTESIAN_POINT('Ctrl Pts',(-0.173946627587731,-1.,-1.8489811319852));
#23296=CARTESIAN_POINT('Ctrl Pts',(-0.17473525927603,-1.,-1.85948367088837));
#23297=CARTESIAN_POINT('Ctrl Pts',(-0.175268337590758,-1.,-1.86828349694799));
#23298=CARTESIAN_POINT('Ctrl Pts',(-0.175563480746485,-1.,-1.87563767773588));
#23299=CARTESIAN_POINT('Ctrl Pts',(-0.175644148889699,-1.,-1.88188663145367));
#23300=CARTESIAN_POINT('Ctrl Pts',(-0.175538155840648,-1.,-1.88742606273259));
#23301=CARTESIAN_POINT('Ctrl Pts',(-0.175274276190844,-1.,-1.892646301985));
#23302=CARTESIAN_POINT('Ctrl Pts',(-0.174879405091263,-1.,-1.89788101117132));
#23303=CARTESIAN_POINT('Ctrl Pts',(-0.174375518661085,-1.,-1.90335253862834));
#23304=CARTESIAN_POINT('Ctrl Pts',(-0.173776635257817,-1.,-1.90911693975267));
#23305=CARTESIAN_POINT('Ctrl Pts',(-0.173090695383496,-1.,-1.91511429159527));
#23306=CARTESIAN_POINT('Ctrl Pts',(-0.172321621259514,-1.,-1.9212233439798));
#23307=CARTESIAN_POINT('Ctrl Pts',(-0.171471191532988,-1.,-1.92731093582036));
#23308=CARTESIAN_POINT('Ctrl Pts',(-0.170541253116202,-1.,-1.93329183155539));
#23309=CARTESIAN_POINT('Ctrl Pts',(-0.169534904817491,-1.,-1.93915639211581));
#23310=CARTESIAN_POINT('Ctrl Pts',(-0.168455741607556,-1.,-1.94493757756931));
#23311=CARTESIAN_POINT('Ctrl Pts',(-0.167307501784475,-1.,-1.95069027794294));
#23312=CARTESIAN_POINT('Ctrl Pts',(-0.166093592002812,-1.,-1.9564675971873));
#23313=CARTESIAN_POINT('Ctrl Pts',(-0.164816568920269,-1.,-1.96229379940136));
#23314=CARTESIAN_POINT('Ctrl Pts',(-0.163478185457734,-1.,-1.96816512677967));
#23315=CARTESIAN_POINT('Ctrl Pts',(-0.162079693556289,-1.,-1.97406280235188));
#23316=CARTESIAN_POINT('Ctrl Pts',(-0.160622060784611,-1.,-1.97996195437559));
#23317=CARTESIAN_POINT('Ctrl Pts',(-0.159106226437299,-1.,-1.98584238283292));
#23318=CARTESIAN_POINT('Ctrl Pts',(-0.157533331459227,-1.,-1.99169810931908));
#23319=CARTESIAN_POINT('Ctrl Pts',(-0.155904629548783,-1.,-1.99753284771497));
#23320=CARTESIAN_POINT('Ctrl Pts',(-0.154221403049722,-1.,-2.00335565310543));
#23321=CARTESIAN_POINT('Ctrl Pts',(-0.15248488362145,-1.,-2.00917680318424));
#23322=CARTESIAN_POINT('Ctrl Pts',(-0.150696157673078,-1.,-2.01500291940238));
#23323=CARTESIAN_POINT('Ctrl Pts',(-0.148856124775337,-1.,-2.02083464969894));
#23324=CARTESIAN_POINT('Ctrl Pts',(-0.146965557332583,-1.,-2.02666926182017));
#23325=CARTESIAN_POINT('Ctrl Pts',(-0.145025140186057,-1.,-2.03250223739942));
#23326=CARTESIAN_POINT('Ctrl Pts',(-0.143035515058209,-1.,-2.03832911025912));
#23327=CARTESIAN_POINT('Ctrl Pts',(-0.140997332152546,-1.,-2.04414757947916));
#23328=CARTESIAN_POINT('Ctrl Pts',(-0.138911255368966,-1.,-2.04995762001328));
#23329=CARTESIAN_POINT('Ctrl Pts',(-0.136777941218044,-1.,-2.05576044414264));
#23330=CARTESIAN_POINT('Ctrl Pts',(-0.134598026192106,-1.,-2.06155781517842));
#23331=CARTESIAN_POINT('Ctrl Pts',(-0.13237211154771,-1.,-2.06735123910326));
#23332=CARTESIAN_POINT('Ctrl Pts',(-0.130100748328403,-1.,-2.07314114713063));
#23333=CARTESIAN_POINT('Ctrl Pts',(-0.12778444527612,-1.,-2.07892715110987));
#23334=CARTESIAN_POINT('Ctrl Pts',(-0.125423679412061,-1.,-2.08470840653643));
#23335=CARTESIAN_POINT('Ctrl Pts',(-0.123018905621083,-1.,-2.09048392424825));
#23336=CARTESIAN_POINT('Ctrl Pts',(-0.120570567965122,-1.,-2.0962529286773));
#23337=CARTESIAN_POINT('Ctrl Pts',(-0.118079107988355,-1.,-2.102015121329));
#23338=CARTESIAN_POINT('Ctrl Pts',(-0.115544957687926,-1.,-2.10777050261309));
#23339=CARTESIAN_POINT('Ctrl Pts',(-0.112968534419737,-1.,-2.11351924490306));
#23340=CARTESIAN_POINT('Ctrl Pts',(-0.110350236135025,-1.,-2.11926155590865));
#23341=CARTESIAN_POINT('Ctrl Pts',(-0.10769043523109,-1.,-2.12499752307));
#23342=CARTESIAN_POINT('Ctrl Pts',(-0.104989479152739,-1.,-2.13072704887293));
#23343=CARTESIAN_POINT('Ctrl Pts',(-0.1022477005561,-1.,-2.13644992667165));
#23344=CARTESIAN_POINT('Ctrl Pts',(-0.0994654261990915,-1.,-2.14216588396025));
#23345=CARTESIAN_POINT('Ctrl Pts',(-0.0966429852305459,-1.,-2.14787463531795));
#23346=CARTESIAN_POINT('Ctrl Pts',(-0.0937807218867643,-1.,-2.1535759397817));
#23347=CARTESIAN_POINT('Ctrl Pts',(-0.0908789888107265,-1.,-2.15926961544516));
#23348=CARTESIAN_POINT('Ctrl Pts',(-0.0879381291386923,-1.,-2.16495552645014));
#23349=CARTESIAN_POINT('Ctrl Pts',(-0.0849584620835372,-1.,-2.17063357870952));
#23350=CARTESIAN_POINT('Ctrl Pts',(-0.0819402680872765,-1.,-2.176303712113));
#23351=CARTESIAN_POINT('Ctrl Pts',(-0.0788837727685243,-1.,-2.18196589448887));
#23352=CARTESIAN_POINT('Ctrl Pts',(-0.0757891465836148,-1.,-2.1876201139953));
#23353=CARTESIAN_POINT('Ctrl Pts',(-0.0732830357306725,-1.,-2.19213712013662));
#23354=CARTESIAN_POINT('Ctrl Pts',(-0.0713863779526154,-1.,-2.19552129484002));
#23355=CARTESIAN_POINT('Ctrl Pts',(-0.070114353632549,-1.,-2.19777582085423));
#23356=CARTESIAN_POINT('Ctrl Pts',(-0.0694764450219581,-1.,-2.19890268624765));
#23357=CARTESIAN_POINT('',(0.0694764450219584,-1.,-2.19890268624765));
#23358=CARTESIAN_POINT('',(-0.0694764450219581,-1.,-2.19890268624765));
#23359=CARTESIAN_POINT('',(0.163289472382896,-1.,-1.74236521665491));
#23360=CARTESIAN_POINT('Ctrl Pts',(0.0694764450219584,-1.,-2.19890268624765));
#23361=CARTESIAN_POINT('Ctrl Pts',(0.0701143536324926,-1.,-2.19777582085261));
#23362=CARTESIAN_POINT('Ctrl Pts',(0.0713863779524627,-1.,-2.19552129483562));
#23363=CARTESIAN_POINT('Ctrl Pts',(0.0732830357304276,-1.,-2.19213712012956));
#23364=CARTESIAN_POINT('Ctrl Pts',(0.0757891465833411,-1.,-2.1876201139874));
#23365=CARTESIAN_POINT('Ctrl Pts',(0.0788837727683228,-1.,-2.18196589448304));
#23366=CARTESIAN_POINT('Ctrl Pts',(0.0819402680871939,-1.,-2.1763037121106));
#23367=CARTESIAN_POINT('Ctrl Pts',(0.0849584620835643,-1.,-2.17063357871031));
#23368=CARTESIAN_POINT('Ctrl Pts',(0.0879381291387823,-1.,-2.16495552645275));
#23369=CARTESIAN_POINT('Ctrl Pts',(0.0908789888108266,-1.,-2.15926961544808));
#23370=CARTESIAN_POINT('Ctrl Pts',(0.0937807218868345,-1.,-2.15357593978377));
#23371=CARTESIAN_POINT('Ctrl Pts',(0.0966429852305689,-1.,-2.14787463531864));
#23372=CARTESIAN_POINT('Ctrl Pts',(0.0994654261990743,-1.,-2.14216588395974));
#23373=CARTESIAN_POINT('Ctrl Pts',(0.102247700556064,-1.,-2.13644992667052));
#23374=CARTESIAN_POINT('Ctrl Pts',(0.104989479152703,-1.,-2.1307270488718));
#23375=CARTESIAN_POINT('Ctrl Pts',(0.107690435231068,-1.,-2.12499752306927));
#23376=CARTESIAN_POINT('Ctrl Pts',(0.11035023613502,-1.,-2.11926155590849));
#23377=CARTESIAN_POINT('Ctrl Pts',(0.112968534419746,-1.,-2.11351924490335));
#23378=CARTESIAN_POINT('Ctrl Pts',(0.11554495768794,-1.,-2.10777050261359));
#23379=CARTESIAN_POINT('Ctrl Pts',(0.118079107988368,-1.,-2.10201512132945));
#23380=CARTESIAN_POINT('Ctrl Pts',(0.120570567965129,-1.,-2.09625292867756));
#23381=CARTESIAN_POINT('Ctrl Pts',(0.123018905621083,-1.,-2.09048392424826));
#23382=CARTESIAN_POINT('Ctrl Pts',(0.125423679412058,-1.,-2.08470840653628));
#23383=CARTESIAN_POINT('Ctrl Pts',(0.127784445276116,-1.,-2.07892715110967));
#23384=CARTESIAN_POINT('Ctrl Pts',(0.1301007483284,-1.,-2.07314114713047));
#23385=CARTESIAN_POINT('Ctrl Pts',(0.13237211154771,-1.,-2.06735123910319));
#23386=CARTESIAN_POINT('Ctrl Pts',(0.134598026192107,-1.,-2.06155781517844));
#23387=CARTESIAN_POINT('Ctrl Pts',(0.136777941218044,-1.,-2.0557604441427));
#23388=CARTESIAN_POINT('Ctrl Pts',(0.138911255368966,-1.,-2.04995762001333));
#23389=CARTESIAN_POINT('Ctrl Pts',(0.140997332152545,-1.,-2.04414757947919));
#23390=CARTESIAN_POINT('Ctrl Pts',(0.143035515058208,-1.,-2.03832911025913));
#23391=CARTESIAN_POINT('Ctrl Pts',(0.145025140186058,-1.,-2.03250223739941));
#23392=CARTESIAN_POINT('Ctrl Pts',(0.146965557332586,-1.,-2.02666926182017));
#23393=CARTESIAN_POINT('Ctrl Pts',(0.148856124775343,-1.,-2.02083464969897));
#23394=CARTESIAN_POINT('Ctrl Pts',(0.150696157673084,-1.,-2.01500291940243));
#23395=CARTESIAN_POINT('Ctrl Pts',(0.152484883621452,-1.,-2.00917680318426));
#23396=CARTESIAN_POINT('Ctrl Pts',(0.154221403049719,-1.,-2.00335565310539));
#23397=CARTESIAN_POINT('Ctrl Pts',(0.155904629548774,-1.,-1.99753284771487));
#23398=CARTESIAN_POINT('Ctrl Pts',(0.157533331459215,-1.,-1.99169810931893));
#23399=CARTESIAN_POINT('Ctrl Pts',(0.159106226437288,-1.,-1.98584238283279));
#23400=CARTESIAN_POINT('Ctrl Pts',(0.16062206078461,-1.,-1.97996195437557));
#23401=CARTESIAN_POINT('Ctrl Pts',(0.162079693556302,-1.,-1.97406280235204));
#23402=CARTESIAN_POINT('Ctrl Pts',(0.16347818545776,-1.,-1.96816512678));
#23403=CARTESIAN_POINT('Ctrl Pts',(0.1648165689203,-1.,-1.96229379940174));
#23404=CARTESIAN_POINT('Ctrl Pts',(0.166093592002833,-1.,-1.95646759718755));
#23405=CARTESIAN_POINT('Ctrl Pts',(0.167307501784469,-1.,-1.95069027794286));
#23406=CARTESIAN_POINT('Ctrl Pts',(0.168455741607516,-1.,-1.94493757756879));
#23407=CARTESIAN_POINT('Ctrl Pts',(0.169534904817425,-1.,-1.93915639211497));
#23408=CARTESIAN_POINT('Ctrl Pts',(0.170541253116136,-1.,-1.93329183155455));
#23409=CARTESIAN_POINT('Ctrl Pts',(0.17147119153296,-1.,-1.92731093582));
#23410=CARTESIAN_POINT('Ctrl Pts',(0.172321621259557,-1.,-1.92122334398034));
#23411=CARTESIAN_POINT('Ctrl Pts',(0.173090695383619,-1.,-1.91511429159681));
#23412=CARTESIAN_POINT('Ctrl Pts',(0.173776635257984,-1.,-1.90911693975475));
#23413=CARTESIAN_POINT('Ctrl Pts',(0.174375518661222,-1.,-1.90335253863003));
#23414=CARTESIAN_POINT('Ctrl Pts',(0.174879405091277,-1.,-1.89788101117148));
#23415=CARTESIAN_POINT('Ctrl Pts',(0.175274276190664,-1.,-1.89264630198279));
#23416=CARTESIAN_POINT('Ctrl Pts',(0.175538155840286,-1.,-1.88742606272818));
#23417=CARTESIAN_POINT('Ctrl Pts',(0.175644148889271,-1.,-1.88188663144846));
#23418=CARTESIAN_POINT('Ctrl Pts',(0.175563480746205,-1.,-1.87563767773249));
#23419=CARTESIAN_POINT('Ctrl Pts',(0.175268337590901,-1.,-1.86828349694972));
#23420=CARTESIAN_POINT('Ctrl Pts',(0.174735259276856,-1.,-1.85948367089838));
#23421=CARTESIAN_POINT('Ctrl Pts',(0.173946627589401,-1.,-1.84898113200543));
#23422=CARTESIAN_POINT('Ctrl Pts',(0.17288944289442,-1.,-1.83658380530747));
#23423=CARTESIAN_POINT('Ctrl Pts',(0.171554770207306,-1.,-1.82215766815414));
#23424=CARTESIAN_POINT('Ctrl Pts',(0.169936923908078,-1.,-1.80561530633924));
#23425=CARTESIAN_POINT('Ctrl Pts',(0.16803277280837,-1.,-1.78690649988931));
#23426=CARTESIAN_POINT('Ctrl Pts',(0.166279355148738,-1.,-1.77018771687692));
#23427=CARTESIAN_POINT('Ctrl Pts',(0.164834765708484,-1.,-1.75666056640041));
#23428=CARTESIAN_POINT('Ctrl Pts',(0.163814161002474,-1.,-1.74720349503904));
#23429=CARTESIAN_POINT('Ctrl Pts',(0.163289472382896,-1.,-1.74236521665491));
#23430=CARTESIAN_POINT('',(0.383122945602004,-1.,-1.7075470150345));
#23431=CARTESIAN_POINT('Origin',(0.,-1.,0.));
#23432=CARTESIAN_POINT('',(0.61342227326009,-1.,-2.11275013067528));
#23433=CARTESIAN_POINT('Ctrl Pts',(0.383122945602004,-1.,-1.7075470150345));
#23434=CARTESIAN_POINT('Ctrl Pts',(0.384119047314215,-1.,-1.71231062891398));
#23435=CARTESIAN_POINT('Ctrl Pts',(0.386070790323281,-1.,-1.72162022244582));
#23436=CARTESIAN_POINT('Ctrl Pts',(0.388877023502615,-1.,-1.73493170972829));
#23437=CARTESIAN_POINT('Ctrl Pts',(0.392375812285395,-1.,-1.75137405310193));
#23438=CARTESIAN_POINT('Ctrl Pts',(0.396346196110688,-1.,-1.76975560043442));
#23439=CARTESIAN_POINT('Ctrl Pts',(0.399919403774155,-1.,-1.78598826343754));
#23440=CARTESIAN_POINT('Ctrl Pts',(0.403107976163396,-1.,-1.80012077173238));
#23441=CARTESIAN_POINT('Ctrl Pts',(0.405933518407175,-1.,-1.81223801812013));
#23442=CARTESIAN_POINT('Ctrl Pts',(0.408428948106227,-1.,-1.82247022677562));
#23443=CARTESIAN_POINT('Ctrl Pts',(0.410641256301276,-1.,-1.83100408895047));
#23444=CARTESIAN_POINT('Ctrl Pts',(0.412633125322945,-1.,-1.8380895347617));
#23445=CARTESIAN_POINT('Ctrl Pts',(0.414487438255542,-1.,-1.84405757074218));
#23446=CARTESIAN_POINT('Ctrl Pts',(0.416300022039885,-1.,-1.84929312930314));
#23447=CARTESIAN_POINT('Ctrl Pts',(0.418164129144045,-1.,-1.8541763285645));
#23448=CARTESIAN_POINT('Ctrl Pts',(0.420157287975583,-1.,-1.8590328109667));
#23449=CARTESIAN_POINT('Ctrl Pts',(0.422327307417884,-1.,-1.86408083333863));
#23450=CARTESIAN_POINT('Ctrl Pts',(0.424678177290876,-1.,-1.8693780394412));
#23451=CARTESIAN_POINT('Ctrl Pts',(0.427183828518743,-1.,-1.87486989291334));
#23452=CARTESIAN_POINT('Ctrl Pts',(0.429803062482217,-1.,-1.88044229001779));
#23453=CARTESIAN_POINT('Ctrl Pts',(0.432493038548833,-1.,-1.88596913666828));
#23454=CARTESIAN_POINT('Ctrl Pts',(0.43522566096358,-1.,-1.89136993975585));
#23455=CARTESIAN_POINT('Ctrl Pts',(0.437995003948443,-1.,-1.89663648956549));
#23456=CARTESIAN_POINT('Ctrl Pts',(0.44080783370416,-1.,-1.90180124389137));
#23457=CARTESIAN_POINT('Ctrl Pts',(0.44367755684917,-1.,-1.90691756144906));
#23458=CARTESIAN_POINT('Ctrl Pts',(0.446617343485651,-1.,-1.91203699981095));
#23459=CARTESIAN_POINT('Ctrl Pts',(0.449632260106572,-1.,-1.91718342555717));
#23460=CARTESIAN_POINT('Ctrl Pts',(0.452719478359356,-1.,-1.9223538064847));
#23461=CARTESIAN_POINT('Ctrl Pts',(0.455872005174335,-1.,-1.92753067150461));
#23462=CARTESIAN_POINT('Ctrl Pts',(0.459081234547931,-1.,-1.93269066517936));
#23463=CARTESIAN_POINT('Ctrl Pts',(0.462340031009087,-1.,-1.93781486640834));
#23464=CARTESIAN_POINT('Ctrl Pts',(0.465645462026064,-1.,-1.94289794196205));
#23465=CARTESIAN_POINT('Ctrl Pts',(0.468997482913158,-1.,-1.94794381136524));
#23466=CARTESIAN_POINT('Ctrl Pts',(0.472397672264079,-1.,-1.95296148278136));
#23467=CARTESIAN_POINT('Ctrl Pts',(0.475848034683171,-1.,-1.95796111148175));
#23468=CARTESIAN_POINT('Ctrl Pts',(0.479349583074846,-1.,-1.96294933055938));
#23469=CARTESIAN_POINT('Ctrl Pts',(0.482901662120686,-1.,-1.96792703422358));
#23470=CARTESIAN_POINT('Ctrl Pts',(0.486502692907661,-1.,-1.97289186263272));
#23471=CARTESIAN_POINT('Ctrl Pts',(0.490150627860955,-1.,-1.97783973019229));
#23472=CARTESIAN_POINT('Ctrl Pts',(0.493843476541492,-1.,-1.9827665876182));
#23473=CARTESIAN_POINT('Ctrl Pts',(0.497579909545564,-1.,-1.98767044752929));
#23474=CARTESIAN_POINT('Ctrl Pts',(0.501359287727129,-1.,-1.9925514912615));
#23475=CARTESIAN_POINT('Ctrl Pts',(0.505181361323011,-1.,-1.99741107463567));
#23476=CARTESIAN_POINT('Ctrl Pts',(0.509046069886152,-1.,-2.00225107134733));
#23477=CARTESIAN_POINT('Ctrl Pts',(0.512953306961813,-1.,-2.00707309946955));
#23478=CARTESIAN_POINT('Ctrl Pts',(0.516902681728733,-1.,-2.01187773939257));
#23479=CARTESIAN_POINT('Ctrl Pts',(0.520893590399428,-1.,-2.01666477917306));
#23480=CARTESIAN_POINT('Ctrl Pts',(0.524925318333518,-1.,-2.02143356304712));
#23481=CARTESIAN_POINT('Ctrl Pts',(0.52899712724191,-1.,-2.02618329083289));
#23482=CARTESIAN_POINT('Ctrl Pts',(0.533108355132905,-1.,-2.03091336214401));
#23483=CARTESIAN_POINT('Ctrl Pts',(0.537258489833134,-1.,-2.03562362953993));
#23484=CARTESIAN_POINT('Ctrl Pts',(0.54144712061552,-1.,-2.0403142269048));
#23485=CARTESIAN_POINT('Ctrl Pts',(0.545673903817348,-1.,-2.0449854471456));
#23486=CARTESIAN_POINT('Ctrl Pts',(0.549938525150342,-1.,-2.04963761077974));
#23487=CARTESIAN_POINT('Ctrl Pts',(0.554240657464109,-1.,-2.05427091604482));
#23488=CARTESIAN_POINT('Ctrl Pts',(0.558579940185467,-1.,-2.05888537756571));
#23489=CARTESIAN_POINT('Ctrl Pts',(0.562955993082574,-1.,-2.06348090160697));
#23490=CARTESIAN_POINT('Ctrl Pts',(0.567368421181229,-1.,-2.06805732997383));
#23491=CARTESIAN_POINT('Ctrl Pts',(0.571816823242411,-1.,-2.07261449292758));
#23492=CARTESIAN_POINT('Ctrl Pts',(0.576300797416274,-1.,-2.07715226767361));
#23493=CARTESIAN_POINT('Ctrl Pts',(0.580819952107256,-1.,-2.08167059018138));
#23494=CARTESIAN_POINT('Ctrl Pts',(0.585373918990895,-1.,-2.086169437277));
#23495=CARTESIAN_POINT('Ctrl Pts',(0.589962365403189,-1.,-2.09064881812053));
#23496=CARTESIAN_POINT('Ctrl Pts',(0.594585006052823,-1.,-2.09510876220501));
#23497=CARTESIAN_POINT('Ctrl Pts',(0.599241616422144,-1.,-2.09954930865331));
#23498=CARTESIAN_POINT('Ctrl Pts',(0.603932030738212,-1.,-2.10397049887709));
#23499=CARTESIAN_POINT('Ctrl Pts',(0.607711315456826,-1.,-2.10749199615859));
#23500=CARTESIAN_POINT('Ctrl Pts',(0.610560911691113,-1.,-2.11012443807661));
#23501=CARTESIAN_POINT('Ctrl Pts',(0.61246736556225,-1.,-2.11187554260142));
#23502=CARTESIAN_POINT('Ctrl Pts',(0.61342227326009,-1.,-2.11275013067528));
#23503=CARTESIAN_POINT('',(0.745574324794401,-1.,-2.0698113262342));
#23504=CARTESIAN_POINT('',(0.61342227326009,-1.,-2.11275013067528));
#23505=CARTESIAN_POINT('',(0.693717979106306,-1.,-1.60662857109684));
#23506=CARTESIAN_POINT('Ctrl Pts',(0.745574324794401,-1.,-2.0698113262342));
#23507=CARTESIAN_POINT('Ctrl Pts',(0.74583279137781,-1.,-2.06854248895575));
#23508=CARTESIAN_POINT('Ctrl Pts',(0.746345871542695,-1.,-2.06600523016401));
#23509=CARTESIAN_POINT('Ctrl Pts',(0.747103932785504,-1.,-2.06220058927162));
#23510=CARTESIAN_POINT('Ctrl Pts',(0.748091554181101,-1.,-2.05713023030263));
#23511=CARTESIAN_POINT('Ctrl Pts',(0.749287468663053,-1.,-2.05079645591606));
#23512=CARTESIAN_POINT('Ctrl Pts',(0.750444657874758,-1.,-2.04446689147754));
#23513=CARTESIAN_POINT('Ctrl Pts',(0.751562963361383,-1.,-2.03814160092173));
#23514=CARTESIAN_POINT('Ctrl Pts',(0.752642180488104,-1.,-2.03182068456467));
#23515=CARTESIAN_POINT('Ctrl Pts',(0.753682061113765,-1.,-2.02550428623587));
#23516=CARTESIAN_POINT('Ctrl Pts',(0.75468233072352,-1.,-2.01919259406003));
#23517=CARTESIAN_POINT('Ctrl Pts',(0.7556427049581,-1.,-2.01288584328149));
#23518=CARTESIAN_POINT('Ctrl Pts',(0.756562904646496,-1.,-2.00658431587682));
#23519=CARTESIAN_POINT('Ctrl Pts',(0.757442676862341,-1.,-2.00028834739072));
#23520=CARTESIAN_POINT('Ctrl Pts',(0.758281796766377,-1.,-1.9939983109871));
#23521=CARTESIAN_POINT('Ctrl Pts',(0.759080037802242,-1.,-1.98771456680806));
#23522=CARTESIAN_POINT('Ctrl Pts',(0.759837147452135,-1.,-1.98143741418156));
#23523=CARTESIAN_POINT('Ctrl Pts',(0.760552825409855,-1.,-1.97516705321521));
#23524=CARTESIAN_POINT('Ctrl Pts',(0.761226690483986,-1.,-1.96890351582545));
#23525=CARTESIAN_POINT('Ctrl Pts',(0.761858300014575,-1.,-1.96264672744229));
#23526=CARTESIAN_POINT('Ctrl Pts',(0.762447203806263,-1.,-1.95639665309893));
#23527=CARTESIAN_POINT('Ctrl Pts',(0.762992990878774,-1.,-1.95015342590025));
#23528=CARTESIAN_POINT('Ctrl Pts',(0.76349533353858,-1.,-1.94391746617626));
#23529=CARTESIAN_POINT('Ctrl Pts',(0.763954049121393,-1.,-1.93768964875867));
#23530=CARTESIAN_POINT('Ctrl Pts',(0.764369010673889,-1.,-1.93147105496367));
#23531=CARTESIAN_POINT('Ctrl Pts',(0.764740025488189,-1.,-1.92526263537041));
#23532=CARTESIAN_POINT('Ctrl Pts',(0.765066729667095,-1.,-1.91906491634197));
#23533=CARTESIAN_POINT('Ctrl Pts',(0.765348465884739,-1.,-1.91287765805174));
#23534=CARTESIAN_POINT('Ctrl Pts',(0.765584196937936,-1.,-1.90669961402362));
#23535=CARTESIAN_POINT('Ctrl Pts',(0.765772772593395,-1.,-1.90052930393599));
#23536=CARTESIAN_POINT('Ctrl Pts',(0.765913193856979,-1.,-1.89436577771389));
#23537=CARTESIAN_POINT('Ctrl Pts',(0.76600483706209,-1.,-1.88820926433409));
#23538=CARTESIAN_POINT('Ctrl Pts',(0.766047794851868,-1.,-1.88206215302561));
#23539=CARTESIAN_POINT('Ctrl Pts',(0.766042837036759,-1.,-1.87592888967886));
#23540=CARTESIAN_POINT('Ctrl Pts',(0.765990708546111,-1.,-1.86981398314345));
#23541=CARTESIAN_POINT('Ctrl Pts',(0.765891519092557,-1.,-1.86372027063315));
#23542=CARTESIAN_POINT('Ctrl Pts',(0.765744212909305,-1.,-1.85764741390391));
#23543=CARTESIAN_POINT('Ctrl Pts',(0.765545710619023,-1.,-1.85158945130054));
#23544=CARTESIAN_POINT('Ctrl Pts',(0.765291664861971,-1.,-1.84553698875911));
#23545=CARTESIAN_POINT('Ctrl Pts',(0.764978057881687,-1.,-1.83948181064823));
#23546=CARTESIAN_POINT('Ctrl Pts',(0.764602549687845,-1.,-1.8334207722714));
#23547=CARTESIAN_POINT('Ctrl Pts',(0.764165902606055,-1.,-1.8273599120008));
#23548=CARTESIAN_POINT('Ctrl Pts',(0.763673465462854,-1.,-1.82131873145297));
#23549=CARTESIAN_POINT('Ctrl Pts',(0.763132003836783,-1.,-1.81532118405566));
#23550=CARTESIAN_POINT('Ctrl Pts',(0.762546129464036,-1.,-1.80938551463989));
#23551=CARTESIAN_POINT('Ctrl Pts',(0.761915336443515,-1.,-1.80351583877334));
#23552=CARTESIAN_POINT('Ctrl Pts',(0.761229695230359,-1.,-1.79768986997735));
#23553=CARTESIAN_POINT('Ctrl Pts',(0.760469555880425,-1.,-1.79185815610802));
#23554=CARTESIAN_POINT('Ctrl Pts',(0.759614401109868,-1.,-1.78596964884527));
#23555=CARTESIAN_POINT('Ctrl Pts',(0.75865062667738,-1.,-1.77999411220912));
#23556=CARTESIAN_POINT('Ctrl Pts',(0.757578264077238,-1.,-1.77394167108342));
#23557=CARTESIAN_POINT('Ctrl Pts',(0.756421896028403,-1.,-1.76789396003141));
#23558=CARTESIAN_POINT('Ctrl Pts',(0.755220979975262,-1.,-1.7619781724032));
#23559=CARTESIAN_POINT('Ctrl Pts',(0.75400925402848,-1.,-1.75631083600175));
#23560=CARTESIAN_POINT('Ctrl Pts',(0.752797683531377,-1.,-1.75095139468809));
#23561=CARTESIAN_POINT('Ctrl Pts',(0.751555614163629,-1.,-1.74585086852298));
#23562=CARTESIAN_POINT('Ctrl Pts',(0.75019343597954,-1.,-1.74080458266705));
#23563=CARTESIAN_POINT('Ctrl Pts',(0.748582462954854,-1.,-1.73550351679848));
#23564=CARTESIAN_POINT('Ctrl Pts',(0.746574710096436,-1.,-1.72958533647399));
#23565=CARTESIAN_POINT('Ctrl Pts',(0.744021445433764,-1.,-1.7226822991693));
#23566=CARTESIAN_POINT('Ctrl Pts',(0.740795162032087,-1.,-1.71447789751927));
#23567=CARTESIAN_POINT('Ctrl Pts',(0.736799665724771,-1.,-1.70473309006121));
#23568=CARTESIAN_POINT('Ctrl Pts',(0.731963238697195,-1.,-1.69326921975743));
#23569=CARTESIAN_POINT('Ctrl Pts',(0.726235967997433,-1.,-1.67996158455503));
#23570=CARTESIAN_POINT('Ctrl Pts',(0.719585433804282,-1.,-1.6647288055568));
#23571=CARTESIAN_POINT('Ctrl Pts',(0.711993139355394,-1.,-1.64752408832016));
#23572=CARTESIAN_POINT('Ctrl Pts',(0.705159151988319,-1.,-1.63216541664676));
#23573=CARTESIAN_POINT('Ctrl Pts',(0.699605146405088,-1.,-1.61974673472612));
#23574=CARTESIAN_POINT('Ctrl Pts',(0.695712097881194,-1.,-1.61106790958151));
#23575=CARTESIAN_POINT('Ctrl Pts',(0.693717979106306,-1.,-1.60662857109684));
#23576=CARTESIAN_POINT('',(0.892032620296855,-1.,-1.5055822144029));
#23577=CARTESIAN_POINT('Origin',(0.,-1.,0.));
#23578=CARTESIAN_POINT('',(1.23627494547115,-1.,-1.81978687191668));
#23579=CARTESIAN_POINT('Ctrl Pts',(0.892032620296855,-1.,-1.5055822144029));
#23580=CARTESIAN_POINT('Ctrl Pts',(0.894452006964543,-1.,-1.50980486806688));
#23581=CARTESIAN_POINT('Ctrl Pts',(0.89918504748351,-1.,-1.51805569590094));
#23582=CARTESIAN_POINT('Ctrl Pts',(0.905967409625651,-1.,-1.52984849887993));
#23583=CARTESIAN_POINT('Ctrl Pts',(0.914375919026456,-1.,-1.54440491149498));
#23584=CARTESIAN_POINT('Ctrl Pts',(0.923832188944341,-1.,-1.56065988578893));
#23585=CARTESIAN_POINT('Ctrl Pts',(0.932246680108685,-1.,-1.57499388382243));
#23586=CARTESIAN_POINT('Ctrl Pts',(0.939646377893399,-1.,-1.58744937487176));
#23587=CARTESIAN_POINT('Ctrl Pts',(0.946078063315257,-1.,-1.59810042043673));
#23588=CARTESIAN_POINT('Ctrl Pts',(0.951613284356035,-1.,-1.60706069896936));
#23589=CARTESIAN_POINT('Ctrl Pts',(0.95635442292067,-1.,-1.61449324337085));
#23590=CARTESIAN_POINT('Ctrl Pts',(0.960438326101728,-1.,-1.62061638140221));
#23591=CARTESIAN_POINT('Ctrl Pts',(0.964046107040535,-1.,-1.62571930670187));
#23592=CARTESIAN_POINT('Ctrl Pts',(0.967387853230345,-1.,-1.63013849959462));
#23593=CARTESIAN_POINT('Ctrl Pts',(0.970669715997509,-1.,-1.63420665729798));
#23594=CARTESIAN_POINT('Ctrl Pts',(0.974066058287418,-1.,-1.63820952658144));
#23595=CARTESIAN_POINT('Ctrl Pts',(0.977689794119416,-1.,-1.64233990826687));
#23596=CARTESIAN_POINT('Ctrl Pts',(0.981562530939489,-1.,-1.64665139190656));
#23597=CARTESIAN_POINT('Ctrl Pts',(0.98564262292082,-1.,-1.65110016612638));
#23598=CARTESIAN_POINT('Ctrl Pts',(0.989855627854164,-1.,-1.65559044289699));
#23599=CARTESIAN_POINT('Ctrl Pts',(0.994121836661305,-1.,-1.66001553809947));
#23600=CARTESIAN_POINT('Ctrl Pts',(0.998389654952757,-1.,-1.66430758030376));
#23601=CARTESIAN_POINT('Ctrl Pts',(1.00265091003727,-1.,-1.66846059277303));
#23602=CARTESIAN_POINT('Ctrl Pts',(1.00692206696414,-1.,-1.67250335383293));
#23603=CARTESIAN_POINT('Ctrl Pts',(1.01123236493511,-1.,-1.67648246776464));
#23604=CARTESIAN_POINT('Ctrl Pts',(1.01561026162773,-1.,-1.68044289894798));
#23605=CARTESIAN_POINT('Ctrl Pts',(1.02006795074201,-1.,-1.68440578021706));
#23606=CARTESIAN_POINT('Ctrl Pts',(1.02460180535255,-1.,-1.68836910178447));
#23607=CARTESIAN_POINT('Ctrl Pts',(1.02919977579147,-1.,-1.69231840863458));
#23608=CARTESIAN_POINT('Ctrl Pts',(1.03384646003588,-1.,-1.69623414782771));
#23609=CARTESIAN_POINT('Ctrl Pts',(1.03852922490789,-1.,-1.70010052930962));
#23610=CARTESIAN_POINT('Ctrl Pts',(1.04324363334554,-1.,-1.70391338707982));
#23611=CARTESIAN_POINT('Ctrl Pts',(1.04799085404995,-1.,-1.70767646263649));
#23612=CARTESIAN_POINT('Ctrl Pts',(1.05277517202855,-1.,-1.71139783543989));
#23613=CARTESIAN_POINT('Ctrl Pts',(1.05760163192479,-1.,-1.7150865442702));
#23614=CARTESIAN_POINT('Ctrl Pts',(1.06247324680647,-1.,-1.71874858456904));
#23615=CARTESIAN_POINT('Ctrl Pts',(1.06738966975462,-1.,-1.72238500928453));
#23616=CARTESIAN_POINT('Ctrl Pts',(1.07234866990252,-1.,-1.72599406198488));
#23617=CARTESIAN_POINT('Ctrl Pts',(1.0773470373727,-1.,-1.72957248977424));
#23618=CARTESIAN_POINT('Ctrl Pts',(1.08238162784749,-1.,-1.73311705663407));
#23619=CARTESIAN_POINT('Ctrl Pts',(1.08745056285427,-1.,-1.73662628326091));
#23620=CARTESIAN_POINT('Ctrl Pts',(1.09255329056493,-1.,-1.74010053962247));
#23621=CARTESIAN_POINT('Ctrl Pts',(1.09768999241225,-1.,-1.74354119236208));
#23622=CARTESIAN_POINT('Ctrl Pts',(1.10286118991143,-1.,-1.74695004214923));
#23623=CARTESIAN_POINT('Ctrl Pts',(1.10806728183007,-1.,-1.7503286607592));
#23624=CARTESIAN_POINT('Ctrl Pts',(1.11330807582551,-1.,-1.7536777209463));
#23625=CARTESIAN_POINT('Ctrl Pts',(1.11858293216763,-1.,-1.75699720772105));
#23626=CARTESIAN_POINT('Ctrl Pts',(1.12389096855086,-1.,-1.76028671825096));
#23627=CARTESIAN_POINT('Ctrl Pts',(1.12923123555075,-1.,-1.7635457196617));
#23628=CARTESIAN_POINT('Ctrl Pts',(1.1346029180462,-1.,-1.76677384551862));
#23629=CARTESIAN_POINT('Ctrl Pts',(1.14000548336975,-1.,-1.76997111386769));
#23630=CARTESIAN_POINT('Ctrl Pts',(1.1454385822692,-1.,-1.77313777896194));
#23631=CARTESIAN_POINT('Ctrl Pts',(1.15090197841514,-1.,-1.7762742255701));
#23632=CARTESIAN_POINT('Ctrl Pts',(1.15639547194698,-1.,-1.77938085564275));
#23633=CARTESIAN_POINT('Ctrl Pts',(1.16191881298499,-1.,-1.78245795881009));
#23634=CARTESIAN_POINT('Ctrl Pts',(1.16747166312303,-1.,-1.78550566040443));
#23635=CARTESIAN_POINT('Ctrl Pts',(1.17305363177328,-1.,-1.78852398877617));
#23636=CARTESIAN_POINT('Ctrl Pts',(1.17866429440809,-1.,-1.79151291552689));
#23637=CARTESIAN_POINT('Ctrl Pts',(1.18430321697432,-1.,-1.79447240321515));
#23638=CARTESIAN_POINT('Ctrl Pts',(1.18996997934445,-1.,-1.79740245923478));
#23639=CARTESIAN_POINT('Ctrl Pts',(1.19566418930242,-1.,-1.80030314369879));
#23640=CARTESIAN_POINT('Ctrl Pts',(1.20138548938974,-1.,-1.80317454838603));
#23641=CARTESIAN_POINT('Ctrl Pts',(1.20713356605475,-1.,-1.80601678480707));
#23642=CARTESIAN_POINT('Ctrl Pts',(1.21290815708314,-1.,-1.80882996917129));
#23643=CARTESIAN_POINT('Ctrl Pts',(1.21870906103557,-1.,-1.81161420806656));
#23644=CARTESIAN_POINT('Ctrl Pts',(1.2245361330495,-1.,-1.81436959210434));
#23645=CARTESIAN_POINT('Ctrl Pts',(1.2292186489137,-1.,-1.8165508718364));
#23646=CARTESIAN_POINT('Ctrl Pts',(1.2327422452705,-1.,-1.81817389921279));
#23647=CARTESIAN_POINT('Ctrl Pts',(1.23509651170476,-1.,-1.81925017193666));
#23648=CARTESIAN_POINT('Ctrl Pts',(1.23627494547115,-1.,-1.81978687191668));
#23649=CARTESIAN_POINT('',(1.34869019493419,-1.,-1.73811241238545));
#23650=CARTESIAN_POINT('',(1.23627494547115,-1.,-1.81978687191668));
#23651=CARTESIAN_POINT('',(1.15624053661742,-1.,-1.31362392696032));
#23652=CARTESIAN_POINT('Ctrl Pts',(1.34869019493419,-1.,-1.73811241238545));
#23653=CARTESIAN_POINT('Ctrl Pts',(1.34854391898045,-1.,-1.73682580585691));
#23654=CARTESIAN_POINT('Ctrl Pts',(1.34824783112887,-1.,-1.73425417885907));
#23655=CARTESIAN_POINT('Ctrl Pts',(1.34779309152035,-1.,-1.7304014965394));
#23656=CARTESIAN_POINT('Ctrl Pts',(1.34716554819527,-1.,-1.72527410680674));
#23657=CARTESIAN_POINT('Ctrl Pts',(1.34634568653227,-1.,-1.7188807715049));
#23658=CARTESIAN_POINT('Ctrl Pts',(1.34549029589416,-1.,-1.71250340686822));
#23659=CARTESIAN_POINT('Ctrl Pts',(1.34459924533831,-1.,-1.70614212266738));
#23660=CARTESIAN_POINT('Ctrl Pts',(1.34367237124483,-1.,-1.69979707754427));
#23661=CARTESIAN_POINT('Ctrl Pts',(1.34270948206319,-1.,-1.6934684849687));
#23662=CARTESIAN_POINT('Ctrl Pts',(1.341710374848,-1.,-1.68715660868764));
#23663=CARTESIAN_POINT('Ctrl Pts',(1.34067485185203,-1.,-1.68086176030362));
#23664=CARTESIAN_POINT('Ctrl Pts',(1.3396027347034,-1.,-1.67458429426086));
#23665=CARTESIAN_POINT('Ctrl Pts',(1.33849388654388,-1.,-1.66832460783989));
#23666=CARTESIAN_POINT('Ctrl Pts',(1.33734820885262,-1.,-1.66208312541983));
#23667=CARTESIAN_POINT('Ctrl Pts',(1.33616559745172,-1.,-1.65586025952593));
#23668=CARTESIAN_POINT('Ctrl Pts',(1.33494590467993,-1.,-1.6496563728683));
#23669=CARTESIAN_POINT('Ctrl Pts',(1.33368890676572,-1.,-1.6434717485603));
#23670=CARTESIAN_POINT('Ctrl Pts',(1.33239425103724,-1.,-1.63730653475089));
#23671=CARTESIAN_POINT('Ctrl Pts',(1.33106149345645,-1.,-1.63116079730923));
#23672=CARTESIAN_POINT('Ctrl Pts',(1.3296901950568,-1.,-1.62503464209797));
#23673=CARTESIAN_POINT('Ctrl Pts',(1.32828000610449,-1.,-1.61892832270724));
#23674=CARTESIAN_POINT('Ctrl Pts',(1.32683074483356,-1.,-1.6128423401575));
#23675=CARTESIAN_POINT('Ctrl Pts',(1.32534250785782,-1.,-1.60677758290954));
#23676=CARTESIAN_POINT('Ctrl Pts',(1.32381550858256,-1.,-1.60073511858687));
#23677=CARTESIAN_POINT('Ctrl Pts',(1.32224985747682,-1.,-1.59471591079403));
#23678=CARTESIAN_POINT('Ctrl Pts',(1.32064537110892,-1.,-1.58872057258245));
#23679=CARTESIAN_POINT('Ctrl Pts',(1.31900135021432,-1.,-1.58274907898834));
#23680=CARTESIAN_POINT('Ctrl Pts',(1.31731642317187,-1.,-1.5768005650559));
#23681=CARTESIAN_POINT('Ctrl Pts',(1.31558903860016,-1.,-1.57087397835723));
#23682=CARTESIAN_POINT('Ctrl Pts',(1.31381795281002,-1.,-1.56496872402353));
#23683=CARTESIAN_POINT('Ctrl Pts',(1.31200264341696,-1.,-1.55908521254821));
#23684=CARTESIAN_POINT('Ctrl Pts',(1.31014393684222,-1.,-1.55322568759481));
#23685=CARTESIAN_POINT('Ctrl Pts',(1.30824393907473,-1.,-1.54739413957185));
#23686=CARTESIAN_POINT('Ctrl Pts',(1.30630475189556,-1.,-1.54159462645432));
#23687=CARTESIAN_POINT('Ctrl Pts',(1.30432735639489,-1.,-1.53582981268977));
#23688=CARTESIAN_POINT('Ctrl Pts',(1.30231064395568,-1.,-1.53009970283891));
#23689=CARTESIAN_POINT('Ctrl Pts',(1.30024984366328,-1.,-1.52439957861062));
#23690=CARTESIAN_POINT('Ctrl Pts',(1.29813791800747,-1.,-1.51872184912724));
#23691=CARTESIAN_POINT('Ctrl Pts',(1.29596850710509,-1.,-1.51305994241402));
#23692=CARTESIAN_POINT('Ctrl Pts',(1.29373841372842,-1.,-1.50741159078365));
#23693=CARTESIAN_POINT('Ctrl Pts',(1.29145022885181,-1.,-1.50178230149776));
#23694=CARTESIAN_POINT('Ctrl Pts',(1.28911506584254,-1.,-1.49618896881754));
#23695=CARTESIAN_POINT('Ctrl Pts',(1.2867467611644,-1.,-1.4906522831278));
#23696=CARTESIAN_POINT('Ctrl Pts',(1.28435533880201,-1.,-1.4851881711891));
#23697=CARTESIAN_POINT('Ctrl Pts',(1.28194158939517,-1.,-1.47980070347096));
#23698=CARTESIAN_POINT('Ctrl Pts',(1.2794891824849,-1.,-1.4744717526707));
#23699=CARTESIAN_POINT('Ctrl Pts',(1.27696414831089,-1.,-1.46916035917133));
#23700=CARTESIAN_POINT('Ctrl Pts',(1.27433119897822,-1.,-1.46382431332476));
#23701=CARTESIAN_POINT('Ctrl Pts',(1.27156805265289,-1.,-1.45843906294697));
#23702=CARTESIAN_POINT('Ctrl Pts',(1.2686778680489,-1.,-1.45301422764247));
#23703=CARTESIAN_POINT('Ctrl Pts',(1.26570925118868,-1.,-1.44761985001662));
#23704=CARTESIAN_POINT('Ctrl Pts',(1.26273903323858,-1.,-1.44236470511303));
#23705=CARTESIAN_POINT('Ctrl Pts',(1.25983531012005,-1.,-1.43734919180848));
#23706=CARTESIAN_POINT('Ctrl Pts',(1.25702687965755,-1.,-1.43262645609691));
#23707=CARTESIAN_POINT('Ctrl Pts',(1.25426945222639,-1.,-1.42815938799387));
#23708=CARTESIAN_POINT('Ctrl Pts',(1.2514145557001,-1.,-1.42378102115575));
#23709=CARTESIAN_POINT('Ctrl Pts',(1.24824430986571,-1.,-1.41923722596025));
#23710=CARTESIAN_POINT('Ctrl Pts',(1.24450600513056,-1.,-1.41422913175179));
#23711=CARTESIAN_POINT('Ctrl Pts',(1.23994455029534,-1.,-1.40845295531283));
#23712=CARTESIAN_POINT('Ctrl Pts',(1.23434087290423,-1.,-1.40164708206106));
#23713=CARTESIAN_POINT('Ctrl Pts',(1.22752961899387,-1.,-1.39361389568796));
#23714=CARTESIAN_POINT('Ctrl Pts',(1.21938737280852,-1.,-1.38420564527715));
#23715=CARTESIAN_POINT('Ctrl Pts',(1.20982812925645,-1.,-1.37331915607905));
#23716=CARTESIAN_POINT('Ctrl Pts',(1.1987959077932,-1.,-1.36088705043885));
#23717=CARTESIAN_POINT('Ctrl Pts',(1.18625865667441,-1.,-1.34687054001093));
#23718=CARTESIAN_POINT('Ctrl Pts',(1.17501305789857,-1.,-1.33437539347008));
#23719=CARTESIAN_POINT('Ctrl Pts',(1.16589330093588,-1.,-1.32428080721772));
#23720=CARTESIAN_POINT('Ctrl Pts',(1.15950888730809,-1.,-1.31722977216397));
#23721=CARTESIAN_POINT('Ctrl Pts',(1.15624053661742,-1.,-1.31362392696032));
#23722=CARTESIAN_POINT('',(1.31362392696032,-1.,-1.15624053661742));
#23723=CARTESIAN_POINT('Origin',(0.,-1.,0.));
#23724=CARTESIAN_POINT('',(1.73811241238545,-1.,-1.34869019493419));
#23725=CARTESIAN_POINT('Ctrl Pts',(1.31362392696032,-1.,-1.15624053661742));
#23726=CARTESIAN_POINT('Ctrl Pts',(1.3172297721596,-1.,-1.15950888730433));
#23727=CARTESIAN_POINT('Ctrl Pts',(1.32428080720544,-1.,-1.16589330092532));
#23728=CARTESIAN_POINT('Ctrl Pts',(1.33437539344842,-1.,-1.17501305787994));
#23729=CARTESIAN_POINT('Ctrl Pts',(1.34687053998157,-1.,-1.18625865664915));
#23730=CARTESIAN_POINT('Ctrl Pts',(1.36088705040677,-1.,-1.1987959077656));
#23731=CARTESIAN_POINT('Ctrl Pts',(1.37331915604962,-1.,-1.20982812923113));
#23732=CARTESIAN_POINT('Ctrl Pts',(1.38420564525391,-1.,-1.21938737278853));
#23733=CARTESIAN_POINT('Ctrl Pts',(1.39361389567257,-1.,-1.22752961898063));
#23734=CARTESIAN_POINT('Ctrl Pts',(1.40164708205345,-1.,-1.23434087289768));
#23735=CARTESIAN_POINT('Ctrl Pts',(1.40845295531151,-1.,-1.23994455029421));
#23736=CARTESIAN_POINT('Ctrl Pts',(1.41422913175437,-1.,-1.24450600513278));
#23737=CARTESIAN_POINT('Ctrl Pts',(1.41923722596421,-1.,-1.24824430986911));
#23738=CARTESIAN_POINT('Ctrl Pts',(1.42378102115911,-1.,-1.25141455570299));
#23739=CARTESIAN_POINT('Ctrl Pts',(1.42815938799555,-1.,-1.25426945222783));
#23740=CARTESIAN_POINT('Ctrl Pts',(1.43262645609679,-1.,-1.25702687965744));
#23741=CARTESIAN_POINT('Ctrl Pts',(1.43734919180719,-1.,-1.25983531011894));
#23742=CARTESIAN_POINT('Ctrl Pts',(1.44236470511145,-1.,-1.26273903323723));
#23743=CARTESIAN_POINT('Ctrl Pts',(1.44761985001544,-1.,-1.26570925118767));
#23744=CARTESIAN_POINT('Ctrl Pts',(1.45301422764205,-1.,-1.26867786804854));
#23745=CARTESIAN_POINT('Ctrl Pts',(1.45843906294725,-1.,-1.27156805265312));
#23746=CARTESIAN_POINT('Ctrl Pts',(1.4638243133254,-1.,-1.27433119897877));
#23747=CARTESIAN_POINT('Ctrl Pts',(1.46916035917197,-1.,-1.27696414831144));
#23748=CARTESIAN_POINT('Ctrl Pts',(1.4744717526711,-1.,-1.27948918248524));
#23749=CARTESIAN_POINT('Ctrl Pts',(1.47980070347102,-1.,-1.28194158939522));
#23750=CARTESIAN_POINT('Ctrl Pts',(1.48518817118891,-1.,-1.28435533880184));
#23751=CARTESIAN_POINT('Ctrl Pts',(1.4906522831275,-1.,-1.28674676116415));
#23752=CARTESIAN_POINT('Ctrl Pts',(1.49618896881729,-1.,-1.28911506584232));
#23753=CARTESIAN_POINT('Ctrl Pts',(1.50178230149764,-1.,-1.29145022885171));
#23754=CARTESIAN_POINT('Ctrl Pts',(1.50741159078367,-1.,-1.29373841372843));
#23755=CARTESIAN_POINT('Ctrl Pts',(1.51305994241412,-1.,-1.29596850710518));
#23756=CARTESIAN_POINT('Ctrl Pts',(1.51872184912735,-1.,-1.29813791800757));
#23757=CARTESIAN_POINT('Ctrl Pts',(1.5243995786107,-1.,-1.30024984366334));
#23758=CARTESIAN_POINT('Ctrl Pts',(1.53009970283893,-1.,-1.3023106439557));
#23759=CARTESIAN_POINT('Ctrl Pts',(1.53582981268976,-1.,-1.30432735639487));
#23760=CARTESIAN_POINT('Ctrl Pts',(1.54159462645428,-1.,-1.30630475189553));
#23761=CARTESIAN_POINT('Ctrl Pts',(1.54739413957183,-1.,-1.30824393907471));
#23762=CARTESIAN_POINT('Ctrl Pts',(1.55322568759481,-1.,-1.31014393684221));
#23763=CARTESIAN_POINT('Ctrl Pts',(1.55908521254822,-1.,-1.31200264341696));
#23764=CARTESIAN_POINT('Ctrl Pts',(1.56496872402352,-1.,-1.31381795281002));
#23765=CARTESIAN_POINT('Ctrl Pts',(1.57087397835721,-1.,-1.31558903860015));
#23766=CARTESIAN_POINT('Ctrl Pts',(1.57680056505585,-1.,-1.31731642317183));
#23767=CARTESIAN_POINT('Ctrl Pts',(1.58274907898829,-1.,-1.31900135021428));
#23768=CARTESIAN_POINT('Ctrl Pts',(1.58872057258244,-1.,-1.32064537110891));
#23769=CARTESIAN_POINT('Ctrl Pts',(1.59471591079408,-1.,-1.32224985747686));
#23770=CARTESIAN_POINT('Ctrl Pts',(1.600735118587,-1.,-1.32381550858266));
#23771=CARTESIAN_POINT('Ctrl Pts',(1.6067775829097,-1.,-1.32534250785794));
#23772=CARTESIAN_POINT('Ctrl Pts',(1.61284234015762,-1.,-1.32683074483365));
#23773=CARTESIAN_POINT('Ctrl Pts',(1.61892832270723,-1.,-1.32828000610448));
#23774=CARTESIAN_POINT('Ctrl Pts',(1.62503464209777,-1.,-1.32969019505665));
#23775=CARTESIAN_POINT('Ctrl Pts',(1.63116079730887,-1.,-1.33106149345618));
#23776=CARTESIAN_POINT('Ctrl Pts',(1.63730653475049,-1.,-1.33239425103694));
#23777=CARTESIAN_POINT('Ctrl Pts',(1.64347174856007,-1.,-1.33368890676554));
#23778=CARTESIAN_POINT('Ctrl Pts',(1.64965637286843,-1.,-1.33494590468003));
#23779=CARTESIAN_POINT('Ctrl Pts',(1.65586025952651,-1.,-1.33616559745217));
#23780=CARTESIAN_POINT('Ctrl Pts',(1.66208312542073,-1.,-1.33734820885331));
#23781=CARTESIAN_POINT('Ctrl Pts',(1.66832460784078,-1.,-1.33849388654458));
#23782=CARTESIAN_POINT('Ctrl Pts',(1.67458429426126,-1.,-1.33960273470372));
#23783=CARTESIAN_POINT('Ctrl Pts',(1.68086176030308,-1.,-1.3406748518516));
#23784=CARTESIAN_POINT('Ctrl Pts',(1.68715660868602,-1.,-1.34171037484673));
#23785=CARTESIAN_POINT('Ctrl Pts',(1.6934684849664,-1.,-1.34270948206139));
#23786=CARTESIAN_POINT('Ctrl Pts',(1.69979707754221,-1.,-1.34367237124322));
#23787=CARTESIAN_POINT('Ctrl Pts',(1.70614212266676,-1.,-1.34459924533783));
#23788=CARTESIAN_POINT('Ctrl Pts',(1.71250340687011,-1.,-1.34549029589563));
#23789=CARTESIAN_POINT('Ctrl Pts',(1.7188807715095,-1.,-1.34634568653586));
#23790=CARTESIAN_POINT('Ctrl Pts',(1.72527410681298,-1.,-1.34716554820013));
#23791=CARTESIAN_POINT('Ctrl Pts',(1.73040149654497,-1.,-1.3477930915247));
#23792=CARTESIAN_POINT('Ctrl Pts',(1.73425417886254,-1.,-1.34824783113158));
#23793=CARTESIAN_POINT('Ctrl Pts',(1.73682580585819,-1.,-1.34854391898145));
#23794=CARTESIAN_POINT('Ctrl Pts',(1.73811241238545,-1.,-1.34869019493419));
#23795=CARTESIAN_POINT('',(1.81978687191668,-1.,-1.23627494547115));
#23796=CARTESIAN_POINT('',(1.73811241238545,-1.,-1.34869019493419));
#23797=CARTESIAN_POINT('',(1.5055822144029,-1.,-0.892032620296855));
#23798=CARTESIAN_POINT('Ctrl Pts',(1.81978687191668,-1.,-1.23627494547115));
#23799=CARTESIAN_POINT('Ctrl Pts',(1.81925017193531,-1.,-1.23509651170384));
#23800=CARTESIAN_POINT('Ctrl Pts',(1.81817389920914,-1.,-1.23274224526804));
#23801=CARTESIAN_POINT('Ctrl Pts',(1.81655087183054,-1.,-1.22921864890975));
#23802=CARTESIAN_POINT('Ctrl Pts',(1.81436959209778,-1.,-1.22453613304507));
#23803=CARTESIAN_POINT('Ctrl Pts',(1.81161420806172,-1.,-1.2187090610323));
#23804=CARTESIAN_POINT('Ctrl Pts',(1.80882996916931,-1.,-1.2129081570818));
#23805=CARTESIAN_POINT('Ctrl Pts',(1.80601678480772,-1.,-1.20713356605519));
#23806=CARTESIAN_POINT('Ctrl Pts',(1.8031745483882,-1.,-1.2013854893912));
#23807=CARTESIAN_POINT('Ctrl Pts',(1.80030314370121,-1.,-1.19566418930405));
#23808=CARTESIAN_POINT('Ctrl Pts',(1.79740245923649,-1.,-1.1899699793456));
#23809=CARTESIAN_POINT('Ctrl Pts',(1.79447240321572,-1.,-1.18430321697471));
#23810=CARTESIAN_POINT('Ctrl Pts',(1.79151291552646,-1.,-1.17866429440781));
#23811=CARTESIAN_POINT('Ctrl Pts',(1.78852398877523,-1.,-1.17305363177265));
#23812=CARTESIAN_POINT('Ctrl Pts',(1.78550566040349,-1.,-1.16747166312239));
#23813=CARTESIAN_POINT('Ctrl Pts',(1.78245795880949,-1.,-1.16191881298458));
#23814=CARTESIAN_POINT('Ctrl Pts',(1.77938085564261,-1.,-1.15639547194689));
#23815=CARTESIAN_POINT('Ctrl Pts',(1.77627422557034,-1.,-1.15090197841531));
#23816=CARTESIAN_POINT('Ctrl Pts',(1.77313777896234,-1.,-1.14543858226948));
#23817=CARTESIAN_POINT('Ctrl Pts',(1.76997111386806,-1.,-1.14000548337));
#23818=CARTESIAN_POINT('Ctrl Pts',(1.76677384551883,-1.,-1.13460291804635));
#23819=CARTESIAN_POINT('Ctrl Pts',(1.76354571966171,-1.,-1.12923123555076));
#23820=CARTESIAN_POINT('Ctrl Pts',(1.76028671825084,-1.,-1.12389096855078));
#23821=CARTESIAN_POINT('Ctrl Pts',(1.75699720772089,-1.,-1.11858293216752));
#23822=CARTESIAN_POINT('Ctrl Pts',(1.75367772094617,-1.,-1.11330807582542));
#23823=CARTESIAN_POINT('Ctrl Pts',(1.75032866075914,-1.,-1.10806728183003));
#23824=CARTESIAN_POINT('Ctrl Pts',(1.74695004214924,-1.,-1.10286118991144));
#23825=CARTESIAN_POINT('Ctrl Pts',(1.74354119236212,-1.,-1.09768999241229));
#23826=CARTESIAN_POINT('Ctrl Pts',(1.74010053962252,-1.,-1.09255329056496));
#23827=CARTESIAN_POINT('Ctrl Pts',(1.73662628326093,-1.,-1.08745056285429));
#23828=CARTESIAN_POINT('Ctrl Pts',(1.73311705663407,-1.,-1.08238162784749));
#23829=CARTESIAN_POINT('Ctrl Pts',(1.72957248977424,-1.,-1.0773470373727));
#23830=CARTESIAN_POINT('Ctrl Pts',(1.72599406198489,-1.,-1.07234866990252));
#23831=CARTESIAN_POINT('Ctrl Pts',(1.72238500928456,-1.,-1.06738966975463));
#23832=CARTESIAN_POINT('Ctrl Pts',(1.71874858456908,-1.,-1.0624732468065));
#23833=CARTESIAN_POINT('Ctrl Pts',(1.71508654427022,-1.,-1.05760163192481));
#23834=CARTESIAN_POINT('Ctrl Pts',(1.71139783543986,-1.,-1.05277517202854));
#23835=CARTESIAN_POINT('Ctrl Pts',(1.70767646263641,-1.,-1.0479908540499));
#23836=CARTESIAN_POINT('Ctrl Pts',(1.70391338707969,-1.,-1.04324363334546));
#23837=CARTESIAN_POINT('Ctrl Pts',(1.70010052930951,-1.,-1.03852922490782));
#23838=CARTESIAN_POINT('Ctrl Pts',(1.69623414782769,-1.,-1.03384646003587));
#23839=CARTESIAN_POINT('Ctrl Pts',(1.69231840863471,-1.,-1.02919977579155));
#23840=CARTESIAN_POINT('Ctrl Pts',(1.68836910178475,-1.,-1.02460180535272));
#23841=CARTESIAN_POINT('Ctrl Pts',(1.68440578021739,-1.,-1.02006795074222));
#23842=CARTESIAN_POINT('Ctrl Pts',(1.6804428989482,-1.,-1.01561026162787));
#23843=CARTESIAN_POINT('Ctrl Pts',(1.67648246776457,-1.,-1.01123236493507));
#23844=CARTESIAN_POINT('Ctrl Pts',(1.67250335383248,-1.,-1.00692206696387));
#23845=CARTESIAN_POINT('Ctrl Pts',(1.66846059277231,-1.,-1.00265091003682));
#23846=CARTESIAN_POINT('Ctrl Pts',(1.66430758030304,-1.,-0.998389654952317));
#23847=CARTESIAN_POINT('Ctrl Pts',(1.66001553809916,-1.,-0.994121836661116));
#23848=CARTESIAN_POINT('Ctrl Pts',(1.65559044289746,-1.,-0.98985562785445));
#23849=CARTESIAN_POINT('Ctrl Pts',(1.6511001661277,-1.,-0.985642622921626));
#23850=CARTESIAN_POINT('Ctrl Pts',(1.64665139190834,-1.,-0.981562530940574));
#23851=CARTESIAN_POINT('Ctrl Pts',(1.64233990826831,-1.,-0.977689794120297));
#23852=CARTESIAN_POINT('Ctrl Pts',(1.63820952658157,-1.,-0.974066058287501));
#23853=CARTESIAN_POINT('Ctrl Pts',(1.63420665729609,-1.,-0.970669715996356));
#23854=CARTESIAN_POINT('Ctrl Pts',(1.63013849959083,-1.,-0.967387853228041));
#23855=CARTESIAN_POINT('Ctrl Pts',(1.6257193066974,-1.,-0.964046107037821));
#23856=CARTESIAN_POINT('Ctrl Pts',(1.62061638139929,-1.,-0.960438326099958));
#23857=CARTESIAN_POINT('Ctrl Pts',(1.61449324337233,-1.,-0.956354422921573));
#23858=CARTESIAN_POINT('Ctrl Pts',(1.60706069897794,-1.,-0.951613284361248));
#23859=CARTESIAN_POINT('Ctrl Pts',(1.59810042045408,-1.,-0.946078063325796));
#23860=CARTESIAN_POINT('Ctrl Pts',(1.58744937489796,-1.,-0.939646377909319));
#23861=CARTESIAN_POINT('Ctrl Pts',(1.57499388385561,-1.,-0.932246680128849));
#23862=CARTESIAN_POINT('Ctrl Pts',(1.56065988582509,-1.,-0.923832188966322));
#23863=CARTESIAN_POINT('Ctrl Pts',(1.54440491152807,-1.,-0.91437591904658));
#23864=CARTESIAN_POINT('Ctrl Pts',(1.52984849890434,-1.,-0.905967409640499));
#23865=CARTESIAN_POINT('Ctrl Pts',(1.51805569591479,-1.,-0.89918504749193));
#23866=CARTESIAN_POINT('Ctrl Pts',(1.50980486807181,-1.,-0.894452006967538));
#23867=CARTESIAN_POINT('Ctrl Pts',(1.5055822144029,-1.,-0.892032620296855));
#23868=CARTESIAN_POINT('',(1.60662857109684,-1.,-0.693717979106306));
#23869=CARTESIAN_POINT('Origin',(0.,-1.,0.));
#23870=CARTESIAN_POINT('',(2.0698113262342,-1.,-0.745574324794401));
#23871=CARTESIAN_POINT('Ctrl Pts',(1.60662857109684,-1.,-0.693717979106306));
#23872=CARTESIAN_POINT('Ctrl Pts',(1.61106790957619,-1.,-0.69571209787897));
#23873=CARTESIAN_POINT('Ctrl Pts',(1.61974673471117,-1.,-0.699605146398837));
#23874=CARTESIAN_POINT('Ctrl Pts',(1.6321654166204,-1.,-0.705159151977294));
#23875=CARTESIAN_POINT('Ctrl Pts',(1.64752408828442,-1.,-0.711993139340448));
#23876=CARTESIAN_POINT('Ctrl Pts',(1.66472880551777,-1.,-0.71958543378795));
#23877=CARTESIAN_POINT('Ctrl Pts',(1.67996158451922,-1.,-0.726235967982445));
#23878=CARTESIAN_POINT('Ctrl Pts',(1.69326921972915,-1.,-0.731963238685357));
#23879=CARTESIAN_POINT('Ctrl Pts',(1.70473309004249,-1.,-0.736799665716932));
#23880=CARTESIAN_POINT('Ctrl Pts',(1.71447789751001,-1.,-0.74079516202821));
#23881=CARTESIAN_POINT('Ctrl Pts',(1.72268229916769,-1.,-0.744021445433094));
#23882=CARTESIAN_POINT('Ctrl Pts',(1.72958533647714,-1.,-0.746574710097752));
#23883=CARTESIAN_POINT('Ctrl Pts',(1.7355035168033,-1.,-0.74858246295687));
#23884=CARTESIAN_POINT('Ctrl Pts',(1.74080458267114,-1.,-0.75019343598125));
#23885=CARTESIAN_POINT('Ctrl Pts',(1.74585086852502,-1.,-0.751555614164483));
#23886=CARTESIAN_POINT('Ctrl Pts',(1.75095139468794,-1.,-0.752797683531314));
#23887=CARTESIAN_POINT('Ctrl Pts',(1.75631083600019,-1.,-0.754009254027829));
#23888=CARTESIAN_POINT('Ctrl Pts',(1.76197817240128,-1.,-0.755220979974462));
#23889=CARTESIAN_POINT('Ctrl Pts',(1.76789396002998,-1.,-0.75642189602781));
#23890=CARTESIAN_POINT('Ctrl Pts',(1.77394167108292,-1.,-0.757578264077029));
#23891=CARTESIAN_POINT('Ctrl Pts',(1.77999411220945,-1.,-0.758650626677519));
#23892=CARTESIAN_POINT('Ctrl Pts',(1.78596964884604,-1.,-0.75961440111019));
#23893=CARTESIAN_POINT('Ctrl Pts',(1.7918581561088,-1.,-0.760469555880749));
#23894=CARTESIAN_POINT('Ctrl Pts',(1.79768986997783,-1.,-0.761229695230558));
#23895=CARTESIAN_POINT('Ctrl Pts',(1.80351583877342,-1.,-0.761915336443547));
#23896=CARTESIAN_POINT('Ctrl Pts',(1.80938551463965,-1.,-0.762546129463938));
#23897=CARTESIAN_POINT('Ctrl Pts',(1.8153211840553,-1.,-0.763132003836634));
#23898=CARTESIAN_POINT('Ctrl Pts',(1.82131873145266,-1.,-0.763673465462727));
#23899=CARTESIAN_POINT('Ctrl Pts',(1.82735991200065,-1.,-0.764165902605995));
#23900=CARTESIAN_POINT('Ctrl Pts',(1.83342077227142,-1.,-0.764602549687853));
#23901=CARTESIAN_POINT('Ctrl Pts',(1.83948181064835,-1.,-0.764978057881738));
#23902=CARTESIAN_POINT('Ctrl Pts',(1.84553698875924,-1.,-0.765291664862029));
#23903=CARTESIAN_POINT('Ctrl Pts',(1.85158945130063,-1.,-0.765545710619063));
#23904=CARTESIAN_POINT('Ctrl Pts',(1.85764741390394,-1.,-0.765744212909319));
#23905=CARTESIAN_POINT('Ctrl Pts',(1.86372027063312,-1.,-0.765891519092547));
#23906=CARTESIAN_POINT('Ctrl Pts',(1.86981398314341,-1.,-0.765990708546091));
#23907=CARTESIAN_POINT('Ctrl Pts',(1.87592888967883,-1.,-0.766042837036744));
#23908=CARTESIAN_POINT('Ctrl Pts',(1.88206215302561,-1.,-0.766047794851865));
#23909=CARTESIAN_POINT('Ctrl Pts',(1.88820926433409,-1.,-0.766004837062091));
#23910=CARTESIAN_POINT('Ctrl Pts',(1.89436577771388,-1.,-0.765913193856978));
#23911=CARTESIAN_POINT('Ctrl Pts',(1.90052930393596,-1.,-0.765772772593386));
#23912=CARTESIAN_POINT('Ctrl Pts',(1.90669961402356,-1.,-0.765584196937919));
#23913=CARTESIAN_POINT('Ctrl Pts',(1.91287765805169,-1.,-0.765348465884722));
#23914=CARTESIAN_POINT('Ctrl Pts',(1.91906491634196,-1.,-0.765066729667089));
#23915=CARTESIAN_POINT('Ctrl Pts',(1.92526263537048,-1.,-0.764740025488212));
#23916=CARTESIAN_POINT('Ctrl Pts',(1.93147105496382,-1.,-0.764369010673941));
#23917=CARTESIAN_POINT('Ctrl Pts',(1.93768964875886,-1.,-0.763954049121459));
#23918=CARTESIAN_POINT('Ctrl Pts',(1.9439174661764,-1.,-0.763495333538629));
#23919=CARTESIAN_POINT('Ctrl Pts',(1.95015342590024,-1.,-0.762992990878769));
#23920=CARTESIAN_POINT('Ctrl Pts',(1.95639665309869,-1.,-0.762447203806179));
#23921=CARTESIAN_POINT('Ctrl Pts',(1.96264672744186,-1.,-0.761858300014424));
#23922=CARTESIAN_POINT('Ctrl Pts',(1.96890351582499,-1.,-0.761226690483821));
#23923=CARTESIAN_POINT('Ctrl Pts',(1.97516705321494,-1.,-0.760552825409757));
#23924=CARTESIAN_POINT('Ctrl Pts',(1.98143741418172,-1.,-0.75983714745219));
#23925=CARTESIAN_POINT('Ctrl Pts',(1.98771456680874,-1.,-0.759080037802488));
#23926=CARTESIAN_POINT('Ctrl Pts',(1.99399831098817,-1.,-0.758281796766761));
#23927=CARTESIAN_POINT('Ctrl Pts',(2.00028834739178,-1.,-0.757442676862724));
#23928=CARTESIAN_POINT('Ctrl Pts',(2.0065843158773,-1.,-0.756562904646671));
#23929=CARTESIAN_POINT('Ctrl Pts',(2.01288584328084,-1.,-0.755642704957865));
#23930=CARTESIAN_POINT('Ctrl Pts',(2.01919259405809,-1.,-0.754682330722816));
#23931=CARTESIAN_POINT('Ctrl Pts',(2.02550428623313,-1.,-0.753682061112768));
#23932=CARTESIAN_POINT('Ctrl Pts',(2.03182068456221,-1.,-0.752642180487211));
#23933=CARTESIAN_POINT('Ctrl Pts',(2.03814160092099,-1.,-0.751562963361115));
#23934=CARTESIAN_POINT('Ctrl Pts',(2.04446689147979,-1.,-0.750444657875576));
#23935=CARTESIAN_POINT('Ctrl Pts',(2.05079645592154,-1.,-0.749287468665046));
#23936=CARTESIAN_POINT('Ctrl Pts',(2.05713023031006,-1.,-0.748091554183803));
#23937=CARTESIAN_POINT('Ctrl Pts',(2.06220058927826,-1.,-0.74710393278792));
#23938=CARTESIAN_POINT('Ctrl Pts',(2.06600523016815,-1.,-0.746345871544201));
#23939=CARTESIAN_POINT('Ctrl Pts',(2.06854248895728,-1.,-0.745832791378367));
#23940=CARTESIAN_POINT('Ctrl Pts',(2.0698113262342,-1.,-0.745574324794401));
#23941=CARTESIAN_POINT('',(2.11275013067528,-1.,-0.61342227326009));
#23942=CARTESIAN_POINT('',(2.0698113262342,-1.,-0.745574324794401));
#23943=CARTESIAN_POINT('',(1.7075470150345,-1.,-0.383122945602004));
#23944=CARTESIAN_POINT('Ctrl Pts',(2.11275013067528,-1.,-0.61342227326009));
#23945=CARTESIAN_POINT('Ctrl Pts',(2.11187554259986,-1.,-0.6124673655618));
#23946=CARTESIAN_POINT('Ctrl Pts',(2.11012443807238,-1.,-0.610560911689899));
#23947=CARTESIAN_POINT('Ctrl Pts',(2.1074919961518,-1.,-0.607711315454876));
#23948=CARTESIAN_POINT('Ctrl Pts',(2.10397049886949,-1.,-0.60393203073603));
#23949=CARTESIAN_POINT('Ctrl Pts',(2.0995493086477,-1.,-0.599241616420534));
#23950=CARTESIAN_POINT('Ctrl Pts',(2.0951087622027,-1.,-0.594585006052162));
#23951=CARTESIAN_POINT('Ctrl Pts',(2.09064881812129,-1.,-0.589962365403406));
#23952=CARTESIAN_POINT('Ctrl Pts',(2.08616943727951,-1.,-0.585373918991617));
#23953=CARTESIAN_POINT('Ctrl Pts',(2.08167059018418,-1.,-0.580819952108064));
#23954=CARTESIAN_POINT('Ctrl Pts',(2.07715226767559,-1.,-0.576300797416845));
#23955=CARTESIAN_POINT('Ctrl Pts',(2.07261449292824,-1.,-0.571816823242603));
#23956=CARTESIAN_POINT('Ctrl Pts',(2.06805732997334,-1.,-0.567368421181087));
#23957=CARTESIAN_POINT('Ctrl Pts',(2.06348090160589,-1.,-0.562955993082262));
#23958=CARTESIAN_POINT('Ctrl Pts',(2.05888537756462,-1.,-0.558579940185152));
#23959=CARTESIAN_POINT('Ctrl Pts',(2.05427091604413,-1.,-0.554240657463906));
#23960=CARTESIAN_POINT('Ctrl Pts',(2.04963761077958,-1.,-0.549938525150295));
#23961=CARTESIAN_POINT('Ctrl Pts',(2.04498544714588,-1.,-0.54567390381743));
#23962=CARTESIAN_POINT('Ctrl Pts',(2.04031422690527,-1.,-0.541447120615659));
#23963=CARTESIAN_POINT('Ctrl Pts',(2.03562362954037,-1.,-0.537258489833262));
#23964=CARTESIAN_POINT('Ctrl Pts',(2.03091336214426,-1.,-0.533108355132977));
#23965=CARTESIAN_POINT('Ctrl Pts',(2.0261832908329,-1.,-0.528997127241914));
#23966=CARTESIAN_POINT('Ctrl Pts',(2.02143356304698,-1.,-0.524925318333476));
#23967=CARTESIAN_POINT('Ctrl Pts',(2.01666477917286,-1.,-0.520893590399371));
#23968=CARTESIAN_POINT('Ctrl Pts',(2.01187773939242,-1.,-0.516902681728687));
#23969=CARTESIAN_POINT('Ctrl Pts',(2.00707309946949,-1.,-0.512953306961793));
#23970=CARTESIAN_POINT('Ctrl Pts',(2.00225107134734,-1.,-0.509046069886157));
#23971=CARTESIAN_POINT('Ctrl Pts',(1.99741107463572,-1.,-0.505181361323026));
#23972=CARTESIAN_POINT('Ctrl Pts',(1.99255149126155,-1.,-0.501359287727146));
#23973=CARTESIAN_POINT('Ctrl Pts',(1.98767044752932,-1.,-0.497579909545574));
#23974=CARTESIAN_POINT('Ctrl Pts',(1.98276658761821,-1.,-0.493843476541495));
#23975=CARTESIAN_POINT('Ctrl Pts',(1.97783973019229,-1.,-0.490150627860953));
#23976=CARTESIAN_POINT('Ctrl Pts',(1.97289186263272,-1.,-0.486502692907659));
#23977=CARTESIAN_POINT('Ctrl Pts',(1.96792703422362,-1.,-0.482901662120691));
#23978=CARTESIAN_POINT('Ctrl Pts',(1.96294933055943,-1.,-0.479349583074855));
#23979=CARTESIAN_POINT('Ctrl Pts',(1.95796111148177,-1.,-0.475848034683176));
#23980=CARTESIAN_POINT('Ctrl Pts',(1.95296148278133,-1.,-0.472397672264072));
#23981=CARTESIAN_POINT('Ctrl Pts',(1.94794381136514,-1.,-0.468997482913135));
#23982=CARTESIAN_POINT('Ctrl Pts',(1.9428979419619,-1.,-0.46564546202603));
#23983=CARTESIAN_POINT('Ctrl Pts',(1.93781486640821,-1.,-0.462340031009057));
#23984=CARTESIAN_POINT('Ctrl Pts',(1.93269066517934,-1.,-0.459081234547926));
#23985=CARTESIAN_POINT('Ctrl Pts',(1.92753067150476,-1.,-0.455872005174371));
#23986=CARTESIAN_POINT('Ctrl Pts',(1.92235380648502,-1.,-0.452719478359433));
#23987=CARTESIAN_POINT('Ctrl Pts',(1.91718342555755,-1.,-0.449632260106662));
#23988=CARTESIAN_POINT('Ctrl Pts',(1.9120369998112,-1.,-0.446617343485711));
#23989=CARTESIAN_POINT('Ctrl Pts',(1.90691756144898,-1.,-0.443677556849151));
#23990=CARTESIAN_POINT('Ctrl Pts',(1.90180124389086,-1.,-0.440807833704038));
#23991=CARTESIAN_POINT('Ctrl Pts',(1.89663648956466,-1.,-0.437995003948244));
#23992=CARTESIAN_POINT('Ctrl Pts',(1.89136993975504,-1.,-0.435225660963383));
#23993=CARTESIAN_POINT('Ctrl Pts',(1.88596913666793,-1.,-0.432493038548748));
#23994=CARTESIAN_POINT('Ctrl Pts',(1.88044229001832,-1.,-0.429803062482345));
#23995=CARTESIAN_POINT('Ctrl Pts',(1.87486989291484,-1.,-0.427183828519102));
#23996=CARTESIAN_POINT('Ctrl Pts',(1.86937803944323,-1.,-0.424678177291359));
#23997=CARTESIAN_POINT('Ctrl Pts',(1.86408083334028,-1.,-0.422327307418275));
#23998=CARTESIAN_POINT('Ctrl Pts',(1.85903281096686,-1.,-0.42015728797562));
#23999=CARTESIAN_POINT('Ctrl Pts',(1.85417632856234,-1.,-0.418164129143534));
#24000=CARTESIAN_POINT('Ctrl Pts',(1.84929312929882,-1.,-0.416300022038864));
#24001=CARTESIAN_POINT('Ctrl Pts',(1.8440575707371,-1.,-0.41448743825434));
#24002=CARTESIAN_POINT('Ctrl Pts',(1.83808953475839,-1.,-0.412633125322162));
#24003=CARTESIAN_POINT('Ctrl Pts',(1.83100408895216,-1.,-0.410641256301675));
#24004=CARTESIAN_POINT('Ctrl Pts',(1.8224702267854,-1.,-0.408428948108534));
#24005=CARTESIAN_POINT('Ctrl Pts',(1.81223801813988,-1.,-0.405933518411838));
#24006=CARTESIAN_POINT('Ctrl Pts',(1.80012077176221,-1.,-0.403107976170441));
#24007=CARTESIAN_POINT('Ctrl Pts',(1.78598826347533,-1.,-0.399919403783081));
#24008=CARTESIAN_POINT('Ctrl Pts',(1.7697556004756,-1.,-0.39634619612042));
#24009=CARTESIAN_POINT('Ctrl Pts',(1.75137405313962,-1.,-0.392375812294307));
#24010=CARTESIAN_POINT('Ctrl Pts',(1.7349317097561,-1.,-0.388877023509192));
#24011=CARTESIAN_POINT('Ctrl Pts',(1.72162022246158,-1.,-0.38607079032701));
#24012=CARTESIAN_POINT('Ctrl Pts',(1.71231062891958,-1.,-0.384119047315542));
#24013=CARTESIAN_POINT('Ctrl Pts',(1.7075470150345,-1.,-0.383122945602004));
#24014=CARTESIAN_POINT('',(1.74236521665491,-1.,-0.163289472382896));
#24015=CARTESIAN_POINT('Origin',(0.,-1.,0.));
#24016=CARTESIAN_POINT('',(2.19890268624765,-1.,-0.0694764450219582));
#24017=CARTESIAN_POINT('Ctrl Pts',(1.74236521665491,-1.,-0.163289472382896));
#24018=CARTESIAN_POINT('Ctrl Pts',(1.7472034950333,-1.,-0.163814161002002));
#24019=CARTESIAN_POINT('Ctrl Pts',(1.75666056638427,-1.,-0.164834765707159));
#24020=CARTESIAN_POINT('Ctrl Pts',(1.77018771684844,-1.,-0.1662793551464));
#24021=CARTESIAN_POINT('Ctrl Pts',(1.7869064998507,-1.,-0.168032772805197));
#24022=CARTESIAN_POINT('Ctrl Pts',(1.80561530629706,-1.,-0.169936923904608));
#24023=CARTESIAN_POINT('Ctrl Pts',(1.82215766811545,-1.,-0.171554770204119));
#24024=CARTESIAN_POINT('Ctrl Pts',(1.83658380527692,-1.,-0.1728894428919));
#24025=CARTESIAN_POINT('Ctrl Pts',(1.8489811319852,-1.,-0.173946627587732));
#24026=CARTESIAN_POINT('Ctrl Pts',(1.85948367088837,-1.,-0.17473525927603));
#24027=CARTESIAN_POINT('Ctrl Pts',(1.86828349694799,-1.,-0.175268337590758));
#24028=CARTESIAN_POINT('Ctrl Pts',(1.87563767773588,-1.,-0.175563480746485));
#24029=CARTESIAN_POINT('Ctrl Pts',(1.88188663145367,-1.,-0.175644148889699));
#24030=CARTESIAN_POINT('Ctrl Pts',(1.88742606273259,-1.,-0.175538155840648));
#24031=CARTESIAN_POINT('Ctrl Pts',(1.892646301985,-1.,-0.175274276190844));
#24032=CARTESIAN_POINT('Ctrl Pts',(1.89788101117132,-1.,-0.174879405091263));
#24033=CARTESIAN_POINT('Ctrl Pts',(1.90335253862834,-1.,-0.174375518661085));
#24034=CARTESIAN_POINT('Ctrl Pts',(1.90911693975267,-1.,-0.173776635257817));
#24035=CARTESIAN_POINT('Ctrl Pts',(1.91511429159527,-1.,-0.173090695383496));
#24036=CARTESIAN_POINT('Ctrl Pts',(1.9212233439798,-1.,-0.172321621259514));
#24037=CARTESIAN_POINT('Ctrl Pts',(1.92731093582036,-1.,-0.171471191532988));
#24038=CARTESIAN_POINT('Ctrl Pts',(1.93329183155539,-1.,-0.170541253116202));
#24039=CARTESIAN_POINT('Ctrl Pts',(1.93915639211581,-1.,-0.169534904817491));
#24040=CARTESIAN_POINT('Ctrl Pts',(1.94493757756931,-1.,-0.168455741607556));
#24041=CARTESIAN_POINT('Ctrl Pts',(1.95069027794294,-1.,-0.167307501784476));
#24042=CARTESIAN_POINT('Ctrl Pts',(1.9564675971873,-1.,-0.166093592002813));
#24043=CARTESIAN_POINT('Ctrl Pts',(1.96229379940136,-1.,-0.164816568920269));
#24044=CARTESIAN_POINT('Ctrl Pts',(1.96816512677967,-1.,-0.163478185457734));
#24045=CARTESIAN_POINT('Ctrl Pts',(1.97406280235188,-1.,-0.162079693556289));
#24046=CARTESIAN_POINT('Ctrl Pts',(1.97996195437559,-1.,-0.160622060784611));
#24047=CARTESIAN_POINT('Ctrl Pts',(1.98584238283292,-1.,-0.159106226437299));
#24048=CARTESIAN_POINT('Ctrl Pts',(1.99169810931908,-1.,-0.157533331459227));
#24049=CARTESIAN_POINT('Ctrl Pts',(1.99753284771497,-1.,-0.155904629548784));
#24050=CARTESIAN_POINT('Ctrl Pts',(2.00335565310543,-1.,-0.154221403049722));
#24051=CARTESIAN_POINT('Ctrl Pts',(2.00917680318424,-1.,-0.15248488362145));
#24052=CARTESIAN_POINT('Ctrl Pts',(2.01500291940238,-1.,-0.150696157673078));
#24053=CARTESIAN_POINT('Ctrl Pts',(2.02083464969894,-1.,-0.148856124775337));
#24054=CARTESIAN_POINT('Ctrl Pts',(2.02666926182017,-1.,-0.146965557332583));
#24055=CARTESIAN_POINT('Ctrl Pts',(2.03250223739942,-1.,-0.145025140186058));
#24056=CARTESIAN_POINT('Ctrl Pts',(2.03832911025912,-1.,-0.143035515058209));
#24057=CARTESIAN_POINT('Ctrl Pts',(2.04414757947916,-1.,-0.140997332152546));
#24058=CARTESIAN_POINT('Ctrl Pts',(2.04995762001328,-1.,-0.138911255368966));
#24059=CARTESIAN_POINT('Ctrl Pts',(2.05576044414264,-1.,-0.136777941218044));
#24060=CARTESIAN_POINT('Ctrl Pts',(2.06155781517842,-1.,-0.134598026192106));
#24061=CARTESIAN_POINT('Ctrl Pts',(2.06735123910326,-1.,-0.132372111547711));
#24062=CARTESIAN_POINT('Ctrl Pts',(2.07314114713063,-1.,-0.130100748328404));
#24063=CARTESIAN_POINT('Ctrl Pts',(2.07892715110987,-1.,-0.12778444527612));
#24064=CARTESIAN_POINT('Ctrl Pts',(2.08470840653643,-1.,-0.125423679412062));
#24065=CARTESIAN_POINT('Ctrl Pts',(2.09048392424825,-1.,-0.123018905621083));
#24066=CARTESIAN_POINT('Ctrl Pts',(2.0962529286773,-1.,-0.120570567965122));
#24067=CARTESIAN_POINT('Ctrl Pts',(2.102015121329,-1.,-0.118079107988356));
#24068=CARTESIAN_POINT('Ctrl Pts',(2.10777050261309,-1.,-0.115544957687927));
#24069=CARTESIAN_POINT('Ctrl Pts',(2.11351924490306,-1.,-0.112968534419737));
#24070=CARTESIAN_POINT('Ctrl Pts',(2.11926155590865,-1.,-0.110350236135025));
#24071=CARTESIAN_POINT('Ctrl Pts',(2.12499752307,-1.,-0.10769043523109));
#24072=CARTESIAN_POINT('Ctrl Pts',(2.13072704887293,-1.,-0.10498947915274));
#24073=CARTESIAN_POINT('Ctrl Pts',(2.13644992667165,-1.,-0.102247700556101));
#24074=CARTESIAN_POINT('Ctrl Pts',(2.14216588396025,-1.,-0.0994654261990917));
#24075=CARTESIAN_POINT('Ctrl Pts',(2.14787463531795,-1.,-0.096642985230546));
#24076=CARTESIAN_POINT('Ctrl Pts',(2.1535759397817,-1.,-0.0937807218867645));
#24077=CARTESIAN_POINT('Ctrl Pts',(2.15926961544516,-1.,-0.0908789888107267));
#24078=CARTESIAN_POINT('Ctrl Pts',(2.16495552645014,-1.,-0.0879381291386924));
#24079=CARTESIAN_POINT('Ctrl Pts',(2.17063357870952,-1.,-0.0849584620835374));
#24080=CARTESIAN_POINT('Ctrl Pts',(2.176303712113,-1.,-0.0819402680872767));
#24081=CARTESIAN_POINT('Ctrl Pts',(2.18196589448887,-1.,-0.0788837727685244));
#24082=CARTESIAN_POINT('Ctrl Pts',(2.1876201139953,-1.,-0.0757891465836149));
#24083=CARTESIAN_POINT('Ctrl Pts',(2.19213712013662,-1.,-0.0732830357306726));
#24084=CARTESIAN_POINT('Ctrl Pts',(2.19552129484002,-1.,-0.0713863779526155));
#24085=CARTESIAN_POINT('Ctrl Pts',(2.19777582085423,-1.,-0.0701143536325491));
#24086=CARTESIAN_POINT('Ctrl Pts',(2.19890268624765,-1.,-0.0694764450219582));
#24087=CARTESIAN_POINT('',(2.19890268624765,-1.,0.0694764450219582));
#24088=CARTESIAN_POINT('',(2.19890268624765,-1.,-0.0694764450219582));
#24089=CARTESIAN_POINT('',(1.74236521665491,-1.,0.163289472382896));
#24090=CARTESIAN_POINT('Ctrl Pts',(2.19890268624765,-1.,0.0694764450219582));
#24091=CARTESIAN_POINT('Ctrl Pts',(2.19777582085261,-1.,0.0701143536324925));
#24092=CARTESIAN_POINT('Ctrl Pts',(2.19552129483562,-1.,0.0713863779524626));
#24093=CARTESIAN_POINT('Ctrl Pts',(2.19213712012956,-1.,0.0732830357304275));
#24094=CARTESIAN_POINT('Ctrl Pts',(2.1876201139874,-1.,0.075789146583341));
#24095=CARTESIAN_POINT('Ctrl Pts',(2.18196589448304,-1.,0.0788837727683226));
#24096=CARTESIAN_POINT('Ctrl Pts',(2.1763037121106,-1.,0.0819402680871938));
#24097=CARTESIAN_POINT('Ctrl Pts',(2.17063357871031,-1.,0.0849584620835642));
#24098=CARTESIAN_POINT('Ctrl Pts',(2.16495552645275,-1.,0.0879381291387821));
#24099=CARTESIAN_POINT('Ctrl Pts',(2.15926961544808,-1.,0.0908789888108265));
#24100=CARTESIAN_POINT('Ctrl Pts',(2.15357593978377,-1.,0.0937807218868344));
#24101=CARTESIAN_POINT('Ctrl Pts',(2.14787463531864,-1.,0.0966429852305688));
#24102=CARTESIAN_POINT('Ctrl Pts',(2.14216588395974,-1.,0.0994654261990741));
#24103=CARTESIAN_POINT('Ctrl Pts',(2.13644992667052,-1.,0.102247700556063));
#24104=CARTESIAN_POINT('Ctrl Pts',(2.1307270488718,-1.,0.104989479152703));
#24105=CARTESIAN_POINT('Ctrl Pts',(2.12499752306927,-1.,0.107690435231068));
#24106=CARTESIAN_POINT('Ctrl Pts',(2.11926155590849,-1.,0.11035023613502));
#24107=CARTESIAN_POINT('Ctrl Pts',(2.11351924490335,-1.,0.112968534419746));
#24108=CARTESIAN_POINT('Ctrl Pts',(2.10777050261359,-1.,0.11554495768794));
#24109=CARTESIAN_POINT('Ctrl Pts',(2.10201512132945,-1.,0.118079107988368));
#24110=CARTESIAN_POINT('Ctrl Pts',(2.09625292867756,-1.,0.120570567965129));
#24111=CARTESIAN_POINT('Ctrl Pts',(2.09048392424826,-1.,0.123018905621083));
#24112=CARTESIAN_POINT('Ctrl Pts',(2.08470840653628,-1.,0.125423679412058));
#24113=CARTESIAN_POINT('Ctrl Pts',(2.07892715110967,-1.,0.127784445276116));
#24114=CARTESIAN_POINT('Ctrl Pts',(2.07314114713047,-1.,0.1301007483284));
#24115=CARTESIAN_POINT('Ctrl Pts',(2.06735123910319,-1.,0.132372111547709));
#24116=CARTESIAN_POINT('Ctrl Pts',(2.06155781517844,-1.,0.134598026192107));
#24117=CARTESIAN_POINT('Ctrl Pts',(2.0557604441427,-1.,0.136777941218044));
#24118=CARTESIAN_POINT('Ctrl Pts',(2.04995762001333,-1.,0.138911255368966));
#24119=CARTESIAN_POINT('Ctrl Pts',(2.04414757947919,-1.,0.140997332152545));
#24120=CARTESIAN_POINT('Ctrl Pts',(2.03832911025913,-1.,0.143035515058208));
#24121=CARTESIAN_POINT('Ctrl Pts',(2.03250223739941,-1.,0.145025140186058));
#24122=CARTESIAN_POINT('Ctrl Pts',(2.02666926182017,-1.,0.146965557332586));
#24123=CARTESIAN_POINT('Ctrl Pts',(2.02083464969897,-1.,0.148856124775342));
#24124=CARTESIAN_POINT('Ctrl Pts',(2.01500291940243,-1.,0.150696157673084));
#24125=CARTESIAN_POINT('Ctrl Pts',(2.00917680318426,-1.,0.152484883621452));
#24126=CARTESIAN_POINT('Ctrl Pts',(2.00335565310539,-1.,0.154221403049719));
#24127=CARTESIAN_POINT('Ctrl Pts',(1.99753284771487,-1.,0.155904629548774));
#24128=CARTESIAN_POINT('Ctrl Pts',(1.99169810931893,-1.,0.157533331459215));
#24129=CARTESIAN_POINT('Ctrl Pts',(1.98584238283279,-1.,0.159106226437288));
#24130=CARTESIAN_POINT('Ctrl Pts',(1.97996195437557,-1.,0.16062206078461));
#24131=CARTESIAN_POINT('Ctrl Pts',(1.97406280235204,-1.,0.162079693556302));
#24132=CARTESIAN_POINT('Ctrl Pts',(1.96816512678,-1.,0.16347818545776));
#24133=CARTESIAN_POINT('Ctrl Pts',(1.96229379940174,-1.,0.1648165689203));
#24134=CARTESIAN_POINT('Ctrl Pts',(1.95646759718755,-1.,0.166093592002832));
#24135=CARTESIAN_POINT('Ctrl Pts',(1.95069027794286,-1.,0.167307501784469));
#24136=CARTESIAN_POINT('Ctrl Pts',(1.94493757756879,-1.,0.168455741607515));
#24137=CARTESIAN_POINT('Ctrl Pts',(1.93915639211497,-1.,0.169534904817425));
#24138=CARTESIAN_POINT('Ctrl Pts',(1.93329183155455,-1.,0.170541253116136));
#24139=CARTESIAN_POINT('Ctrl Pts',(1.92731093582,-1.,0.17147119153296));
#24140=CARTESIAN_POINT('Ctrl Pts',(1.92122334398034,-1.,0.172321621259556));
#24141=CARTESIAN_POINT('Ctrl Pts',(1.91511429159681,-1.,0.173090695383619));
#24142=CARTESIAN_POINT('Ctrl Pts',(1.90911693975475,-1.,0.173776635257983));
#24143=CARTESIAN_POINT('Ctrl Pts',(1.90335253863003,-1.,0.174375518661222));
#24144=CARTESIAN_POINT('Ctrl Pts',(1.89788101117148,-1.,0.174879405091277));
#24145=CARTESIAN_POINT('Ctrl Pts',(1.89264630198279,-1.,0.175274276190664));
#24146=CARTESIAN_POINT('Ctrl Pts',(1.88742606272818,-1.,0.175538155840286));
#24147=CARTESIAN_POINT('Ctrl Pts',(1.88188663144846,-1.,0.175644148889271));
#24148=CARTESIAN_POINT('Ctrl Pts',(1.87563767773249,-1.,0.175563480746205));
#24149=CARTESIAN_POINT('Ctrl Pts',(1.86828349694972,-1.,0.1752683375909));
#24150=CARTESIAN_POINT('Ctrl Pts',(1.85948367089838,-1.,0.174735259276856));
#24151=CARTESIAN_POINT('Ctrl Pts',(1.84898113200543,-1.,0.173946627589401));
#24152=CARTESIAN_POINT('Ctrl Pts',(1.83658380530747,-1.,0.17288944289442));
#24153=CARTESIAN_POINT('Ctrl Pts',(1.82215766815414,-1.,0.171554770207306));
#24154=CARTESIAN_POINT('Ctrl Pts',(1.80561530633924,-1.,0.169936923908078));
#24155=CARTESIAN_POINT('Ctrl Pts',(1.78690649988931,-1.,0.16803277280837));
#24156=CARTESIAN_POINT('Ctrl Pts',(1.77018771687692,-1.,0.166279355148738));
#24157=CARTESIAN_POINT('Ctrl Pts',(1.75666056640041,-1.,0.164834765708484));
#24158=CARTESIAN_POINT('Ctrl Pts',(1.74720349503904,-1.,0.163814161002474));
#24159=CARTESIAN_POINT('Ctrl Pts',(1.74236521665491,-1.,0.163289472382896));
#24160=CARTESIAN_POINT('',(1.7075470150345,-1.,0.383122945602004));
#24161=CARTESIAN_POINT('Origin',(0.,-1.,0.));
#24162=CARTESIAN_POINT('',(2.11275013067528,-1.,0.613422273260091));
#24163=CARTESIAN_POINT('Ctrl Pts',(1.7075470150345,-1.,0.383122945602004));
#24164=CARTESIAN_POINT('Ctrl Pts',(1.71231062891398,-1.,0.384119047314215));
#24165=CARTESIAN_POINT('Ctrl Pts',(1.72162022244582,-1.,0.386070790323281));
#24166=CARTESIAN_POINT('Ctrl Pts',(1.73493170972829,-1.,0.388877023502615));
#24167=CARTESIAN_POINT('Ctrl Pts',(1.75137405310193,-1.,0.392375812285396));
#24168=CARTESIAN_POINT('Ctrl Pts',(1.76975560043442,-1.,0.396346196110688));
#24169=CARTESIAN_POINT('Ctrl Pts',(1.78598826343754,-1.,0.399919403774156));
#24170=CARTESIAN_POINT('Ctrl Pts',(1.80012077173238,-1.,0.403107976163396));
#24171=CARTESIAN_POINT('Ctrl Pts',(1.81223801812013,-1.,0.405933518407176));
#24172=CARTESIAN_POINT('Ctrl Pts',(1.82247022677562,-1.,0.408428948106228));
#24173=CARTESIAN_POINT('Ctrl Pts',(1.83100408895047,-1.,0.410641256301276));
#24174=CARTESIAN_POINT('Ctrl Pts',(1.8380895347617,-1.,0.412633125322945));
#24175=CARTESIAN_POINT('Ctrl Pts',(1.84405757074218,-1.,0.414487438255542));
#24176=CARTESIAN_POINT('Ctrl Pts',(1.84929312930314,-1.,0.416300022039885));
#24177=CARTESIAN_POINT('Ctrl Pts',(1.8541763285645,-1.,0.418164129144046));
#24178=CARTESIAN_POINT('Ctrl Pts',(1.8590328109667,-1.,0.420157287975583));
#24179=CARTESIAN_POINT('Ctrl Pts',(1.86408083333863,-1.,0.422327307417885));
#24180=CARTESIAN_POINT('Ctrl Pts',(1.8693780394412,-1.,0.424678177290876));
#24181=CARTESIAN_POINT('Ctrl Pts',(1.87486989291333,-1.,0.427183828518743));
#24182=CARTESIAN_POINT('Ctrl Pts',(1.88044229001778,-1.,0.429803062482217));
#24183=CARTESIAN_POINT('Ctrl Pts',(1.88596913666828,-1.,0.432493038548833));
#24184=CARTESIAN_POINT('Ctrl Pts',(1.89136993975585,-1.,0.43522566096358));
#24185=CARTESIAN_POINT('Ctrl Pts',(1.89663648956549,-1.,0.437995003948443));
#24186=CARTESIAN_POINT('Ctrl Pts',(1.90180124389137,-1.,0.440807833704161));
#24187=CARTESIAN_POINT('Ctrl Pts',(1.90691756144906,-1.,0.443677556849171));
#24188=CARTESIAN_POINT('Ctrl Pts',(1.91203699981095,-1.,0.446617343485651));
#24189=CARTESIAN_POINT('Ctrl Pts',(1.91718342555717,-1.,0.449632260106572));
#24190=CARTESIAN_POINT('Ctrl Pts',(1.9223538064847,-1.,0.452719478359356));
#24191=CARTESIAN_POINT('Ctrl Pts',(1.92753067150461,-1.,0.455872005174336));
#24192=CARTESIAN_POINT('Ctrl Pts',(1.93269066517936,-1.,0.459081234547932));
#24193=CARTESIAN_POINT('Ctrl Pts',(1.93781486640834,-1.,0.462340031009087));
#24194=CARTESIAN_POINT('Ctrl Pts',(1.94289794196205,-1.,0.465645462026065));
#24195=CARTESIAN_POINT('Ctrl Pts',(1.94794381136524,-1.,0.468997482913158));
#24196=CARTESIAN_POINT('Ctrl Pts',(1.95296148278136,-1.,0.47239767226408));
#24197=CARTESIAN_POINT('Ctrl Pts',(1.95796111148175,-1.,0.475848034683172));
#24198=CARTESIAN_POINT('Ctrl Pts',(1.96294933055938,-1.,0.479349583074846));
#24199=CARTESIAN_POINT('Ctrl Pts',(1.96792703422358,-1.,0.482901662120687));
#24200=CARTESIAN_POINT('Ctrl Pts',(1.97289186263272,-1.,0.486502692907661));
#24201=CARTESIAN_POINT('Ctrl Pts',(1.97783973019229,-1.,0.490150627860955));
#24202=CARTESIAN_POINT('Ctrl Pts',(1.9827665876182,-1.,0.493843476541493));
#24203=CARTESIAN_POINT('Ctrl Pts',(1.98767044752929,-1.,0.497579909545564));
#24204=CARTESIAN_POINT('Ctrl Pts',(1.9925514912615,-1.,0.501359287727129));
#24205=CARTESIAN_POINT('Ctrl Pts',(1.99741107463567,-1.,0.505181361323011));
#24206=CARTESIAN_POINT('Ctrl Pts',(2.00225107134733,-1.,0.509046069886152));
#24207=CARTESIAN_POINT('Ctrl Pts',(2.00707309946955,-1.,0.512953306961814));
#24208=CARTESIAN_POINT('Ctrl Pts',(2.01187773939257,-1.,0.516902681728733));
#24209=CARTESIAN_POINT('Ctrl Pts',(2.01666477917305,-1.,0.520893590399429));
#24210=CARTESIAN_POINT('Ctrl Pts',(2.02143356304712,-1.,0.524925318333519));
#24211=CARTESIAN_POINT('Ctrl Pts',(2.02618329083289,-1.,0.528997127241911));
#24212=CARTESIAN_POINT('Ctrl Pts',(2.03091336214401,-1.,0.533108355132905));
#24213=CARTESIAN_POINT('Ctrl Pts',(2.03562362953993,-1.,0.537258489833135));
#24214=CARTESIAN_POINT('Ctrl Pts',(2.0403142269048,-1.,0.54144712061552));
#24215=CARTESIAN_POINT('Ctrl Pts',(2.0449854471456,-1.,0.545673903817349));
#24216=CARTESIAN_POINT('Ctrl Pts',(2.04963761077974,-1.,0.549938525150342));
#24217=CARTESIAN_POINT('Ctrl Pts',(2.05427091604482,-1.,0.55424065746411));
#24218=CARTESIAN_POINT('Ctrl Pts',(2.05888537756571,-1.,0.558579940185468));
#24219=CARTESIAN_POINT('Ctrl Pts',(2.06348090160697,-1.,0.562955993082574));
#24220=CARTESIAN_POINT('Ctrl Pts',(2.06805732997383,-1.,0.56736842118123));
#24221=CARTESIAN_POINT('Ctrl Pts',(2.07261449292757,-1.,0.571816823242411));
#24222=CARTESIAN_POINT('Ctrl Pts',(2.07715226767361,-1.,0.576300797416275));
#24223=CARTESIAN_POINT('Ctrl Pts',(2.08167059018138,-1.,0.580819952107257));
#24224=CARTESIAN_POINT('Ctrl Pts',(2.086169437277,-1.,0.585373918990895));
#24225=CARTESIAN_POINT('Ctrl Pts',(2.09064881812053,-1.,0.58996236540319));
#24226=CARTESIAN_POINT('Ctrl Pts',(2.09510876220501,-1.,0.594585006052824));
#24227=CARTESIAN_POINT('Ctrl Pts',(2.09954930865331,-1.,0.599241616422144));
#24228=CARTESIAN_POINT('Ctrl Pts',(2.10397049887709,-1.,0.603932030738212));
#24229=CARTESIAN_POINT('Ctrl Pts',(2.10749199615859,-1.,0.607711315456826));
#24230=CARTESIAN_POINT('Ctrl Pts',(2.11012443807661,-1.,0.610560911691114));
#24231=CARTESIAN_POINT('Ctrl Pts',(2.11187554260142,-1.,0.61246736556225));
#24232=CARTESIAN_POINT('Ctrl Pts',(2.11275013067528,-1.,0.613422273260091));
#24233=CARTESIAN_POINT('',(2.0698113262342,-1.,0.745574324794401));
#24234=CARTESIAN_POINT('',(2.11275013067528,-1.,0.613422273260091));
#24235=CARTESIAN_POINT('Ctrl Pts',(2.0698113262342,-1.,0.745574324794401));
#24236=CARTESIAN_POINT('Ctrl Pts',(2.06854248895575,-1.,0.74583279137781));
#24237=CARTESIAN_POINT('Ctrl Pts',(2.06600523016401,-1.,0.746345871542696));
#24238=CARTESIAN_POINT('Ctrl Pts',(2.06220058927162,-1.,0.747103932785504));
#24239=CARTESIAN_POINT('Ctrl Pts',(2.05713023030263,-1.,0.748091554181101));
#24240=CARTESIAN_POINT('Ctrl Pts',(2.05079645591606,-1.,0.749287468663053));
#24241=CARTESIAN_POINT('Ctrl Pts',(2.04446689147754,-1.,0.750444657874758));
#24242=CARTESIAN_POINT('Ctrl Pts',(2.03814160092173,-1.,0.751562963361384));
#24243=CARTESIAN_POINT('Ctrl Pts',(2.03182068456467,-1.,0.752642180488104));
#24244=CARTESIAN_POINT('Ctrl Pts',(2.02550428623587,-1.,0.753682061113766));
#24245=CARTESIAN_POINT('Ctrl Pts',(2.01919259406003,-1.,0.75468233072352));
#24246=CARTESIAN_POINT('Ctrl Pts',(2.01288584328149,-1.,0.755642704958101));
#24247=CARTESIAN_POINT('Ctrl Pts',(2.00658431587682,-1.,0.756562904646496));
#24248=CARTESIAN_POINT('Ctrl Pts',(2.00028834739072,-1.,0.757442676862342));
#24249=CARTESIAN_POINT('Ctrl Pts',(1.9939983109871,-1.,0.758281796766377));
#24250=CARTESIAN_POINT('Ctrl Pts',(1.98771456680806,-1.,0.759080037802243));
#24251=CARTESIAN_POINT('Ctrl Pts',(1.98143741418156,-1.,0.759837147452135));
#24252=CARTESIAN_POINT('Ctrl Pts',(1.97516705321521,-1.,0.760552825409856));
#24253=CARTESIAN_POINT('Ctrl Pts',(1.96890351582545,-1.,0.761226690483986));
#24254=CARTESIAN_POINT('Ctrl Pts',(1.96264672744229,-1.,0.761858300014575));
#24255=CARTESIAN_POINT('Ctrl Pts',(1.95639665309893,-1.,0.762447203806264));
#24256=CARTESIAN_POINT('Ctrl Pts',(1.95015342590025,-1.,0.762992990878774));
#24257=CARTESIAN_POINT('Ctrl Pts',(1.94391746617626,-1.,0.763495333538581));
#24258=CARTESIAN_POINT('Ctrl Pts',(1.93768964875867,-1.,0.763954049121394));
#24259=CARTESIAN_POINT('Ctrl Pts',(1.93147105496367,-1.,0.76436901067389));
#24260=CARTESIAN_POINT('Ctrl Pts',(1.92526263537041,-1.,0.764740025488189));
#24261=CARTESIAN_POINT('Ctrl Pts',(1.91906491634197,-1.,0.765066729667095));
#24262=CARTESIAN_POINT('Ctrl Pts',(1.91287765805174,-1.,0.765348465884739));
#24263=CARTESIAN_POINT('Ctrl Pts',(1.90669961402362,-1.,0.765584196937937));
#24264=CARTESIAN_POINT('Ctrl Pts',(1.90052930393599,-1.,0.765772772593395));
#24265=CARTESIAN_POINT('Ctrl Pts',(1.89436577771389,-1.,0.765913193856979));
#24266=CARTESIAN_POINT('Ctrl Pts',(1.88820926433409,-1.,0.76600483706209));
#24267=CARTESIAN_POINT('Ctrl Pts',(1.88206215302561,-1.,0.766047794851869));
#24268=CARTESIAN_POINT('Ctrl Pts',(1.87592888967886,-1.,0.766042837036759));
#24269=CARTESIAN_POINT('Ctrl Pts',(1.86981398314345,-1.,0.765990708546112));
#24270=CARTESIAN_POINT('Ctrl Pts',(1.86372027063314,-1.,0.765891519092557));
#24271=CARTESIAN_POINT('Ctrl Pts',(1.85764741390391,-1.,0.765744212909305));
#24272=CARTESIAN_POINT('Ctrl Pts',(1.85158945130054,-1.,0.765545710619023));
#24273=CARTESIAN_POINT('Ctrl Pts',(1.8455369887591,-1.,0.765291664861972));
#24274=CARTESIAN_POINT('Ctrl Pts',(1.83948181064823,-1.,0.764978057881688));
#24275=CARTESIAN_POINT('Ctrl Pts',(1.8334207722714,-1.,0.764602549687846));
#24276=CARTESIAN_POINT('Ctrl Pts',(1.8273599120008,-1.,0.764165902606056));
#24277=CARTESIAN_POINT('Ctrl Pts',(1.82131873145297,-1.,0.763673465462854));
#24278=CARTESIAN_POINT('Ctrl Pts',(1.81532118405566,-1.,0.763132003836783));
#24279=CARTESIAN_POINT('Ctrl Pts',(1.80938551463989,-1.,0.762546129464036));
#24280=CARTESIAN_POINT('Ctrl Pts',(1.80351583877334,-1.,0.761915336443516));
#24281=CARTESIAN_POINT('Ctrl Pts',(1.79768986997735,-1.,0.761229695230359));
#24282=CARTESIAN_POINT('Ctrl Pts',(1.79185815610802,-1.,0.760469555880425));
#24283=CARTESIAN_POINT('Ctrl Pts',(1.78596964884526,-1.,0.759614401109868));
#24284=CARTESIAN_POINT('Ctrl Pts',(1.77999411220912,-1.,0.75865062667738));
#24285=CARTESIAN_POINT('Ctrl Pts',(1.77394167108342,-1.,0.757578264077238));
#24286=CARTESIAN_POINT('Ctrl Pts',(1.76789396003141,-1.,0.756421896028403));
#24287=CARTESIAN_POINT('Ctrl Pts',(1.7619781724032,-1.,0.755220979975262));
#24288=CARTESIAN_POINT('Ctrl Pts',(1.75631083600175,-1.,0.75400925402848));
#24289=CARTESIAN_POINT('Ctrl Pts',(1.75095139468809,-1.,0.752797683531377));
#24290=CARTESIAN_POINT('Ctrl Pts',(1.74585086852298,-1.,0.751555614163629));
#24291=CARTESIAN_POINT('Ctrl Pts',(1.74080458266705,-1.,0.750193435979541));
#24292=CARTESIAN_POINT('Ctrl Pts',(1.73550351679848,-1.,0.748582462954855));
#24293=CARTESIAN_POINT('Ctrl Pts',(1.72958533647399,-1.,0.746574710096437));
#24294=CARTESIAN_POINT('Ctrl Pts',(1.7226822991693,-1.,0.744021445433765));
#24295=CARTESIAN_POINT('Ctrl Pts',(1.71447789751927,-1.,0.740795162032088));
#24296=CARTESIAN_POINT('Ctrl Pts',(1.70473309006121,-1.,0.736799665724771));
#24297=CARTESIAN_POINT('Ctrl Pts',(1.69326921975743,-1.,0.731963238697195));
#24298=CARTESIAN_POINT('Ctrl Pts',(1.67996158455503,-1.,0.726235967997433));
#24299=CARTESIAN_POINT('Ctrl Pts',(1.6647288055568,-1.,0.719585433804282));
#24300=CARTESIAN_POINT('Ctrl Pts',(1.64752408832016,-1.,0.711993139355394));
#24301=CARTESIAN_POINT('Ctrl Pts',(1.63216541664676,-1.,0.705159151988319));
#24302=CARTESIAN_POINT('Ctrl Pts',(1.61974673472612,-1.,0.699605146405088));
#24303=CARTESIAN_POINT('Ctrl Pts',(1.61106790958151,-1.,0.695712097881194));
#24304=CARTESIAN_POINT('Ctrl Pts',(1.60662857109684,-1.,0.693717979106306));
#24305=CARTESIAN_POINT('Origin',(0.,-1.,0.));
#24306=CARTESIAN_POINT('Origin',(0.,0.,0.));
#24307=CARTESIAN_POINT('Origin',(0.,2.2,0.));
#24308=CARTESIAN_POINT('Origin',(0.,1.,0.));
#24309=CARTESIAN_POINT('',(-1.4,2.2,1.71450551880629E-16));
#24310=CARTESIAN_POINT('Origin',(0.,2.2,0.));
#24311=CARTESIAN_POINT('',(-1.4,1.,1.71450551880629E-16));
#24312=CARTESIAN_POINT('',(-1.4,1.,1.71450551880629E-16));
#24313=CARTESIAN_POINT('Origin',(0.,1.,0.));
#24314=CARTESIAN_POINT('Origin',(0.,2.2,0.));
#24315=CARTESIAN_POINT('Ctrl Pts',(2.11275013067528,-1.,0.613422273260091));
#24316=CARTESIAN_POINT('Ctrl Pts',(2.11275013067528,1.,0.613422273260091));
#24317=CARTESIAN_POINT('Ctrl Pts',(2.11187554260142,-1.,0.61246736556225));
#24318=CARTESIAN_POINT('Ctrl Pts',(2.11187554260142,1.,0.61246736556225));
#24319=CARTESIAN_POINT('Ctrl Pts',(2.11012443807661,-1.,0.610560911691114));
#24320=CARTESIAN_POINT('Ctrl Pts',(2.11012443807661,1.,0.610560911691114));
#24321=CARTESIAN_POINT('Ctrl Pts',(2.10749199615859,-1.,0.607711315456826));
#24322=CARTESIAN_POINT('Ctrl Pts',(2.10749199615859,1.,0.607711315456826));
#24323=CARTESIAN_POINT('Ctrl Pts',(2.10397049887709,-1.,0.603932030738212));
#24324=CARTESIAN_POINT('Ctrl Pts',(2.10397049887709,1.,0.603932030738212));
#24325=CARTESIAN_POINT('Ctrl Pts',(2.09954930865331,-1.,0.599241616422144));
#24326=CARTESIAN_POINT('Ctrl Pts',(2.09954930865331,1.,0.599241616422144));
#24327=CARTESIAN_POINT('Ctrl Pts',(2.09510876220501,-1.,0.594585006052824));
#24328=CARTESIAN_POINT('Ctrl Pts',(2.09510876220501,1.,0.594585006052824));
#24329=CARTESIAN_POINT('Ctrl Pts',(2.09064881812053,-1.,0.58996236540319));
#24330=CARTESIAN_POINT('Ctrl Pts',(2.09064881812053,1.,0.58996236540319));
#24331=CARTESIAN_POINT('Ctrl Pts',(2.086169437277,-1.,0.585373918990895));
#24332=CARTESIAN_POINT('Ctrl Pts',(2.086169437277,1.,0.585373918990895));
#24333=CARTESIAN_POINT('Ctrl Pts',(2.08167059018138,-1.,0.580819952107257));
#24334=CARTESIAN_POINT('Ctrl Pts',(2.08167059018138,1.,0.580819952107257));
#24335=CARTESIAN_POINT('Ctrl Pts',(2.07715226767361,-1.,0.576300797416275));
#24336=CARTESIAN_POINT('Ctrl Pts',(2.07715226767361,1.,0.576300797416275));
#24337=CARTESIAN_POINT('Ctrl Pts',(2.07261449292757,-1.,0.571816823242411));
#24338=CARTESIAN_POINT('Ctrl Pts',(2.07261449292757,1.,0.571816823242411));
#24339=CARTESIAN_POINT('Ctrl Pts',(2.06805732997383,-1.,0.56736842118123));
#24340=CARTESIAN_POINT('Ctrl Pts',(2.06805732997383,1.,0.56736842118123));
#24341=CARTESIAN_POINT('Ctrl Pts',(2.06348090160697,-1.,0.562955993082574));
#24342=CARTESIAN_POINT('Ctrl Pts',(2.06348090160697,1.,0.562955993082574));
#24343=CARTESIAN_POINT('Ctrl Pts',(2.05888537756571,-1.,0.558579940185468));
#24344=CARTESIAN_POINT('Ctrl Pts',(2.05888537756571,1.,0.558579940185468));
#24345=CARTESIAN_POINT('Ctrl Pts',(2.05427091604482,-1.,0.55424065746411));
#24346=CARTESIAN_POINT('Ctrl Pts',(2.05427091604482,1.,0.55424065746411));
#24347=CARTESIAN_POINT('Ctrl Pts',(2.04963761077974,-1.,0.549938525150342));
#24348=CARTESIAN_POINT('Ctrl Pts',(2.04963761077974,1.,0.549938525150342));
#24349=CARTESIAN_POINT('Ctrl Pts',(2.0449854471456,-1.,0.545673903817349));
#24350=CARTESIAN_POINT('Ctrl Pts',(2.0449854471456,1.,0.545673903817349));
#24351=CARTESIAN_POINT('Ctrl Pts',(2.0403142269048,-1.,0.54144712061552));
#24352=CARTESIAN_POINT('Ctrl Pts',(2.0403142269048,1.,0.54144712061552));
#24353=CARTESIAN_POINT('Ctrl Pts',(2.03562362953993,-1.,0.537258489833135));
#24354=CARTESIAN_POINT('Ctrl Pts',(2.03562362953993,1.,0.537258489833135));
#24355=CARTESIAN_POINT('Ctrl Pts',(2.03091336214401,-1.,0.533108355132905));
#24356=CARTESIAN_POINT('Ctrl Pts',(2.03091336214401,1.,0.533108355132905));
#24357=CARTESIAN_POINT('Ctrl Pts',(2.02618329083289,-1.,0.528997127241911));
#24358=CARTESIAN_POINT('Ctrl Pts',(2.02618329083289,1.,0.528997127241911));
#24359=CARTESIAN_POINT('Ctrl Pts',(2.02143356304712,-1.,0.524925318333519));
#24360=CARTESIAN_POINT('Ctrl Pts',(2.02143356304712,1.,0.524925318333519));
#24361=CARTESIAN_POINT('Ctrl Pts',(2.01666477917305,-1.,0.520893590399429));
#24362=CARTESIAN_POINT('Ctrl Pts',(2.01666477917305,1.,0.520893590399429));
#24363=CARTESIAN_POINT('Ctrl Pts',(2.01187773939257,-1.,0.516902681728733));
#24364=CARTESIAN_POINT('Ctrl Pts',(2.01187773939257,1.,0.516902681728733));
#24365=CARTESIAN_POINT('Ctrl Pts',(2.00707309946955,-1.,0.512953306961814));
#24366=CARTESIAN_POINT('Ctrl Pts',(2.00707309946955,1.,0.512953306961814));
#24367=CARTESIAN_POINT('Ctrl Pts',(2.00225107134733,-1.,0.509046069886152));
#24368=CARTESIAN_POINT('Ctrl Pts',(2.00225107134733,1.,0.509046069886152));
#24369=CARTESIAN_POINT('Ctrl Pts',(1.99741107463567,-1.,0.505181361323011));
#24370=CARTESIAN_POINT('Ctrl Pts',(1.99741107463567,1.,0.505181361323011));
#24371=CARTESIAN_POINT('Ctrl Pts',(1.9925514912615,-1.,0.501359287727129));
#24372=CARTESIAN_POINT('Ctrl Pts',(1.9925514912615,1.,0.501359287727129));
#24373=CARTESIAN_POINT('Ctrl Pts',(1.98767044752929,-1.,0.497579909545564));
#24374=CARTESIAN_POINT('Ctrl Pts',(1.98767044752929,1.,0.497579909545564));
#24375=CARTESIAN_POINT('Ctrl Pts',(1.9827665876182,-1.,0.493843476541493));
#24376=CARTESIAN_POINT('Ctrl Pts',(1.9827665876182,1.,0.493843476541493));
#24377=CARTESIAN_POINT('Ctrl Pts',(1.97783973019229,-1.,0.490150627860955));
#24378=CARTESIAN_POINT('Ctrl Pts',(1.97783973019229,1.,0.490150627860955));
#24379=CARTESIAN_POINT('Ctrl Pts',(1.97289186263272,-1.,0.486502692907661));
#24380=CARTESIAN_POINT('Ctrl Pts',(1.97289186263272,1.,0.486502692907661));
#24381=CARTESIAN_POINT('Ctrl Pts',(1.96792703422358,-1.,0.482901662120687));
#24382=CARTESIAN_POINT('Ctrl Pts',(1.96792703422358,1.,0.482901662120687));
#24383=CARTESIAN_POINT('Ctrl Pts',(1.96294933055938,-1.,0.479349583074846));
#24384=CARTESIAN_POINT('Ctrl Pts',(1.96294933055938,1.,0.479349583074846));
#24385=CARTESIAN_POINT('Ctrl Pts',(1.95796111148175,-1.,0.475848034683172));
#24386=CARTESIAN_POINT('Ctrl Pts',(1.95796111148175,1.,0.475848034683172));
#24387=CARTESIAN_POINT('Ctrl Pts',(1.95296148278136,-1.,0.47239767226408));
#24388=CARTESIAN_POINT('Ctrl Pts',(1.95296148278136,1.,0.47239767226408));
#24389=CARTESIAN_POINT('Ctrl Pts',(1.94794381136524,-1.,0.468997482913158));
#24390=CARTESIAN_POINT('Ctrl Pts',(1.94794381136524,1.,0.468997482913158));
#24391=CARTESIAN_POINT('Ctrl Pts',(1.94289794196205,-1.,0.465645462026065));
#24392=CARTESIAN_POINT('Ctrl Pts',(1.94289794196205,1.,0.465645462026065));
#24393=CARTESIAN_POINT('Ctrl Pts',(1.93781486640834,-1.,0.462340031009087));
#24394=CARTESIAN_POINT('Ctrl Pts',(1.93781486640834,1.,0.462340031009087));
#24395=CARTESIAN_POINT('Ctrl Pts',(1.93269066517936,-1.,0.459081234547932));
#24396=CARTESIAN_POINT('Ctrl Pts',(1.93269066517936,1.,0.459081234547932));
#24397=CARTESIAN_POINT('Ctrl Pts',(1.92753067150461,-1.,0.455872005174336));
#24398=CARTESIAN_POINT('Ctrl Pts',(1.92753067150461,1.,0.455872005174336));
#24399=CARTESIAN_POINT('Ctrl Pts',(1.9223538064847,-1.,0.452719478359356));
#24400=CARTESIAN_POINT('Ctrl Pts',(1.9223538064847,1.,0.452719478359356));
#24401=CARTESIAN_POINT('Ctrl Pts',(1.91718342555717,-1.,0.449632260106572));
#24402=CARTESIAN_POINT('Ctrl Pts',(1.91718342555717,1.,0.449632260106572));
#24403=CARTESIAN_POINT('Ctrl Pts',(1.91203699981095,-1.,0.446617343485651));
#24404=CARTESIAN_POINT('Ctrl Pts',(1.91203699981095,1.,0.446617343485651));
#24405=CARTESIAN_POINT('Ctrl Pts',(1.90691756144906,-1.,0.443677556849171));
#24406=CARTESIAN_POINT('Ctrl Pts',(1.90691756144906,1.,0.443677556849171));
#24407=CARTESIAN_POINT('Ctrl Pts',(1.90180124389137,-1.,0.440807833704161));
#24408=CARTESIAN_POINT('Ctrl Pts',(1.90180124389137,1.,0.440807833704161));
#24409=CARTESIAN_POINT('Ctrl Pts',(1.89663648956549,-1.,0.437995003948443));
#24410=CARTESIAN_POINT('Ctrl Pts',(1.89663648956549,1.,0.437995003948443));
#24411=CARTESIAN_POINT('Ctrl Pts',(1.89136993975585,-1.,0.43522566096358));
#24412=CARTESIAN_POINT('Ctrl Pts',(1.89136993975585,1.,0.43522566096358));
#24413=CARTESIAN_POINT('Ctrl Pts',(1.88596913666828,-1.,0.432493038548833));
#24414=CARTESIAN_POINT('Ctrl Pts',(1.88596913666828,1.,0.432493038548833));
#24415=CARTESIAN_POINT('Ctrl Pts',(1.88044229001778,-1.,0.429803062482217));
#24416=CARTESIAN_POINT('Ctrl Pts',(1.88044229001778,1.,0.429803062482217));
#24417=CARTESIAN_POINT('Ctrl Pts',(1.87486989291333,-1.,0.427183828518743));
#24418=CARTESIAN_POINT('Ctrl Pts',(1.87486989291333,1.,0.427183828518743));
#24419=CARTESIAN_POINT('Ctrl Pts',(1.8693780394412,-1.,0.424678177290876));
#24420=CARTESIAN_POINT('Ctrl Pts',(1.8693780394412,1.,0.424678177290876));
#24421=CARTESIAN_POINT('Ctrl Pts',(1.86408083333863,-1.,0.422327307417885));
#24422=CARTESIAN_POINT('Ctrl Pts',(1.86408083333863,1.,0.422327307417885));
#24423=CARTESIAN_POINT('Ctrl Pts',(1.8590328109667,-1.,0.420157287975583));
#24424=CARTESIAN_POINT('Ctrl Pts',(1.8590328109667,1.,0.420157287975583));
#24425=CARTESIAN_POINT('Ctrl Pts',(1.8541763285645,-1.,0.418164129144046));
#24426=CARTESIAN_POINT('Ctrl Pts',(1.8541763285645,1.,0.418164129144046));
#24427=CARTESIAN_POINT('Ctrl Pts',(1.84929312930314,-1.,0.416300022039885));
#24428=CARTESIAN_POINT('Ctrl Pts',(1.84929312930314,1.,0.416300022039885));
#24429=CARTESIAN_POINT('Ctrl Pts',(1.84405757074218,-1.,0.414487438255542));
#24430=CARTESIAN_POINT('Ctrl Pts',(1.84405757074218,1.,0.414487438255542));
#24431=CARTESIAN_POINT('Ctrl Pts',(1.8380895347617,-1.,0.412633125322945));
#24432=CARTESIAN_POINT('Ctrl Pts',(1.8380895347617,1.,0.412633125322945));
#24433=CARTESIAN_POINT('Ctrl Pts',(1.83100408895047,-1.,0.410641256301276));
#24434=CARTESIAN_POINT('Ctrl Pts',(1.83100408895047,1.,0.410641256301276));
#24435=CARTESIAN_POINT('Ctrl Pts',(1.82247022677562,-1.,0.408428948106228));
#24436=CARTESIAN_POINT('Ctrl Pts',(1.82247022677562,1.,0.408428948106228));
#24437=CARTESIAN_POINT('Ctrl Pts',(1.81223801812013,-1.,0.405933518407176));
#24438=CARTESIAN_POINT('Ctrl Pts',(1.81223801812013,1.,0.405933518407176));
#24439=CARTESIAN_POINT('Ctrl Pts',(1.80012077173238,-1.,0.403107976163396));
#24440=CARTESIAN_POINT('Ctrl Pts',(1.80012077173238,1.,0.403107976163396));
#24441=CARTESIAN_POINT('Ctrl Pts',(1.78598826343754,-1.,0.399919403774156));
#24442=CARTESIAN_POINT('Ctrl Pts',(1.78598826343754,1.,0.399919403774156));
#24443=CARTESIAN_POINT('Ctrl Pts',(1.76975560043442,-1.,0.396346196110688));
#24444=CARTESIAN_POINT('Ctrl Pts',(1.76975560043442,1.,0.396346196110688));
#24445=CARTESIAN_POINT('Ctrl Pts',(1.75137405310193,-1.,0.392375812285396));
#24446=CARTESIAN_POINT('Ctrl Pts',(1.75137405310193,1.,0.392375812285396));
#24447=CARTESIAN_POINT('Ctrl Pts',(1.73493170972829,-1.,0.388877023502615));
#24448=CARTESIAN_POINT('Ctrl Pts',(1.73493170972829,1.,0.388877023502615));
#24449=CARTESIAN_POINT('Ctrl Pts',(1.72162022244582,-1.,0.386070790323281));
#24450=CARTESIAN_POINT('Ctrl Pts',(1.72162022244582,1.,0.386070790323281));
#24451=CARTESIAN_POINT('Ctrl Pts',(1.71231062891398,-1.,0.384119047314215));
#24452=CARTESIAN_POINT('Ctrl Pts',(1.71231062891398,1.,0.384119047314215));
#24453=CARTESIAN_POINT('Ctrl Pts',(1.7075470150345,-1.,0.383122945602004));
#24454=CARTESIAN_POINT('Ctrl Pts',(1.7075470150345,1.,0.383122945602004));
#24455=CARTESIAN_POINT('',(1.7075470150345,1.,0.383122945602004));
#24456=CARTESIAN_POINT('',(1.7075470150345,0.,0.383122945602005));
#24457=CARTESIAN_POINT('',(2.11275013067528,1.,0.613422273260091));
#24458=CARTESIAN_POINT('Ctrl Pts',(2.11275013067528,1.,0.613422273260091));
#24459=CARTESIAN_POINT('Ctrl Pts',(2.11187554260142,1.,0.61246736556225));
#24460=CARTESIAN_POINT('Ctrl Pts',(2.11012443807661,1.,0.610560911691114));
#24461=CARTESIAN_POINT('Ctrl Pts',(2.10749199615859,1.,0.607711315456826));
#24462=CARTESIAN_POINT('Ctrl Pts',(2.10397049887709,1.,0.603932030738212));
#24463=CARTESIAN_POINT('Ctrl Pts',(2.09954930865331,1.,0.599241616422144));
#24464=CARTESIAN_POINT('Ctrl Pts',(2.09510876220501,1.,0.594585006052824));
#24465=CARTESIAN_POINT('Ctrl Pts',(2.09064881812053,1.,0.58996236540319));
#24466=CARTESIAN_POINT('Ctrl Pts',(2.086169437277,1.,0.585373918990895));
#24467=CARTESIAN_POINT('Ctrl Pts',(2.08167059018138,1.,0.580819952107257));
#24468=CARTESIAN_POINT('Ctrl Pts',(2.07715226767361,1.,0.576300797416275));
#24469=CARTESIAN_POINT('Ctrl Pts',(2.07261449292757,1.,0.571816823242411));
#24470=CARTESIAN_POINT('Ctrl Pts',(2.06805732997383,1.,0.56736842118123));
#24471=CARTESIAN_POINT('Ctrl Pts',(2.06348090160697,1.,0.562955993082574));
#24472=CARTESIAN_POINT('Ctrl Pts',(2.05888537756571,1.,0.558579940185468));
#24473=CARTESIAN_POINT('Ctrl Pts',(2.05427091604482,1.,0.55424065746411));
#24474=CARTESIAN_POINT('Ctrl Pts',(2.04963761077974,1.,0.549938525150342));
#24475=CARTESIAN_POINT('Ctrl Pts',(2.0449854471456,1.,0.545673903817349));
#24476=CARTESIAN_POINT('Ctrl Pts',(2.0403142269048,1.,0.54144712061552));
#24477=CARTESIAN_POINT('Ctrl Pts',(2.03562362953993,1.,0.537258489833135));
#24478=CARTESIAN_POINT('Ctrl Pts',(2.03091336214401,1.,0.533108355132905));
#24479=CARTESIAN_POINT('Ctrl Pts',(2.02618329083289,1.,0.528997127241911));
#24480=CARTESIAN_POINT('Ctrl Pts',(2.02143356304712,1.,0.524925318333519));
#24481=CARTESIAN_POINT('Ctrl Pts',(2.01666477917305,1.,0.520893590399429));
#24482=CARTESIAN_POINT('Ctrl Pts',(2.01187773939257,1.,0.516902681728733));
#24483=CARTESIAN_POINT('Ctrl Pts',(2.00707309946955,1.,0.512953306961814));
#24484=CARTESIAN_POINT('Ctrl Pts',(2.00225107134733,1.,0.509046069886152));
#24485=CARTESIAN_POINT('Ctrl Pts',(1.99741107463567,1.,0.505181361323011));
#24486=CARTESIAN_POINT('Ctrl Pts',(1.9925514912615,1.,0.501359287727129));
#24487=CARTESIAN_POINT('Ctrl Pts',(1.98767044752929,1.,0.497579909545564));
#24488=CARTESIAN_POINT('Ctrl Pts',(1.9827665876182,1.,0.493843476541493));
#24489=CARTESIAN_POINT('Ctrl Pts',(1.97783973019229,1.,0.490150627860955));
#24490=CARTESIAN_POINT('Ctrl Pts',(1.97289186263272,1.,0.486502692907661));
#24491=CARTESIAN_POINT('Ctrl Pts',(1.96792703422358,1.,0.482901662120687));
#24492=CARTESIAN_POINT('Ctrl Pts',(1.96294933055938,1.,0.479349583074846));
#24493=CARTESIAN_POINT('Ctrl Pts',(1.95796111148175,1.,0.475848034683172));
#24494=CARTESIAN_POINT('Ctrl Pts',(1.95296148278136,1.,0.47239767226408));
#24495=CARTESIAN_POINT('Ctrl Pts',(1.94794381136524,1.,0.468997482913158));
#24496=CARTESIAN_POINT('Ctrl Pts',(1.94289794196205,1.,0.465645462026065));
#24497=CARTESIAN_POINT('Ctrl Pts',(1.93781486640834,1.,0.462340031009087));
#24498=CARTESIAN_POINT('Ctrl Pts',(1.93269066517936,1.,0.459081234547932));
#24499=CARTESIAN_POINT('Ctrl Pts',(1.92753067150461,1.,0.455872005174336));
#24500=CARTESIAN_POINT('Ctrl Pts',(1.9223538064847,1.,0.452719478359356));
#24501=CARTESIAN_POINT('Ctrl Pts',(1.91718342555717,1.,0.449632260106572));
#24502=CARTESIAN_POINT('Ctrl Pts',(1.91203699981095,1.,0.446617343485651));
#24503=CARTESIAN_POINT('Ctrl Pts',(1.90691756144906,1.,0.443677556849171));
#24504=CARTESIAN_POINT('Ctrl Pts',(1.90180124389137,1.,0.440807833704161));
#24505=CARTESIAN_POINT('Ctrl Pts',(1.89663648956549,1.,0.437995003948443));
#24506=CARTESIAN_POINT('Ctrl Pts',(1.89136993975585,1.,0.43522566096358));
#24507=CARTESIAN_POINT('Ctrl Pts',(1.88596913666828,1.,0.432493038548833));
#24508=CARTESIAN_POINT('Ctrl Pts',(1.88044229001778,1.,0.429803062482217));
#24509=CARTESIAN_POINT('Ctrl Pts',(1.87486989291333,1.,0.427183828518743));
#24510=CARTESIAN_POINT('Ctrl Pts',(1.8693780394412,1.,0.424678177290876));
#24511=CARTESIAN_POINT('Ctrl Pts',(1.86408083333863,1.,0.422327307417885));
#24512=CARTESIAN_POINT('Ctrl Pts',(1.8590328109667,1.,0.420157287975583));
#24513=CARTESIAN_POINT('Ctrl Pts',(1.8541763285645,1.,0.418164129144046));
#24514=CARTESIAN_POINT('Ctrl Pts',(1.84929312930314,1.,0.416300022039885));
#24515=CARTESIAN_POINT('Ctrl Pts',(1.84405757074218,1.,0.414487438255542));
#24516=CARTESIAN_POINT('Ctrl Pts',(1.8380895347617,1.,0.412633125322945));
#24517=CARTESIAN_POINT('Ctrl Pts',(1.83100408895047,1.,0.410641256301276));
#24518=CARTESIAN_POINT('Ctrl Pts',(1.82247022677562,1.,0.408428948106228));
#24519=CARTESIAN_POINT('Ctrl Pts',(1.81223801812013,1.,0.405933518407176));
#24520=CARTESIAN_POINT('Ctrl Pts',(1.80012077173238,1.,0.403107976163396));
#24521=CARTESIAN_POINT('Ctrl Pts',(1.78598826343754,1.,0.399919403774156));
#24522=CARTESIAN_POINT('Ctrl Pts',(1.76975560043442,1.,0.396346196110688));
#24523=CARTESIAN_POINT('Ctrl Pts',(1.75137405310193,1.,0.392375812285396));
#24524=CARTESIAN_POINT('Ctrl Pts',(1.73493170972829,1.,0.388877023502615));
#24525=CARTESIAN_POINT('Ctrl Pts',(1.72162022244582,1.,0.386070790323281));
#24526=CARTESIAN_POINT('Ctrl Pts',(1.71231062891398,1.,0.384119047314215));
#24527=CARTESIAN_POINT('Ctrl Pts',(1.7075470150345,1.,0.383122945602004));
#24528=CARTESIAN_POINT('',(2.11275013067528,0.,0.613422273260091));
#24529=CARTESIAN_POINT('Origin',(2.0698113262342,0.,0.745574324794401));
#24530=CARTESIAN_POINT('',(2.0698113262342,1.,0.745574324794401));
#24531=CARTESIAN_POINT('',(2.11275013067528,1.,0.613422273260091));
#24532=CARTESIAN_POINT('',(2.0698113262342,0.,0.745574324794401));
#24533=CARTESIAN_POINT('Ctrl Pts',(1.60662857109684,-1.,0.693717979106306));
#24534=CARTESIAN_POINT('Ctrl Pts',(1.60662857109684,1.,0.693717979106306));
#24535=CARTESIAN_POINT('Ctrl Pts',(1.61106790958151,-1.,0.695712097881194));
#24536=CARTESIAN_POINT('Ctrl Pts',(1.61106790958151,1.,0.695712097881194));
#24537=CARTESIAN_POINT('Ctrl Pts',(1.61974673472612,-1.,0.699605146405088));
#24538=CARTESIAN_POINT('Ctrl Pts',(1.61974673472612,1.,0.699605146405088));
#24539=CARTESIAN_POINT('Ctrl Pts',(1.63216541664676,-1.,0.705159151988319));
#24540=CARTESIAN_POINT('Ctrl Pts',(1.63216541664676,1.,0.705159151988319));
#24541=CARTESIAN_POINT('Ctrl Pts',(1.64752408832016,-1.,0.711993139355394));
#24542=CARTESIAN_POINT('Ctrl Pts',(1.64752408832016,1.,0.711993139355394));
#24543=CARTESIAN_POINT('Ctrl Pts',(1.6647288055568,-1.,0.719585433804282));
#24544=CARTESIAN_POINT('Ctrl Pts',(1.6647288055568,1.,0.719585433804282));
#24545=CARTESIAN_POINT('Ctrl Pts',(1.67996158455503,-1.,0.726235967997433));
#24546=CARTESIAN_POINT('Ctrl Pts',(1.67996158455503,1.,0.726235967997433));
#24547=CARTESIAN_POINT('Ctrl Pts',(1.69326921975743,-1.,0.731963238697195));
#24548=CARTESIAN_POINT('Ctrl Pts',(1.69326921975743,1.,0.731963238697195));
#24549=CARTESIAN_POINT('Ctrl Pts',(1.70473309006121,-1.,0.736799665724771));
#24550=CARTESIAN_POINT('Ctrl Pts',(1.70473309006121,1.,0.736799665724771));
#24551=CARTESIAN_POINT('Ctrl Pts',(1.71447789751927,-1.,0.740795162032088));
#24552=CARTESIAN_POINT('Ctrl Pts',(1.71447789751927,1.,0.740795162032088));
#24553=CARTESIAN_POINT('Ctrl Pts',(1.7226822991693,-1.,0.744021445433765));
#24554=CARTESIAN_POINT('Ctrl Pts',(1.7226822991693,1.,0.744021445433765));
#24555=CARTESIAN_POINT('Ctrl Pts',(1.72958533647399,-1.,0.746574710096437));
#24556=CARTESIAN_POINT('Ctrl Pts',(1.72958533647399,1.,0.746574710096437));
#24557=CARTESIAN_POINT('Ctrl Pts',(1.73550351679848,-1.,0.748582462954855));
#24558=CARTESIAN_POINT('Ctrl Pts',(1.73550351679848,1.,0.748582462954855));
#24559=CARTESIAN_POINT('Ctrl Pts',(1.74080458266705,-1.,0.750193435979541));
#24560=CARTESIAN_POINT('Ctrl Pts',(1.74080458266705,1.,0.750193435979541));
#24561=CARTESIAN_POINT('Ctrl Pts',(1.74585086852298,-1.,0.751555614163629));
#24562=CARTESIAN_POINT('Ctrl Pts',(1.74585086852298,1.,0.751555614163629));
#24563=CARTESIAN_POINT('Ctrl Pts',(1.75095139468809,-1.,0.752797683531377));
#24564=CARTESIAN_POINT('Ctrl Pts',(1.75095139468809,1.,0.752797683531377));
#24565=CARTESIAN_POINT('Ctrl Pts',(1.75631083600175,-1.,0.75400925402848));
#24566=CARTESIAN_POINT('Ctrl Pts',(1.75631083600175,1.,0.75400925402848));
#24567=CARTESIAN_POINT('Ctrl Pts',(1.7619781724032,-1.,0.755220979975262));
#24568=CARTESIAN_POINT('Ctrl Pts',(1.7619781724032,1.,0.755220979975262));
#24569=CARTESIAN_POINT('Ctrl Pts',(1.76789396003141,-1.,0.756421896028403));
#24570=CARTESIAN_POINT('Ctrl Pts',(1.76789396003141,1.,0.756421896028403));
#24571=CARTESIAN_POINT('Ctrl Pts',(1.77394167108342,-1.,0.757578264077238));
#24572=CARTESIAN_POINT('Ctrl Pts',(1.77394167108342,1.,0.757578264077238));
#24573=CARTESIAN_POINT('Ctrl Pts',(1.77999411220912,-1.,0.75865062667738));
#24574=CARTESIAN_POINT('Ctrl Pts',(1.77999411220912,1.,0.75865062667738));
#24575=CARTESIAN_POINT('Ctrl Pts',(1.78596964884526,-1.,0.759614401109868));
#24576=CARTESIAN_POINT('Ctrl Pts',(1.78596964884526,1.,0.759614401109868));
#24577=CARTESIAN_POINT('Ctrl Pts',(1.79185815610802,-1.,0.760469555880425));
#24578=CARTESIAN_POINT('Ctrl Pts',(1.79185815610802,1.,0.760469555880425));
#24579=CARTESIAN_POINT('Ctrl Pts',(1.79768986997735,-1.,0.761229695230359));
#24580=CARTESIAN_POINT('Ctrl Pts',(1.79768986997735,1.,0.761229695230359));
#24581=CARTESIAN_POINT('Ctrl Pts',(1.80351583877334,-1.,0.761915336443516));
#24582=CARTESIAN_POINT('Ctrl Pts',(1.80351583877334,1.,0.761915336443516));
#24583=CARTESIAN_POINT('Ctrl Pts',(1.80938551463989,-1.,0.762546129464036));
#24584=CARTESIAN_POINT('Ctrl Pts',(1.80938551463989,1.,0.762546129464036));
#24585=CARTESIAN_POINT('Ctrl Pts',(1.81532118405566,-1.,0.763132003836783));
#24586=CARTESIAN_POINT('Ctrl Pts',(1.81532118405566,1.,0.763132003836783));
#24587=CARTESIAN_POINT('Ctrl Pts',(1.82131873145297,-1.,0.763673465462854));
#24588=CARTESIAN_POINT('Ctrl Pts',(1.82131873145297,1.,0.763673465462854));
#24589=CARTESIAN_POINT('Ctrl Pts',(1.8273599120008,-1.,0.764165902606056));
#24590=CARTESIAN_POINT('Ctrl Pts',(1.8273599120008,1.,0.764165902606056));
#24591=CARTESIAN_POINT('Ctrl Pts',(1.8334207722714,-1.,0.764602549687846));
#24592=CARTESIAN_POINT('Ctrl Pts',(1.8334207722714,1.,0.764602549687846));
#24593=CARTESIAN_POINT('Ctrl Pts',(1.83948181064823,-1.,0.764978057881688));
#24594=CARTESIAN_POINT('Ctrl Pts',(1.83948181064823,1.,0.764978057881688));
#24595=CARTESIAN_POINT('Ctrl Pts',(1.8455369887591,-1.,0.765291664861972));
#24596=CARTESIAN_POINT('Ctrl Pts',(1.8455369887591,1.,0.765291664861972));
#24597=CARTESIAN_POINT('Ctrl Pts',(1.85158945130054,-1.,0.765545710619023));
#24598=CARTESIAN_POINT('Ctrl Pts',(1.85158945130054,1.,0.765545710619023));
#24599=CARTESIAN_POINT('Ctrl Pts',(1.85764741390391,-1.,0.765744212909305));
#24600=CARTESIAN_POINT('Ctrl Pts',(1.85764741390391,1.,0.765744212909305));
#24601=CARTESIAN_POINT('Ctrl Pts',(1.86372027063314,-1.,0.765891519092557));
#24602=CARTESIAN_POINT('Ctrl Pts',(1.86372027063314,1.,0.765891519092557));
#24603=CARTESIAN_POINT('Ctrl Pts',(1.86981398314345,-1.,0.765990708546112));
#24604=CARTESIAN_POINT('Ctrl Pts',(1.86981398314345,1.,0.765990708546112));
#24605=CARTESIAN_POINT('Ctrl Pts',(1.87592888967886,-1.,0.766042837036759));
#24606=CARTESIAN_POINT('Ctrl Pts',(1.87592888967886,1.,0.766042837036759));
#24607=CARTESIAN_POINT('Ctrl Pts',(1.88206215302561,-1.,0.766047794851869));
#24608=CARTESIAN_POINT('Ctrl Pts',(1.88206215302561,1.,0.766047794851869));
#24609=CARTESIAN_POINT('Ctrl Pts',(1.88820926433409,-1.,0.76600483706209));
#24610=CARTESIAN_POINT('Ctrl Pts',(1.88820926433409,1.,0.76600483706209));
#24611=CARTESIAN_POINT('Ctrl Pts',(1.89436577771389,-1.,0.765913193856979));
#24612=CARTESIAN_POINT('Ctrl Pts',(1.89436577771389,1.,0.765913193856979));
#24613=CARTESIAN_POINT('Ctrl Pts',(1.90052930393599,-1.,0.765772772593395));
#24614=CARTESIAN_POINT('Ctrl Pts',(1.90052930393599,1.,0.765772772593395));
#24615=CARTESIAN_POINT('Ctrl Pts',(1.90669961402362,-1.,0.765584196937937));
#24616=CARTESIAN_POINT('Ctrl Pts',(1.90669961402362,1.,0.765584196937937));
#24617=CARTESIAN_POINT('Ctrl Pts',(1.91287765805174,-1.,0.765348465884739));
#24618=CARTESIAN_POINT('Ctrl Pts',(1.91287765805174,1.,0.765348465884739));
#24619=CARTESIAN_POINT('Ctrl Pts',(1.91906491634197,-1.,0.765066729667095));
#24620=CARTESIAN_POINT('Ctrl Pts',(1.91906491634197,1.,0.765066729667095));
#24621=CARTESIAN_POINT('Ctrl Pts',(1.92526263537041,-1.,0.764740025488189));
#24622=CARTESIAN_POINT('Ctrl Pts',(1.92526263537041,1.,0.764740025488189));
#24623=CARTESIAN_POINT('Ctrl Pts',(1.93147105496367,-1.,0.76436901067389));
#24624=CARTESIAN_POINT('Ctrl Pts',(1.93147105496367,1.,0.76436901067389));
#24625=CARTESIAN_POINT('Ctrl Pts',(1.93768964875867,-1.,0.763954049121394));
#24626=CARTESIAN_POINT('Ctrl Pts',(1.93768964875867,1.,0.763954049121394));
#24627=CARTESIAN_POINT('Ctrl Pts',(1.94391746617626,-1.,0.763495333538581));
#24628=CARTESIAN_POINT('Ctrl Pts',(1.94391746617626,1.,0.763495333538581));
#24629=CARTESIAN_POINT('Ctrl Pts',(1.95015342590025,-1.,0.762992990878774));
#24630=CARTESIAN_POINT('Ctrl Pts',(1.95015342590025,1.,0.762992990878774));
#24631=CARTESIAN_POINT('Ctrl Pts',(1.95639665309893,-1.,0.762447203806264));
#24632=CARTESIAN_POINT('Ctrl Pts',(1.95639665309893,1.,0.762447203806264));
#24633=CARTESIAN_POINT('Ctrl Pts',(1.96264672744229,-1.,0.761858300014575));
#24634=CARTESIAN_POINT('Ctrl Pts',(1.96264672744229,1.,0.761858300014575));
#24635=CARTESIAN_POINT('Ctrl Pts',(1.96890351582545,-1.,0.761226690483986));
#24636=CARTESIAN_POINT('Ctrl Pts',(1.96890351582545,1.,0.761226690483986));
#24637=CARTESIAN_POINT('Ctrl Pts',(1.97516705321521,-1.,0.760552825409856));
#24638=CARTESIAN_POINT('Ctrl Pts',(1.97516705321521,1.,0.760552825409856));
#24639=CARTESIAN_POINT('Ctrl Pts',(1.98143741418156,-1.,0.759837147452135));
#24640=CARTESIAN_POINT('Ctrl Pts',(1.98143741418156,1.,0.759837147452135));
#24641=CARTESIAN_POINT('Ctrl Pts',(1.98771456680806,-1.,0.759080037802243));
#24642=CARTESIAN_POINT('Ctrl Pts',(1.98771456680806,1.,0.759080037802243));
#24643=CARTESIAN_POINT('Ctrl Pts',(1.9939983109871,-1.,0.758281796766377));
#24644=CARTESIAN_POINT('Ctrl Pts',(1.9939983109871,1.,0.758281796766377));
#24645=CARTESIAN_POINT('Ctrl Pts',(2.00028834739072,-1.,0.757442676862342));
#24646=CARTESIAN_POINT('Ctrl Pts',(2.00028834739072,1.,0.757442676862342));
#24647=CARTESIAN_POINT('Ctrl Pts',(2.00658431587682,-1.,0.756562904646496));
#24648=CARTESIAN_POINT('Ctrl Pts',(2.00658431587682,1.,0.756562904646496));
#24649=CARTESIAN_POINT('Ctrl Pts',(2.01288584328149,-1.,0.755642704958101));
#24650=CARTESIAN_POINT('Ctrl Pts',(2.01288584328149,1.,0.755642704958101));
#24651=CARTESIAN_POINT('Ctrl Pts',(2.01919259406003,-1.,0.75468233072352));
#24652=CARTESIAN_POINT('Ctrl Pts',(2.01919259406003,1.,0.75468233072352));
#24653=CARTESIAN_POINT('Ctrl Pts',(2.02550428623587,-1.,0.753682061113766));
#24654=CARTESIAN_POINT('Ctrl Pts',(2.02550428623587,1.,0.753682061113766));
#24655=CARTESIAN_POINT('Ctrl Pts',(2.03182068456467,-1.,0.752642180488104));
#24656=CARTESIAN_POINT('Ctrl Pts',(2.03182068456467,1.,0.752642180488104));
#24657=CARTESIAN_POINT('Ctrl Pts',(2.03814160092173,-1.,0.751562963361384));
#24658=CARTESIAN_POINT('Ctrl Pts',(2.03814160092173,1.,0.751562963361384));
#24659=CARTESIAN_POINT('Ctrl Pts',(2.04446689147754,-1.,0.750444657874758));
#24660=CARTESIAN_POINT('Ctrl Pts',(2.04446689147754,1.,0.750444657874758));
#24661=CARTESIAN_POINT('Ctrl Pts',(2.05079645591606,-1.,0.749287468663053));
#24662=CARTESIAN_POINT('Ctrl Pts',(2.05079645591606,1.,0.749287468663053));
#24663=CARTESIAN_POINT('Ctrl Pts',(2.05713023030263,-1.,0.748091554181101));
#24664=CARTESIAN_POINT('Ctrl Pts',(2.05713023030263,1.,0.748091554181101));
#24665=CARTESIAN_POINT('Ctrl Pts',(2.06220058927162,-1.,0.747103932785504));
#24666=CARTESIAN_POINT('Ctrl Pts',(2.06220058927162,1.,0.747103932785504));
#24667=CARTESIAN_POINT('Ctrl Pts',(2.06600523016401,-1.,0.746345871542696));
#24668=CARTESIAN_POINT('Ctrl Pts',(2.06600523016401,1.,0.746345871542696));
#24669=CARTESIAN_POINT('Ctrl Pts',(2.06854248895575,-1.,0.74583279137781));
#24670=CARTESIAN_POINT('Ctrl Pts',(2.06854248895575,1.,0.74583279137781));
#24671=CARTESIAN_POINT('Ctrl Pts',(2.0698113262342,-1.,0.745574324794401));
#24672=CARTESIAN_POINT('Ctrl Pts',(2.0698113262342,1.,0.745574324794401));
#24673=CARTESIAN_POINT('',(1.60662857109684,1.,0.693717979106306));
#24674=CARTESIAN_POINT('Ctrl Pts',(1.60662857109684,1.,0.693717979106306));
#24675=CARTESIAN_POINT('Ctrl Pts',(1.61106790958151,1.,0.695712097881194));
#24676=CARTESIAN_POINT('Ctrl Pts',(1.61974673472612,1.,0.699605146405088));
#24677=CARTESIAN_POINT('Ctrl Pts',(1.63216541664676,1.,0.705159151988319));
#24678=CARTESIAN_POINT('Ctrl Pts',(1.64752408832016,1.,0.711993139355394));
#24679=CARTESIAN_POINT('Ctrl Pts',(1.6647288055568,1.,0.719585433804282));
#24680=CARTESIAN_POINT('Ctrl Pts',(1.67996158455503,1.,0.726235967997433));
#24681=CARTESIAN_POINT('Ctrl Pts',(1.69326921975743,1.,0.731963238697195));
#24682=CARTESIAN_POINT('Ctrl Pts',(1.70473309006121,1.,0.736799665724771));
#24683=CARTESIAN_POINT('Ctrl Pts',(1.71447789751927,1.,0.740795162032088));
#24684=CARTESIAN_POINT('Ctrl Pts',(1.7226822991693,1.,0.744021445433765));
#24685=CARTESIAN_POINT('Ctrl Pts',(1.72958533647399,1.,0.746574710096437));
#24686=CARTESIAN_POINT('Ctrl Pts',(1.73550351679848,1.,0.748582462954855));
#24687=CARTESIAN_POINT('Ctrl Pts',(1.74080458266705,1.,0.750193435979541));
#24688=CARTESIAN_POINT('Ctrl Pts',(1.74585086852298,1.,0.751555614163629));
#24689=CARTESIAN_POINT('Ctrl Pts',(1.75095139468809,1.,0.752797683531377));
#24690=CARTESIAN_POINT('Ctrl Pts',(1.75631083600175,1.,0.75400925402848));
#24691=CARTESIAN_POINT('Ctrl Pts',(1.7619781724032,1.,0.755220979975262));
#24692=CARTESIAN_POINT('Ctrl Pts',(1.76789396003141,1.,0.756421896028403));
#24693=CARTESIAN_POINT('Ctrl Pts',(1.77394167108342,1.,0.757578264077238));
#24694=CARTESIAN_POINT('Ctrl Pts',(1.77999411220912,1.,0.75865062667738));
#24695=CARTESIAN_POINT('Ctrl Pts',(1.78596964884526,1.,0.759614401109868));
#24696=CARTESIAN_POINT('Ctrl Pts',(1.79185815610802,1.,0.760469555880425));
#24697=CARTESIAN_POINT('Ctrl Pts',(1.79768986997735,1.,0.761229695230359));
#24698=CARTESIAN_POINT('Ctrl Pts',(1.80351583877334,1.,0.761915336443516));
#24699=CARTESIAN_POINT('Ctrl Pts',(1.80938551463989,1.,0.762546129464036));
#24700=CARTESIAN_POINT('Ctrl Pts',(1.81532118405566,1.,0.763132003836783));
#24701=CARTESIAN_POINT('Ctrl Pts',(1.82131873145297,1.,0.763673465462854));
#24702=CARTESIAN_POINT('Ctrl Pts',(1.8273599120008,1.,0.764165902606056));
#24703=CARTESIAN_POINT('Ctrl Pts',(1.8334207722714,1.,0.764602549687846));
#24704=CARTESIAN_POINT('Ctrl Pts',(1.83948181064823,1.,0.764978057881688));
#24705=CARTESIAN_POINT('Ctrl Pts',(1.8455369887591,1.,0.765291664861972));
#24706=CARTESIAN_POINT('Ctrl Pts',(1.85158945130054,1.,0.765545710619023));
#24707=CARTESIAN_POINT('Ctrl Pts',(1.85764741390391,1.,0.765744212909305));
#24708=CARTESIAN_POINT('Ctrl Pts',(1.86372027063314,1.,0.765891519092557));
#24709=CARTESIAN_POINT('Ctrl Pts',(1.86981398314345,1.,0.765990708546112));
#24710=CARTESIAN_POINT('Ctrl Pts',(1.87592888967886,1.,0.766042837036759));
#24711=CARTESIAN_POINT('Ctrl Pts',(1.88206215302561,1.,0.766047794851869));
#24712=CARTESIAN_POINT('Ctrl Pts',(1.88820926433409,1.,0.76600483706209));
#24713=CARTESIAN_POINT('Ctrl Pts',(1.89436577771389,1.,0.765913193856979));
#24714=CARTESIAN_POINT('Ctrl Pts',(1.90052930393599,1.,0.765772772593395));
#24715=CARTESIAN_POINT('Ctrl Pts',(1.90669961402362,1.,0.765584196937937));
#24716=CARTESIAN_POINT('Ctrl Pts',(1.91287765805174,1.,0.765348465884739));
#24717=CARTESIAN_POINT('Ctrl Pts',(1.91906491634197,1.,0.765066729667095));
#24718=CARTESIAN_POINT('Ctrl Pts',(1.92526263537041,1.,0.764740025488189));
#24719=CARTESIAN_POINT('Ctrl Pts',(1.93147105496367,1.,0.76436901067389));
#24720=CARTESIAN_POINT('Ctrl Pts',(1.93768964875867,1.,0.763954049121394));
#24721=CARTESIAN_POINT('Ctrl Pts',(1.94391746617626,1.,0.763495333538581));
#24722=CARTESIAN_POINT('Ctrl Pts',(1.95015342590025,1.,0.762992990878774));
#24723=CARTESIAN_POINT('Ctrl Pts',(1.95639665309893,1.,0.762447203806264));
#24724=CARTESIAN_POINT('Ctrl Pts',(1.96264672744229,1.,0.761858300014575));
#24725=CARTESIAN_POINT('Ctrl Pts',(1.96890351582545,1.,0.761226690483986));
#24726=CARTESIAN_POINT('Ctrl Pts',(1.97516705321521,1.,0.760552825409856));
#24727=CARTESIAN_POINT('Ctrl Pts',(1.98143741418156,1.,0.759837147452135));
#24728=CARTESIAN_POINT('Ctrl Pts',(1.98771456680806,1.,0.759080037802243));
#24729=CARTESIAN_POINT('Ctrl Pts',(1.9939983109871,1.,0.758281796766377));
#24730=CARTESIAN_POINT('Ctrl Pts',(2.00028834739072,1.,0.757442676862342));
#24731=CARTESIAN_POINT('Ctrl Pts',(2.00658431587682,1.,0.756562904646496));
#24732=CARTESIAN_POINT('Ctrl Pts',(2.01288584328149,1.,0.755642704958101));
#24733=CARTESIAN_POINT('Ctrl Pts',(2.01919259406003,1.,0.75468233072352));
#24734=CARTESIAN_POINT('Ctrl Pts',(2.02550428623587,1.,0.753682061113766));
#24735=CARTESIAN_POINT('Ctrl Pts',(2.03182068456467,1.,0.752642180488104));
#24736=CARTESIAN_POINT('Ctrl Pts',(2.03814160092173,1.,0.751562963361384));
#24737=CARTESIAN_POINT('Ctrl Pts',(2.04446689147754,1.,0.750444657874758));
#24738=CARTESIAN_POINT('Ctrl Pts',(2.05079645591606,1.,0.749287468663053));
#24739=CARTESIAN_POINT('Ctrl Pts',(2.05713023030263,1.,0.748091554181101));
#24740=CARTESIAN_POINT('Ctrl Pts',(2.06220058927162,1.,0.747103932785504));
#24741=CARTESIAN_POINT('Ctrl Pts',(2.06600523016401,1.,0.746345871542696));
#24742=CARTESIAN_POINT('Ctrl Pts',(2.06854248895575,1.,0.74583279137781));
#24743=CARTESIAN_POINT('Ctrl Pts',(2.0698113262342,1.,0.745574324794401));
#24744=CARTESIAN_POINT('',(1.60662857109684,0.,0.693717979106305));
#24745=CARTESIAN_POINT('Origin',(0.,0.,0.));
#24746=CARTESIAN_POINT('',(1.5055822144029,1.,0.892032620296856));
#24747=CARTESIAN_POINT('Origin',(0.,1.,0.));
#24748=CARTESIAN_POINT('',(1.5055822144029,0.,0.892032620296855));
#24749=CARTESIAN_POINT('Ctrl Pts',(1.81978687191668,-1.,1.23627494547115));
#24750=CARTESIAN_POINT('Ctrl Pts',(1.81978687191668,1.,1.23627494547115));
#24751=CARTESIAN_POINT('Ctrl Pts',(1.81925017193666,-1.,1.23509651170476));
#24752=CARTESIAN_POINT('Ctrl Pts',(1.81925017193666,1.,1.23509651170476));
#24753=CARTESIAN_POINT('Ctrl Pts',(1.81817389921279,-1.,1.2327422452705));
#24754=CARTESIAN_POINT('Ctrl Pts',(1.81817389921279,1.,1.2327422452705));
#24755=CARTESIAN_POINT('Ctrl Pts',(1.8165508718364,-1.,1.2292186489137));
#24756=CARTESIAN_POINT('Ctrl Pts',(1.8165508718364,1.,1.2292186489137));
#24757=CARTESIAN_POINT('Ctrl Pts',(1.81436959210434,-1.,1.2245361330495));
#24758=CARTESIAN_POINT('Ctrl Pts',(1.81436959210434,1.,1.2245361330495));
#24759=CARTESIAN_POINT('Ctrl Pts',(1.81161420806656,-1.,1.21870906103557));
#24760=CARTESIAN_POINT('Ctrl Pts',(1.81161420806656,1.,1.21870906103557));
#24761=CARTESIAN_POINT('Ctrl Pts',(1.80882996917129,-1.,1.21290815708314));
#24762=CARTESIAN_POINT('Ctrl Pts',(1.80882996917129,1.,1.21290815708314));
#24763=CARTESIAN_POINT('Ctrl Pts',(1.80601678480707,-1.,1.20713356605475));
#24764=CARTESIAN_POINT('Ctrl Pts',(1.80601678480707,1.,1.20713356605475));
#24765=CARTESIAN_POINT('Ctrl Pts',(1.80317454838603,-1.,1.20138548938974));
#24766=CARTESIAN_POINT('Ctrl Pts',(1.80317454838603,1.,1.20138548938974));
#24767=CARTESIAN_POINT('Ctrl Pts',(1.80030314369879,-1.,1.19566418930242));
#24768=CARTESIAN_POINT('Ctrl Pts',(1.80030314369879,1.,1.19566418930242));
#24769=CARTESIAN_POINT('Ctrl Pts',(1.79740245923478,-1.,1.18996997934445));
#24770=CARTESIAN_POINT('Ctrl Pts',(1.79740245923478,1.,1.18996997934445));
#24771=CARTESIAN_POINT('Ctrl Pts',(1.79447240321515,-1.,1.18430321697432));
#24772=CARTESIAN_POINT('Ctrl Pts',(1.79447240321515,1.,1.18430321697432));
#24773=CARTESIAN_POINT('Ctrl Pts',(1.79151291552689,-1.,1.17866429440809));
#24774=CARTESIAN_POINT('Ctrl Pts',(1.79151291552689,1.,1.17866429440809));
#24775=CARTESIAN_POINT('Ctrl Pts',(1.78852398877616,-1.,1.17305363177328));
#24776=CARTESIAN_POINT('Ctrl Pts',(1.78852398877616,1.,1.17305363177328));
#24777=CARTESIAN_POINT('Ctrl Pts',(1.78550566040443,-1.,1.16747166312303));
#24778=CARTESIAN_POINT('Ctrl Pts',(1.78550566040443,1.,1.16747166312303));
#24779=CARTESIAN_POINT('Ctrl Pts',(1.78245795881009,-1.,1.16191881298499));
#24780=CARTESIAN_POINT('Ctrl Pts',(1.78245795881009,1.,1.16191881298499));
#24781=CARTESIAN_POINT('Ctrl Pts',(1.77938085564275,-1.,1.15639547194698));
#24782=CARTESIAN_POINT('Ctrl Pts',(1.77938085564275,1.,1.15639547194698));
#24783=CARTESIAN_POINT('Ctrl Pts',(1.7762742255701,-1.,1.15090197841515));
#24784=CARTESIAN_POINT('Ctrl Pts',(1.7762742255701,1.,1.15090197841515));
#24785=CARTESIAN_POINT('Ctrl Pts',(1.77313777896194,-1.,1.1454385822692));
#24786=CARTESIAN_POINT('Ctrl Pts',(1.77313777896194,1.,1.1454385822692));
#24787=CARTESIAN_POINT('Ctrl Pts',(1.76997111386769,-1.,1.14000548336975));
#24788=CARTESIAN_POINT('Ctrl Pts',(1.76997111386769,1.,1.14000548336975));
#24789=CARTESIAN_POINT('Ctrl Pts',(1.76677384551862,-1.,1.1346029180462));
#24790=CARTESIAN_POINT('Ctrl Pts',(1.76677384551862,1.,1.1346029180462));
#24791=CARTESIAN_POINT('Ctrl Pts',(1.7635457196617,-1.,1.12923123555075));
#24792=CARTESIAN_POINT('Ctrl Pts',(1.7635457196617,1.,1.12923123555075));
#24793=CARTESIAN_POINT('Ctrl Pts',(1.76028671825096,-1.,1.12389096855086));
#24794=CARTESIAN_POINT('Ctrl Pts',(1.76028671825096,1.,1.12389096855086));
#24795=CARTESIAN_POINT('Ctrl Pts',(1.75699720772105,-1.,1.11858293216763));
#24796=CARTESIAN_POINT('Ctrl Pts',(1.75699720772105,1.,1.11858293216763));
#24797=CARTESIAN_POINT('Ctrl Pts',(1.7536777209463,-1.,1.11330807582551));
#24798=CARTESIAN_POINT('Ctrl Pts',(1.7536777209463,1.,1.11330807582551));
#24799=CARTESIAN_POINT('Ctrl Pts',(1.7503286607592,-1.,1.10806728183007));
#24800=CARTESIAN_POINT('Ctrl Pts',(1.7503286607592,1.,1.10806728183007));
#24801=CARTESIAN_POINT('Ctrl Pts',(1.74695004214923,-1.,1.10286118991143));
#24802=CARTESIAN_POINT('Ctrl Pts',(1.74695004214923,1.,1.10286118991143));
#24803=CARTESIAN_POINT('Ctrl Pts',(1.74354119236208,-1.,1.09768999241226));
#24804=CARTESIAN_POINT('Ctrl Pts',(1.74354119236208,1.,1.09768999241226));
#24805=CARTESIAN_POINT('Ctrl Pts',(1.74010053962247,-1.,1.09255329056493));
#24806=CARTESIAN_POINT('Ctrl Pts',(1.74010053962247,1.,1.09255329056493));
#24807=CARTESIAN_POINT('Ctrl Pts',(1.73662628326091,-1.,1.08745056285427));
#24808=CARTESIAN_POINT('Ctrl Pts',(1.73662628326091,1.,1.08745056285427));
#24809=CARTESIAN_POINT('Ctrl Pts',(1.73311705663407,-1.,1.08238162784749));
#24810=CARTESIAN_POINT('Ctrl Pts',(1.73311705663407,1.,1.08238162784749));
#24811=CARTESIAN_POINT('Ctrl Pts',(1.72957248977424,-1.,1.0773470373727));
#24812=CARTESIAN_POINT('Ctrl Pts',(1.72957248977424,1.,1.0773470373727));
#24813=CARTESIAN_POINT('Ctrl Pts',(1.72599406198488,-1.,1.07234866990252));
#24814=CARTESIAN_POINT('Ctrl Pts',(1.72599406198488,1.,1.07234866990252));
#24815=CARTESIAN_POINT('Ctrl Pts',(1.72238500928453,-1.,1.06738966975462));
#24816=CARTESIAN_POINT('Ctrl Pts',(1.72238500928453,1.,1.06738966975462));
#24817=CARTESIAN_POINT('Ctrl Pts',(1.71874858456904,-1.,1.06247324680647));
#24818=CARTESIAN_POINT('Ctrl Pts',(1.71874858456904,1.,1.06247324680647));
#24819=CARTESIAN_POINT('Ctrl Pts',(1.7150865442702,-1.,1.05760163192479));
#24820=CARTESIAN_POINT('Ctrl Pts',(1.7150865442702,1.,1.05760163192479));
#24821=CARTESIAN_POINT('Ctrl Pts',(1.71139783543989,-1.,1.05277517202855));
#24822=CARTESIAN_POINT('Ctrl Pts',(1.71139783543989,1.,1.05277517202855));
#24823=CARTESIAN_POINT('Ctrl Pts',(1.70767646263649,-1.,1.04799085404995));
#24824=CARTESIAN_POINT('Ctrl Pts',(1.70767646263649,1.,1.04799085404995));
#24825=CARTESIAN_POINT('Ctrl Pts',(1.70391338707982,-1.,1.04324363334554));
#24826=CARTESIAN_POINT('Ctrl Pts',(1.70391338707982,1.,1.04324363334554));
#24827=CARTESIAN_POINT('Ctrl Pts',(1.70010052930962,-1.,1.03852922490789));
#24828=CARTESIAN_POINT('Ctrl Pts',(1.70010052930962,1.,1.03852922490789));
#24829=CARTESIAN_POINT('Ctrl Pts',(1.69623414782771,-1.,1.03384646003588));
#24830=CARTESIAN_POINT('Ctrl Pts',(1.69623414782771,1.,1.03384646003588));
#24831=CARTESIAN_POINT('Ctrl Pts',(1.69231840863458,-1.,1.02919977579147));
#24832=CARTESIAN_POINT('Ctrl Pts',(1.69231840863458,1.,1.02919977579147));
#24833=CARTESIAN_POINT('Ctrl Pts',(1.68836910178447,-1.,1.02460180535255));
#24834=CARTESIAN_POINT('Ctrl Pts',(1.68836910178447,1.,1.02460180535255));
#24835=CARTESIAN_POINT('Ctrl Pts',(1.68440578021706,-1.,1.02006795074201));
#24836=CARTESIAN_POINT('Ctrl Pts',(1.68440578021706,1.,1.02006795074201));
#24837=CARTESIAN_POINT('Ctrl Pts',(1.68044289894798,-1.,1.01561026162773));
#24838=CARTESIAN_POINT('Ctrl Pts',(1.68044289894798,1.,1.01561026162773));
#24839=CARTESIAN_POINT('Ctrl Pts',(1.67648246776464,-1.,1.01123236493511));
#24840=CARTESIAN_POINT('Ctrl Pts',(1.67648246776464,1.,1.01123236493511));
#24841=CARTESIAN_POINT('Ctrl Pts',(1.67250335383293,-1.,1.00692206696414));
#24842=CARTESIAN_POINT('Ctrl Pts',(1.67250335383293,1.,1.00692206696414));
#24843=CARTESIAN_POINT('Ctrl Pts',(1.66846059277303,-1.,1.00265091003727));
#24844=CARTESIAN_POINT('Ctrl Pts',(1.66846059277303,1.,1.00265091003727));
#24845=CARTESIAN_POINT('Ctrl Pts',(1.66430758030376,-1.,0.998389654952758));
#24846=CARTESIAN_POINT('Ctrl Pts',(1.66430758030376,1.,0.998389654952758));
#24847=CARTESIAN_POINT('Ctrl Pts',(1.66001553809947,-1.,0.994121836661306));
#24848=CARTESIAN_POINT('Ctrl Pts',(1.66001553809947,1.,0.994121836661306));
#24849=CARTESIAN_POINT('Ctrl Pts',(1.65559044289699,-1.,0.989855627854165));
#24850=CARTESIAN_POINT('Ctrl Pts',(1.65559044289699,1.,0.989855627854165));
#24851=CARTESIAN_POINT('Ctrl Pts',(1.65110016612638,-1.,0.985642622920821));
#24852=CARTESIAN_POINT('Ctrl Pts',(1.65110016612638,1.,0.985642622920821));
#24853=CARTESIAN_POINT('Ctrl Pts',(1.64665139190656,-1.,0.981562530939489));
#24854=CARTESIAN_POINT('Ctrl Pts',(1.64665139190656,1.,0.981562530939489));
#24855=CARTESIAN_POINT('Ctrl Pts',(1.64233990826687,-1.,0.977689794119417));
#24856=CARTESIAN_POINT('Ctrl Pts',(1.64233990826687,1.,0.977689794119417));
#24857=CARTESIAN_POINT('Ctrl Pts',(1.63820952658144,-1.,0.974066058287419));
#24858=CARTESIAN_POINT('Ctrl Pts',(1.63820952658144,1.,0.974066058287419));
#24859=CARTESIAN_POINT('Ctrl Pts',(1.63420665729798,-1.,0.970669715997509));
#24860=CARTESIAN_POINT('Ctrl Pts',(1.63420665729798,1.,0.970669715997509));
#24861=CARTESIAN_POINT('Ctrl Pts',(1.63013849959461,-1.,0.967387853230345));
#24862=CARTESIAN_POINT('Ctrl Pts',(1.63013849959461,1.,0.967387853230345));
#24863=CARTESIAN_POINT('Ctrl Pts',(1.62571930670187,-1.,0.964046107040536));
#24864=CARTESIAN_POINT('Ctrl Pts',(1.62571930670187,1.,0.964046107040536));
#24865=CARTESIAN_POINT('Ctrl Pts',(1.62061638140221,-1.,0.960438326101729));
#24866=CARTESIAN_POINT('Ctrl Pts',(1.62061638140221,1.,0.960438326101729));
#24867=CARTESIAN_POINT('Ctrl Pts',(1.61449324337085,-1.,0.956354422920671));
#24868=CARTESIAN_POINT('Ctrl Pts',(1.61449324337085,1.,0.956354422920671));
#24869=CARTESIAN_POINT('Ctrl Pts',(1.60706069896936,-1.,0.951613284356035));
#24870=CARTESIAN_POINT('Ctrl Pts',(1.60706069896936,1.,0.951613284356035));
#24871=CARTESIAN_POINT('Ctrl Pts',(1.59810042043673,-1.,0.946078063315257));
#24872=CARTESIAN_POINT('Ctrl Pts',(1.59810042043673,1.,0.946078063315257));
#24873=CARTESIAN_POINT('Ctrl Pts',(1.58744937487176,-1.,0.939646377893399));
#24874=CARTESIAN_POINT('Ctrl Pts',(1.58744937487176,1.,0.939646377893399));
#24875=CARTESIAN_POINT('Ctrl Pts',(1.57499388382243,-1.,0.932246680108685));
#24876=CARTESIAN_POINT('Ctrl Pts',(1.57499388382243,1.,0.932246680108685));
#24877=CARTESIAN_POINT('Ctrl Pts',(1.56065988578893,-1.,0.923832188944341));
#24878=CARTESIAN_POINT('Ctrl Pts',(1.56065988578893,1.,0.923832188944341));
#24879=CARTESIAN_POINT('Ctrl Pts',(1.54440491149498,-1.,0.914375919026456));
#24880=CARTESIAN_POINT('Ctrl Pts',(1.54440491149498,1.,0.914375919026456));
#24881=CARTESIAN_POINT('Ctrl Pts',(1.52984849887993,-1.,0.905967409625651));
#24882=CARTESIAN_POINT('Ctrl Pts',(1.52984849887993,1.,0.905967409625651));
#24883=CARTESIAN_POINT('Ctrl Pts',(1.51805569590094,-1.,0.899185047483511));
#24884=CARTESIAN_POINT('Ctrl Pts',(1.51805569590094,1.,0.899185047483511));
#24885=CARTESIAN_POINT('Ctrl Pts',(1.50980486806688,-1.,0.894452006964544));
#24886=CARTESIAN_POINT('Ctrl Pts',(1.50980486806688,1.,0.894452006964544));
#24887=CARTESIAN_POINT('Ctrl Pts',(1.5055822144029,-1.,0.892032620296856));
#24888=CARTESIAN_POINT('Ctrl Pts',(1.5055822144029,1.,0.892032620296856));
#24889=CARTESIAN_POINT('',(1.81978687191668,1.,1.23627494547115));
#24890=CARTESIAN_POINT('Ctrl Pts',(1.81978687191668,1.,1.23627494547115));
#24891=CARTESIAN_POINT('Ctrl Pts',(1.81925017193666,1.,1.23509651170476));
#24892=CARTESIAN_POINT('Ctrl Pts',(1.81817389921279,1.,1.2327422452705));
#24893=CARTESIAN_POINT('Ctrl Pts',(1.8165508718364,1.,1.2292186489137));
#24894=CARTESIAN_POINT('Ctrl Pts',(1.81436959210434,1.,1.2245361330495));
#24895=CARTESIAN_POINT('Ctrl Pts',(1.81161420806656,1.,1.21870906103557));
#24896=CARTESIAN_POINT('Ctrl Pts',(1.80882996917129,1.,1.21290815708314));
#24897=CARTESIAN_POINT('Ctrl Pts',(1.80601678480707,1.,1.20713356605475));
#24898=CARTESIAN_POINT('Ctrl Pts',(1.80317454838603,1.,1.20138548938974));
#24899=CARTESIAN_POINT('Ctrl Pts',(1.80030314369879,1.,1.19566418930242));
#24900=CARTESIAN_POINT('Ctrl Pts',(1.79740245923478,1.,1.18996997934445));
#24901=CARTESIAN_POINT('Ctrl Pts',(1.79447240321515,1.,1.18430321697432));
#24902=CARTESIAN_POINT('Ctrl Pts',(1.79151291552689,1.,1.17866429440809));
#24903=CARTESIAN_POINT('Ctrl Pts',(1.78852398877616,1.,1.17305363177328));
#24904=CARTESIAN_POINT('Ctrl Pts',(1.78550566040443,1.,1.16747166312303));
#24905=CARTESIAN_POINT('Ctrl Pts',(1.78245795881009,1.,1.16191881298499));
#24906=CARTESIAN_POINT('Ctrl Pts',(1.77938085564275,1.,1.15639547194698));
#24907=CARTESIAN_POINT('Ctrl Pts',(1.7762742255701,1.,1.15090197841515));
#24908=CARTESIAN_POINT('Ctrl Pts',(1.77313777896194,1.,1.1454385822692));
#24909=CARTESIAN_POINT('Ctrl Pts',(1.76997111386769,1.,1.14000548336975));
#24910=CARTESIAN_POINT('Ctrl Pts',(1.76677384551862,1.,1.1346029180462));
#24911=CARTESIAN_POINT('Ctrl Pts',(1.7635457196617,1.,1.12923123555075));
#24912=CARTESIAN_POINT('Ctrl Pts',(1.76028671825096,1.,1.12389096855086));
#24913=CARTESIAN_POINT('Ctrl Pts',(1.75699720772105,1.,1.11858293216763));
#24914=CARTESIAN_POINT('Ctrl Pts',(1.7536777209463,1.,1.11330807582551));
#24915=CARTESIAN_POINT('Ctrl Pts',(1.7503286607592,1.,1.10806728183007));
#24916=CARTESIAN_POINT('Ctrl Pts',(1.74695004214923,1.,1.10286118991143));
#24917=CARTESIAN_POINT('Ctrl Pts',(1.74354119236208,1.,1.09768999241226));
#24918=CARTESIAN_POINT('Ctrl Pts',(1.74010053962247,1.,1.09255329056493));
#24919=CARTESIAN_POINT('Ctrl Pts',(1.73662628326091,1.,1.08745056285427));
#24920=CARTESIAN_POINT('Ctrl Pts',(1.73311705663407,1.,1.08238162784749));
#24921=CARTESIAN_POINT('Ctrl Pts',(1.72957248977424,1.,1.0773470373727));
#24922=CARTESIAN_POINT('Ctrl Pts',(1.72599406198488,1.,1.07234866990252));
#24923=CARTESIAN_POINT('Ctrl Pts',(1.72238500928453,1.,1.06738966975462));
#24924=CARTESIAN_POINT('Ctrl Pts',(1.71874858456904,1.,1.06247324680647));
#24925=CARTESIAN_POINT('Ctrl Pts',(1.7150865442702,1.,1.05760163192479));
#24926=CARTESIAN_POINT('Ctrl Pts',(1.71139783543989,1.,1.05277517202855));
#24927=CARTESIAN_POINT('Ctrl Pts',(1.70767646263649,1.,1.04799085404995));
#24928=CARTESIAN_POINT('Ctrl Pts',(1.70391338707982,1.,1.04324363334554));
#24929=CARTESIAN_POINT('Ctrl Pts',(1.70010052930962,1.,1.03852922490789));
#24930=CARTESIAN_POINT('Ctrl Pts',(1.69623414782771,1.,1.03384646003588));
#24931=CARTESIAN_POINT('Ctrl Pts',(1.69231840863458,1.,1.02919977579147));
#24932=CARTESIAN_POINT('Ctrl Pts',(1.68836910178447,1.,1.02460180535255));
#24933=CARTESIAN_POINT('Ctrl Pts',(1.68440578021706,1.,1.02006795074201));
#24934=CARTESIAN_POINT('Ctrl Pts',(1.68044289894798,1.,1.01561026162773));
#24935=CARTESIAN_POINT('Ctrl Pts',(1.67648246776464,1.,1.01123236493511));
#24936=CARTESIAN_POINT('Ctrl Pts',(1.67250335383293,1.,1.00692206696414));
#24937=CARTESIAN_POINT('Ctrl Pts',(1.66846059277303,1.,1.00265091003727));
#24938=CARTESIAN_POINT('Ctrl Pts',(1.66430758030376,1.,0.998389654952758));
#24939=CARTESIAN_POINT('Ctrl Pts',(1.66001553809947,1.,0.994121836661306));
#24940=CARTESIAN_POINT('Ctrl Pts',(1.65559044289699,1.,0.989855627854165));
#24941=CARTESIAN_POINT('Ctrl Pts',(1.65110016612638,1.,0.985642622920821));
#24942=CARTESIAN_POINT('Ctrl Pts',(1.64665139190656,1.,0.981562530939489));
#24943=CARTESIAN_POINT('Ctrl Pts',(1.64233990826687,1.,0.977689794119417));
#24944=CARTESIAN_POINT('Ctrl Pts',(1.63820952658144,1.,0.974066058287419));
#24945=CARTESIAN_POINT('Ctrl Pts',(1.63420665729798,1.,0.970669715997509));
#24946=CARTESIAN_POINT('Ctrl Pts',(1.63013849959461,1.,0.967387853230345));
#24947=CARTESIAN_POINT('Ctrl Pts',(1.62571930670187,1.,0.964046107040536));
#24948=CARTESIAN_POINT('Ctrl Pts',(1.62061638140221,1.,0.960438326101729));
#24949=CARTESIAN_POINT('Ctrl Pts',(1.61449324337085,1.,0.956354422920671));
#24950=CARTESIAN_POINT('Ctrl Pts',(1.60706069896936,1.,0.951613284356035));
#24951=CARTESIAN_POINT('Ctrl Pts',(1.59810042043673,1.,0.946078063315257));
#24952=CARTESIAN_POINT('Ctrl Pts',(1.58744937487176,1.,0.939646377893399));
#24953=CARTESIAN_POINT('Ctrl Pts',(1.57499388382243,1.,0.932246680108685));
#24954=CARTESIAN_POINT('Ctrl Pts',(1.56065988578893,1.,0.923832188944341));
#24955=CARTESIAN_POINT('Ctrl Pts',(1.54440491149498,1.,0.914375919026456));
#24956=CARTESIAN_POINT('Ctrl Pts',(1.52984849887993,1.,0.905967409625651));
#24957=CARTESIAN_POINT('Ctrl Pts',(1.51805569590094,1.,0.899185047483511));
#24958=CARTESIAN_POINT('Ctrl Pts',(1.50980486806688,1.,0.894452006964544));
#24959=CARTESIAN_POINT('Ctrl Pts',(1.5055822144029,1.,0.892032620296856));
#24960=CARTESIAN_POINT('',(1.81978687191668,0.,1.23627494547115));
#24961=CARTESIAN_POINT('Origin',(1.73811241238545,0.,1.34869019493419));
#24962=CARTESIAN_POINT('',(1.73811241238545,1.,1.34869019493419));
#24963=CARTESIAN_POINT('',(1.81978687191668,1.,1.23627494547115));
#24964=CARTESIAN_POINT('',(1.73811241238545,0.,1.34869019493419));
#24965=CARTESIAN_POINT('Ctrl Pts',(1.31362392696032,-1.,1.15624053661742));
#24966=CARTESIAN_POINT('Ctrl Pts',(1.31362392696032,1.,1.15624053661742));
#24967=CARTESIAN_POINT('Ctrl Pts',(1.31722977216397,-1.,1.15950888730809));
#24968=CARTESIAN_POINT('Ctrl Pts',(1.31722977216397,1.,1.15950888730809));
#24969=CARTESIAN_POINT('Ctrl Pts',(1.32428080721772,-1.,1.16589330093588));
#24970=CARTESIAN_POINT('Ctrl Pts',(1.32428080721772,1.,1.16589330093588));
#24971=CARTESIAN_POINT('Ctrl Pts',(1.33437539347008,-1.,1.17501305789857));
#24972=CARTESIAN_POINT('Ctrl Pts',(1.33437539347008,1.,1.17501305789857));
#24973=CARTESIAN_POINT('Ctrl Pts',(1.34687054001093,-1.,1.18625865667441));
#24974=CARTESIAN_POINT('Ctrl Pts',(1.34687054001093,1.,1.18625865667441));
#24975=CARTESIAN_POINT('Ctrl Pts',(1.36088705043885,-1.,1.1987959077932));
#24976=CARTESIAN_POINT('Ctrl Pts',(1.36088705043885,1.,1.1987959077932));
#24977=CARTESIAN_POINT('Ctrl Pts',(1.37331915607905,-1.,1.20982812925645));
#24978=CARTESIAN_POINT('Ctrl Pts',(1.37331915607905,1.,1.20982812925645));
#24979=CARTESIAN_POINT('Ctrl Pts',(1.38420564527715,-1.,1.21938737280852));
#24980=CARTESIAN_POINT('Ctrl Pts',(1.38420564527715,1.,1.21938737280852));
#24981=CARTESIAN_POINT('Ctrl Pts',(1.39361389568796,-1.,1.22752961899387));
#24982=CARTESIAN_POINT('Ctrl Pts',(1.39361389568796,1.,1.22752961899387));
#24983=CARTESIAN_POINT('Ctrl Pts',(1.40164708206106,-1.,1.23434087290423));
#24984=CARTESIAN_POINT('Ctrl Pts',(1.40164708206106,1.,1.23434087290423));
#24985=CARTESIAN_POINT('Ctrl Pts',(1.40845295531283,-1.,1.23994455029534));
#24986=CARTESIAN_POINT('Ctrl Pts',(1.40845295531283,1.,1.23994455029534));
#24987=CARTESIAN_POINT('Ctrl Pts',(1.41422913175179,-1.,1.24450600513056));
#24988=CARTESIAN_POINT('Ctrl Pts',(1.41422913175179,1.,1.24450600513056));
#24989=CARTESIAN_POINT('Ctrl Pts',(1.41923722596025,-1.,1.24824430986571));
#24990=CARTESIAN_POINT('Ctrl Pts',(1.41923722596025,1.,1.24824430986571));
#24991=CARTESIAN_POINT('Ctrl Pts',(1.42378102115575,-1.,1.2514145557001));
#24992=CARTESIAN_POINT('Ctrl Pts',(1.42378102115575,1.,1.2514145557001));
#24993=CARTESIAN_POINT('Ctrl Pts',(1.42815938799387,-1.,1.25426945222639));
#24994=CARTESIAN_POINT('Ctrl Pts',(1.42815938799387,1.,1.25426945222639));
#24995=CARTESIAN_POINT('Ctrl Pts',(1.43262645609691,-1.,1.25702687965755));
#24996=CARTESIAN_POINT('Ctrl Pts',(1.43262645609691,1.,1.25702687965755));
#24997=CARTESIAN_POINT('Ctrl Pts',(1.43734919180847,-1.,1.25983531012005));
#24998=CARTESIAN_POINT('Ctrl Pts',(1.43734919180847,1.,1.25983531012005));
#24999=CARTESIAN_POINT('Ctrl Pts',(1.44236470511303,-1.,1.26273903323859));
#25000=CARTESIAN_POINT('Ctrl Pts',(1.44236470511303,1.,1.26273903323859));
#25001=CARTESIAN_POINT('Ctrl Pts',(1.44761985001662,-1.,1.26570925118868));
#25002=CARTESIAN_POINT('Ctrl Pts',(1.44761985001662,1.,1.26570925118868));
#25003=CARTESIAN_POINT('Ctrl Pts',(1.45301422764247,-1.,1.2686778680489));
#25004=CARTESIAN_POINT('Ctrl Pts',(1.45301422764247,1.,1.2686778680489));
#25005=CARTESIAN_POINT('Ctrl Pts',(1.45843906294697,-1.,1.27156805265289));
#25006=CARTESIAN_POINT('Ctrl Pts',(1.45843906294697,1.,1.27156805265289));
#25007=CARTESIAN_POINT('Ctrl Pts',(1.46382431332476,-1.,1.27433119897822));
#25008=CARTESIAN_POINT('Ctrl Pts',(1.46382431332476,1.,1.27433119897822));
#25009=CARTESIAN_POINT('Ctrl Pts',(1.46916035917133,-1.,1.2769641483109));
#25010=CARTESIAN_POINT('Ctrl Pts',(1.46916035917133,1.,1.2769641483109));
#25011=CARTESIAN_POINT('Ctrl Pts',(1.4744717526707,-1.,1.2794891824849));
#25012=CARTESIAN_POINT('Ctrl Pts',(1.4744717526707,1.,1.2794891824849));
#25013=CARTESIAN_POINT('Ctrl Pts',(1.47980070347095,-1.,1.28194158939517));
#25014=CARTESIAN_POINT('Ctrl Pts',(1.47980070347095,1.,1.28194158939517));
#25015=CARTESIAN_POINT('Ctrl Pts',(1.4851881711891,-1.,1.28435533880201));
#25016=CARTESIAN_POINT('Ctrl Pts',(1.4851881711891,1.,1.28435533880201));
#25017=CARTESIAN_POINT('Ctrl Pts',(1.4906522831278,-1.,1.2867467611644));
#25018=CARTESIAN_POINT('Ctrl Pts',(1.4906522831278,1.,1.2867467611644));
#25019=CARTESIAN_POINT('Ctrl Pts',(1.49618896881754,-1.,1.28911506584254));
#25020=CARTESIAN_POINT('Ctrl Pts',(1.49618896881754,1.,1.28911506584254));
#25021=CARTESIAN_POINT('Ctrl Pts',(1.50178230149776,-1.,1.29145022885181));
#25022=CARTESIAN_POINT('Ctrl Pts',(1.50178230149776,1.,1.29145022885181));
#25023=CARTESIAN_POINT('Ctrl Pts',(1.50741159078365,-1.,1.29373841372842));
#25024=CARTESIAN_POINT('Ctrl Pts',(1.50741159078365,1.,1.29373841372842));
#25025=CARTESIAN_POINT('Ctrl Pts',(1.51305994241402,-1.,1.29596850710509));
#25026=CARTESIAN_POINT('Ctrl Pts',(1.51305994241402,1.,1.29596850710509));
#25027=CARTESIAN_POINT('Ctrl Pts',(1.51872184912724,-1.,1.29813791800747));
#25028=CARTESIAN_POINT('Ctrl Pts',(1.51872184912724,1.,1.29813791800747));
#25029=CARTESIAN_POINT('Ctrl Pts',(1.52439957861062,-1.,1.30024984366328));
#25030=CARTESIAN_POINT('Ctrl Pts',(1.52439957861062,1.,1.30024984366328));
#25031=CARTESIAN_POINT('Ctrl Pts',(1.53009970283891,-1.,1.30231064395568));
#25032=CARTESIAN_POINT('Ctrl Pts',(1.53009970283891,1.,1.30231064395568));
#25033=CARTESIAN_POINT('Ctrl Pts',(1.53582981268977,-1.,1.30432735639489));
#25034=CARTESIAN_POINT('Ctrl Pts',(1.53582981268977,1.,1.30432735639489));
#25035=CARTESIAN_POINT('Ctrl Pts',(1.54159462645432,-1.,1.30630475189556));
#25036=CARTESIAN_POINT('Ctrl Pts',(1.54159462645432,1.,1.30630475189556));
#25037=CARTESIAN_POINT('Ctrl Pts',(1.54739413957185,-1.,1.30824393907473));
#25038=CARTESIAN_POINT('Ctrl Pts',(1.54739413957185,1.,1.30824393907473));
#25039=CARTESIAN_POINT('Ctrl Pts',(1.55322568759481,-1.,1.31014393684222));
#25040=CARTESIAN_POINT('Ctrl Pts',(1.55322568759481,1.,1.31014393684222));
#25041=CARTESIAN_POINT('Ctrl Pts',(1.55908521254821,-1.,1.31200264341696));
#25042=CARTESIAN_POINT('Ctrl Pts',(1.55908521254821,1.,1.31200264341696));
#25043=CARTESIAN_POINT('Ctrl Pts',(1.56496872402353,-1.,1.31381795281002));
#25044=CARTESIAN_POINT('Ctrl Pts',(1.56496872402353,1.,1.31381795281002));
#25045=CARTESIAN_POINT('Ctrl Pts',(1.57087397835723,-1.,1.31558903860016));
#25046=CARTESIAN_POINT('Ctrl Pts',(1.57087397835723,1.,1.31558903860016));
#25047=CARTESIAN_POINT('Ctrl Pts',(1.5768005650559,-1.,1.31731642317187));
#25048=CARTESIAN_POINT('Ctrl Pts',(1.5768005650559,1.,1.31731642317187));
#25049=CARTESIAN_POINT('Ctrl Pts',(1.58274907898834,-1.,1.31900135021432));
#25050=CARTESIAN_POINT('Ctrl Pts',(1.58274907898834,1.,1.31900135021432));
#25051=CARTESIAN_POINT('Ctrl Pts',(1.58872057258245,-1.,1.32064537110892));
#25052=CARTESIAN_POINT('Ctrl Pts',(1.58872057258245,1.,1.32064537110892));
#25053=CARTESIAN_POINT('Ctrl Pts',(1.59471591079403,-1.,1.32224985747682));
#25054=CARTESIAN_POINT('Ctrl Pts',(1.59471591079403,1.,1.32224985747682));
#25055=CARTESIAN_POINT('Ctrl Pts',(1.60073511858687,-1.,1.32381550858256));
#25056=CARTESIAN_POINT('Ctrl Pts',(1.60073511858687,1.,1.32381550858256));
#25057=CARTESIAN_POINT('Ctrl Pts',(1.60677758290954,-1.,1.32534250785782));
#25058=CARTESIAN_POINT('Ctrl Pts',(1.60677758290954,1.,1.32534250785782));
#25059=CARTESIAN_POINT('Ctrl Pts',(1.6128423401575,-1.,1.32683074483356));
#25060=CARTESIAN_POINT('Ctrl Pts',(1.6128423401575,1.,1.32683074483356));
#25061=CARTESIAN_POINT('Ctrl Pts',(1.61892832270724,-1.,1.32828000610449));
#25062=CARTESIAN_POINT('Ctrl Pts',(1.61892832270724,1.,1.32828000610449));
#25063=CARTESIAN_POINT('Ctrl Pts',(1.62503464209797,-1.,1.3296901950568));
#25064=CARTESIAN_POINT('Ctrl Pts',(1.62503464209797,1.,1.3296901950568));
#25065=CARTESIAN_POINT('Ctrl Pts',(1.63116079730923,-1.,1.33106149345645));
#25066=CARTESIAN_POINT('Ctrl Pts',(1.63116079730923,1.,1.33106149345645));
#25067=CARTESIAN_POINT('Ctrl Pts',(1.63730653475089,-1.,1.33239425103724));
#25068=CARTESIAN_POINT('Ctrl Pts',(1.63730653475089,1.,1.33239425103724));
#25069=CARTESIAN_POINT('Ctrl Pts',(1.6434717485603,-1.,1.33368890676572));
#25070=CARTESIAN_POINT('Ctrl Pts',(1.6434717485603,1.,1.33368890676572));
#25071=CARTESIAN_POINT('Ctrl Pts',(1.6496563728683,-1.,1.33494590467993));
#25072=CARTESIAN_POINT('Ctrl Pts',(1.6496563728683,1.,1.33494590467993));
#25073=CARTESIAN_POINT('Ctrl Pts',(1.65586025952593,-1.,1.33616559745172));
#25074=CARTESIAN_POINT('Ctrl Pts',(1.65586025952593,1.,1.33616559745172));
#25075=CARTESIAN_POINT('Ctrl Pts',(1.66208312541983,-1.,1.33734820885262));
#25076=CARTESIAN_POINT('Ctrl Pts',(1.66208312541983,1.,1.33734820885262));
#25077=CARTESIAN_POINT('Ctrl Pts',(1.66832460783989,-1.,1.33849388654388));
#25078=CARTESIAN_POINT('Ctrl Pts',(1.66832460783989,1.,1.33849388654388));
#25079=CARTESIAN_POINT('Ctrl Pts',(1.67458429426086,-1.,1.3396027347034));
#25080=CARTESIAN_POINT('Ctrl Pts',(1.67458429426086,1.,1.3396027347034));
#25081=CARTESIAN_POINT('Ctrl Pts',(1.68086176030362,-1.,1.34067485185203));
#25082=CARTESIAN_POINT('Ctrl Pts',(1.68086176030362,1.,1.34067485185203));
#25083=CARTESIAN_POINT('Ctrl Pts',(1.68715660868764,-1.,1.341710374848));
#25084=CARTESIAN_POINT('Ctrl Pts',(1.68715660868764,1.,1.341710374848));
#25085=CARTESIAN_POINT('Ctrl Pts',(1.6934684849687,-1.,1.34270948206319));
#25086=CARTESIAN_POINT('Ctrl Pts',(1.6934684849687,1.,1.34270948206319));
#25087=CARTESIAN_POINT('Ctrl Pts',(1.69979707754427,-1.,1.34367237124483));
#25088=CARTESIAN_POINT('Ctrl Pts',(1.69979707754427,1.,1.34367237124483));
#25089=CARTESIAN_POINT('Ctrl Pts',(1.70614212266738,-1.,1.34459924533831));
#25090=CARTESIAN_POINT('Ctrl Pts',(1.70614212266738,1.,1.34459924533831));
#25091=CARTESIAN_POINT('Ctrl Pts',(1.71250340686822,-1.,1.34549029589416));
#25092=CARTESIAN_POINT('Ctrl Pts',(1.71250340686822,1.,1.34549029589416));
#25093=CARTESIAN_POINT('Ctrl Pts',(1.7188807715049,-1.,1.34634568653227));
#25094=CARTESIAN_POINT('Ctrl Pts',(1.7188807715049,1.,1.34634568653227));
#25095=CARTESIAN_POINT('Ctrl Pts',(1.72527410680674,-1.,1.34716554819527));
#25096=CARTESIAN_POINT('Ctrl Pts',(1.72527410680674,1.,1.34716554819527));
#25097=CARTESIAN_POINT('Ctrl Pts',(1.7304014965394,-1.,1.34779309152035));
#25098=CARTESIAN_POINT('Ctrl Pts',(1.7304014965394,1.,1.34779309152035));
#25099=CARTESIAN_POINT('Ctrl Pts',(1.73425417885907,-1.,1.34824783112887));
#25100=CARTESIAN_POINT('Ctrl Pts',(1.73425417885907,1.,1.34824783112887));
#25101=CARTESIAN_POINT('Ctrl Pts',(1.73682580585691,-1.,1.34854391898045));
#25102=CARTESIAN_POINT('Ctrl Pts',(1.73682580585691,1.,1.34854391898045));
#25103=CARTESIAN_POINT('Ctrl Pts',(1.73811241238545,-1.,1.34869019493419));
#25104=CARTESIAN_POINT('Ctrl Pts',(1.73811241238545,1.,1.34869019493419));
#25105=CARTESIAN_POINT('',(1.31362392696032,1.,1.15624053661742));
#25106=CARTESIAN_POINT('Ctrl Pts',(1.31362392696032,1.,1.15624053661742));
#25107=CARTESIAN_POINT('Ctrl Pts',(1.31722977216397,1.,1.15950888730809));
#25108=CARTESIAN_POINT('Ctrl Pts',(1.32428080721772,1.,1.16589330093588));
#25109=CARTESIAN_POINT('Ctrl Pts',(1.33437539347008,1.,1.17501305789857));
#25110=CARTESIAN_POINT('Ctrl Pts',(1.34687054001093,1.,1.18625865667441));
#25111=CARTESIAN_POINT('Ctrl Pts',(1.36088705043885,1.,1.1987959077932));
#25112=CARTESIAN_POINT('Ctrl Pts',(1.37331915607905,1.,1.20982812925645));
#25113=CARTESIAN_POINT('Ctrl Pts',(1.38420564527715,1.,1.21938737280852));
#25114=CARTESIAN_POINT('Ctrl Pts',(1.39361389568796,1.,1.22752961899387));
#25115=CARTESIAN_POINT('Ctrl Pts',(1.40164708206106,1.,1.23434087290423));
#25116=CARTESIAN_POINT('Ctrl Pts',(1.40845295531283,1.,1.23994455029534));
#25117=CARTESIAN_POINT('Ctrl Pts',(1.41422913175179,1.,1.24450600513056));
#25118=CARTESIAN_POINT('Ctrl Pts',(1.41923722596025,1.,1.24824430986571));
#25119=CARTESIAN_POINT('Ctrl Pts',(1.42378102115575,1.,1.2514145557001));
#25120=CARTESIAN_POINT('Ctrl Pts',(1.42815938799387,1.,1.25426945222639));
#25121=CARTESIAN_POINT('Ctrl Pts',(1.43262645609691,1.,1.25702687965755));
#25122=CARTESIAN_POINT('Ctrl Pts',(1.43734919180847,1.,1.25983531012005));
#25123=CARTESIAN_POINT('Ctrl Pts',(1.44236470511303,1.,1.26273903323859));
#25124=CARTESIAN_POINT('Ctrl Pts',(1.44761985001662,1.,1.26570925118868));
#25125=CARTESIAN_POINT('Ctrl Pts',(1.45301422764247,1.,1.2686778680489));
#25126=CARTESIAN_POINT('Ctrl Pts',(1.45843906294697,1.,1.27156805265289));
#25127=CARTESIAN_POINT('Ctrl Pts',(1.46382431332476,1.,1.27433119897822));
#25128=CARTESIAN_POINT('Ctrl Pts',(1.46916035917133,1.,1.2769641483109));
#25129=CARTESIAN_POINT('Ctrl Pts',(1.4744717526707,1.,1.2794891824849));
#25130=CARTESIAN_POINT('Ctrl Pts',(1.47980070347095,1.,1.28194158939517));
#25131=CARTESIAN_POINT('Ctrl Pts',(1.4851881711891,1.,1.28435533880201));
#25132=CARTESIAN_POINT('Ctrl Pts',(1.4906522831278,1.,1.2867467611644));
#25133=CARTESIAN_POINT('Ctrl Pts',(1.49618896881754,1.,1.28911506584254));
#25134=CARTESIAN_POINT('Ctrl Pts',(1.50178230149776,1.,1.29145022885181));
#25135=CARTESIAN_POINT('Ctrl Pts',(1.50741159078365,1.,1.29373841372842));
#25136=CARTESIAN_POINT('Ctrl Pts',(1.51305994241402,1.,1.29596850710509));
#25137=CARTESIAN_POINT('Ctrl Pts',(1.51872184912724,1.,1.29813791800747));
#25138=CARTESIAN_POINT('Ctrl Pts',(1.52439957861062,1.,1.30024984366328));
#25139=CARTESIAN_POINT('Ctrl Pts',(1.53009970283891,1.,1.30231064395568));
#25140=CARTESIAN_POINT('Ctrl Pts',(1.53582981268977,1.,1.30432735639489));
#25141=CARTESIAN_POINT('Ctrl Pts',(1.54159462645432,1.,1.30630475189556));
#25142=CARTESIAN_POINT('Ctrl Pts',(1.54739413957185,1.,1.30824393907473));
#25143=CARTESIAN_POINT('Ctrl Pts',(1.55322568759481,1.,1.31014393684222));
#25144=CARTESIAN_POINT('Ctrl Pts',(1.55908521254821,1.,1.31200264341696));
#25145=CARTESIAN_POINT('Ctrl Pts',(1.56496872402353,1.,1.31381795281002));
#25146=CARTESIAN_POINT('Ctrl Pts',(1.57087397835723,1.,1.31558903860016));
#25147=CARTESIAN_POINT('Ctrl Pts',(1.5768005650559,1.,1.31731642317187));
#25148=CARTESIAN_POINT('Ctrl Pts',(1.58274907898834,1.,1.31900135021432));
#25149=CARTESIAN_POINT('Ctrl Pts',(1.58872057258245,1.,1.32064537110892));
#25150=CARTESIAN_POINT('Ctrl Pts',(1.59471591079403,1.,1.32224985747682));
#25151=CARTESIAN_POINT('Ctrl Pts',(1.60073511858687,1.,1.32381550858256));
#25152=CARTESIAN_POINT('Ctrl Pts',(1.60677758290954,1.,1.32534250785782));
#25153=CARTESIAN_POINT('Ctrl Pts',(1.6128423401575,1.,1.32683074483356));
#25154=CARTESIAN_POINT('Ctrl Pts',(1.61892832270724,1.,1.32828000610449));
#25155=CARTESIAN_POINT('Ctrl Pts',(1.62503464209797,1.,1.3296901950568));
#25156=CARTESIAN_POINT('Ctrl Pts',(1.63116079730923,1.,1.33106149345645));
#25157=CARTESIAN_POINT('Ctrl Pts',(1.63730653475089,1.,1.33239425103724));
#25158=CARTESIAN_POINT('Ctrl Pts',(1.6434717485603,1.,1.33368890676572));
#25159=CARTESIAN_POINT('Ctrl Pts',(1.6496563728683,1.,1.33494590467993));
#25160=CARTESIAN_POINT('Ctrl Pts',(1.65586025952593,1.,1.33616559745172));
#25161=CARTESIAN_POINT('Ctrl Pts',(1.66208312541983,1.,1.33734820885262));
#25162=CARTESIAN_POINT('Ctrl Pts',(1.66832460783989,1.,1.33849388654388));
#25163=CARTESIAN_POINT('Ctrl Pts',(1.67458429426086,1.,1.3396027347034));
#25164=CARTESIAN_POINT('Ctrl Pts',(1.68086176030362,1.,1.34067485185203));
#25165=CARTESIAN_POINT('Ctrl Pts',(1.68715660868764,1.,1.341710374848));
#25166=CARTESIAN_POINT('Ctrl Pts',(1.6934684849687,1.,1.34270948206319));
#25167=CARTESIAN_POINT('Ctrl Pts',(1.69979707754427,1.,1.34367237124483));
#25168=CARTESIAN_POINT('Ctrl Pts',(1.70614212266738,1.,1.34459924533831));
#25169=CARTESIAN_POINT('Ctrl Pts',(1.71250340686822,1.,1.34549029589416));
#25170=CARTESIAN_POINT('Ctrl Pts',(1.7188807715049,1.,1.34634568653227));
#25171=CARTESIAN_POINT('Ctrl Pts',(1.72527410680674,1.,1.34716554819527));
#25172=CARTESIAN_POINT('Ctrl Pts',(1.7304014965394,1.,1.34779309152035));
#25173=CARTESIAN_POINT('Ctrl Pts',(1.73425417885907,1.,1.34824783112887));
#25174=CARTESIAN_POINT('Ctrl Pts',(1.73682580585691,1.,1.34854391898045));
#25175=CARTESIAN_POINT('Ctrl Pts',(1.73811241238545,1.,1.34869019493419));
#25176=CARTESIAN_POINT('',(1.31362392696032,0.,1.15624053661742));
#25177=CARTESIAN_POINT('Origin',(0.,0.,0.));
#25178=CARTESIAN_POINT('',(1.15624053661742,1.,1.31362392696033));
#25179=CARTESIAN_POINT('Origin',(0.,1.,0.));
#25180=CARTESIAN_POINT('',(1.15624053661742,0.,1.31362392696032));
#25181=CARTESIAN_POINT('Ctrl Pts',(1.34869019493419,-1.,1.73811241238545));
#25182=CARTESIAN_POINT('Ctrl Pts',(1.34869019493419,1.,1.73811241238545));
#25183=CARTESIAN_POINT('Ctrl Pts',(1.34854391898145,-1.,1.73682580585819));
#25184=CARTESIAN_POINT('Ctrl Pts',(1.34854391898145,1.,1.73682580585819));
#25185=CARTESIAN_POINT('Ctrl Pts',(1.34824783113158,-1.,1.73425417886255));
#25186=CARTESIAN_POINT('Ctrl Pts',(1.34824783113158,1.,1.73425417886255));
#25187=CARTESIAN_POINT('Ctrl Pts',(1.3477930915247,-1.,1.73040149654497));
#25188=CARTESIAN_POINT('Ctrl Pts',(1.3477930915247,1.,1.73040149654497));
#25189=CARTESIAN_POINT('Ctrl Pts',(1.34716554820013,-1.,1.72527410681298));
#25190=CARTESIAN_POINT('Ctrl Pts',(1.34716554820013,1.,1.72527410681298));
#25191=CARTESIAN_POINT('Ctrl Pts',(1.34634568653586,-1.,1.7188807715095));
#25192=CARTESIAN_POINT('Ctrl Pts',(1.34634568653586,1.,1.7188807715095));
#25193=CARTESIAN_POINT('Ctrl Pts',(1.34549029589563,-1.,1.71250340687011));
#25194=CARTESIAN_POINT('Ctrl Pts',(1.34549029589563,1.,1.71250340687011));
#25195=CARTESIAN_POINT('Ctrl Pts',(1.34459924533783,-1.,1.70614212266676));
#25196=CARTESIAN_POINT('Ctrl Pts',(1.34459924533783,1.,1.70614212266676));
#25197=CARTESIAN_POINT('Ctrl Pts',(1.34367237124322,-1.,1.69979707754221));
#25198=CARTESIAN_POINT('Ctrl Pts',(1.34367237124322,1.,1.69979707754221));
#25199=CARTESIAN_POINT('Ctrl Pts',(1.34270948206139,-1.,1.6934684849664));
#25200=CARTESIAN_POINT('Ctrl Pts',(1.34270948206139,1.,1.6934684849664));
#25201=CARTESIAN_POINT('Ctrl Pts',(1.34171037484673,-1.,1.68715660868602));
#25202=CARTESIAN_POINT('Ctrl Pts',(1.34171037484673,1.,1.68715660868602));
#25203=CARTESIAN_POINT('Ctrl Pts',(1.3406748518516,-1.,1.68086176030308));
#25204=CARTESIAN_POINT('Ctrl Pts',(1.3406748518516,1.,1.68086176030308));
#25205=CARTESIAN_POINT('Ctrl Pts',(1.33960273470372,-1.,1.67458429426126));
#25206=CARTESIAN_POINT('Ctrl Pts',(1.33960273470372,1.,1.67458429426126));
#25207=CARTESIAN_POINT('Ctrl Pts',(1.33849388654458,-1.,1.66832460784078));
#25208=CARTESIAN_POINT('Ctrl Pts',(1.33849388654458,1.,1.66832460784078));
#25209=CARTESIAN_POINT('Ctrl Pts',(1.33734820885331,-1.,1.66208312542073));
#25210=CARTESIAN_POINT('Ctrl Pts',(1.33734820885331,1.,1.66208312542073));
#25211=CARTESIAN_POINT('Ctrl Pts',(1.33616559745217,-1.,1.65586025952651));
#25212=CARTESIAN_POINT('Ctrl Pts',(1.33616559745217,1.,1.65586025952651));
#25213=CARTESIAN_POINT('Ctrl Pts',(1.33494590468003,-1.,1.64965637286843));
#25214=CARTESIAN_POINT('Ctrl Pts',(1.33494590468003,1.,1.64965637286843));
#25215=CARTESIAN_POINT('Ctrl Pts',(1.33368890676554,-1.,1.64347174856007));
#25216=CARTESIAN_POINT('Ctrl Pts',(1.33368890676554,1.,1.64347174856007));
#25217=CARTESIAN_POINT('Ctrl Pts',(1.33239425103694,-1.,1.6373065347505));
#25218=CARTESIAN_POINT('Ctrl Pts',(1.33239425103694,1.,1.6373065347505));
#25219=CARTESIAN_POINT('Ctrl Pts',(1.33106149345618,-1.,1.63116079730887));
#25220=CARTESIAN_POINT('Ctrl Pts',(1.33106149345618,1.,1.63116079730887));
#25221=CARTESIAN_POINT('Ctrl Pts',(1.32969019505665,-1.,1.62503464209777));
#25222=CARTESIAN_POINT('Ctrl Pts',(1.32969019505665,1.,1.62503464209777));
#25223=CARTESIAN_POINT('Ctrl Pts',(1.32828000610448,-1.,1.61892832270723));
#25224=CARTESIAN_POINT('Ctrl Pts',(1.32828000610448,1.,1.61892832270723));
#25225=CARTESIAN_POINT('Ctrl Pts',(1.32683074483365,-1.,1.61284234015762));
#25226=CARTESIAN_POINT('Ctrl Pts',(1.32683074483365,1.,1.61284234015762));
#25227=CARTESIAN_POINT('Ctrl Pts',(1.32534250785794,-1.,1.6067775829097));
#25228=CARTESIAN_POINT('Ctrl Pts',(1.32534250785794,1.,1.6067775829097));
#25229=CARTESIAN_POINT('Ctrl Pts',(1.32381550858266,-1.,1.600735118587));
#25230=CARTESIAN_POINT('Ctrl Pts',(1.32381550858266,1.,1.600735118587));
#25231=CARTESIAN_POINT('Ctrl Pts',(1.32224985747686,-1.,1.59471591079408));
#25232=CARTESIAN_POINT('Ctrl Pts',(1.32224985747686,1.,1.59471591079408));
#25233=CARTESIAN_POINT('Ctrl Pts',(1.32064537110891,-1.,1.58872057258244));
#25234=CARTESIAN_POINT('Ctrl Pts',(1.32064537110891,1.,1.58872057258244));
#25235=CARTESIAN_POINT('Ctrl Pts',(1.31900135021428,-1.,1.58274907898829));
#25236=CARTESIAN_POINT('Ctrl Pts',(1.31900135021428,1.,1.58274907898829));
#25237=CARTESIAN_POINT('Ctrl Pts',(1.31731642317183,-1.,1.57680056505585));
#25238=CARTESIAN_POINT('Ctrl Pts',(1.31731642317183,1.,1.57680056505585));
#25239=CARTESIAN_POINT('Ctrl Pts',(1.31558903860015,-1.,1.57087397835721));
#25240=CARTESIAN_POINT('Ctrl Pts',(1.31558903860015,1.,1.57087397835721));
#25241=CARTESIAN_POINT('Ctrl Pts',(1.31381795281002,-1.,1.56496872402352));
#25242=CARTESIAN_POINT('Ctrl Pts',(1.31381795281002,1.,1.56496872402352));
#25243=CARTESIAN_POINT('Ctrl Pts',(1.31200264341696,-1.,1.55908521254822));
#25244=CARTESIAN_POINT('Ctrl Pts',(1.31200264341696,1.,1.55908521254822));
#25245=CARTESIAN_POINT('Ctrl Pts',(1.31014393684221,-1.,1.55322568759481));
#25246=CARTESIAN_POINT('Ctrl Pts',(1.31014393684221,1.,1.55322568759481));
#25247=CARTESIAN_POINT('Ctrl Pts',(1.30824393907471,-1.,1.54739413957183));
#25248=CARTESIAN_POINT('Ctrl Pts',(1.30824393907471,1.,1.54739413957183));
#25249=CARTESIAN_POINT('Ctrl Pts',(1.30630475189553,-1.,1.54159462645428));
#25250=CARTESIAN_POINT('Ctrl Pts',(1.30630475189553,1.,1.54159462645428));
#25251=CARTESIAN_POINT('Ctrl Pts',(1.30432735639487,-1.,1.53582981268976));
#25252=CARTESIAN_POINT('Ctrl Pts',(1.30432735639487,1.,1.53582981268976));
#25253=CARTESIAN_POINT('Ctrl Pts',(1.3023106439557,-1.,1.53009970283893));
#25254=CARTESIAN_POINT('Ctrl Pts',(1.3023106439557,1.,1.53009970283893));
#25255=CARTESIAN_POINT('Ctrl Pts',(1.30024984366334,-1.,1.5243995786107));
#25256=CARTESIAN_POINT('Ctrl Pts',(1.30024984366334,1.,1.5243995786107));
#25257=CARTESIAN_POINT('Ctrl Pts',(1.29813791800757,-1.,1.51872184912735));
#25258=CARTESIAN_POINT('Ctrl Pts',(1.29813791800757,1.,1.51872184912735));
#25259=CARTESIAN_POINT('Ctrl Pts',(1.29596850710518,-1.,1.51305994241412));
#25260=CARTESIAN_POINT('Ctrl Pts',(1.29596850710518,1.,1.51305994241412));
#25261=CARTESIAN_POINT('Ctrl Pts',(1.29373841372843,-1.,1.50741159078367));
#25262=CARTESIAN_POINT('Ctrl Pts',(1.29373841372843,1.,1.50741159078367));
#25263=CARTESIAN_POINT('Ctrl Pts',(1.29145022885171,-1.,1.50178230149764));
#25264=CARTESIAN_POINT('Ctrl Pts',(1.29145022885171,1.,1.50178230149764));
#25265=CARTESIAN_POINT('Ctrl Pts',(1.28911506584232,-1.,1.49618896881729));
#25266=CARTESIAN_POINT('Ctrl Pts',(1.28911506584232,1.,1.49618896881729));
#25267=CARTESIAN_POINT('Ctrl Pts',(1.28674676116415,-1.,1.4906522831275));
#25268=CARTESIAN_POINT('Ctrl Pts',(1.28674676116415,1.,1.4906522831275));
#25269=CARTESIAN_POINT('Ctrl Pts',(1.28435533880184,-1.,1.48518817118891));
#25270=CARTESIAN_POINT('Ctrl Pts',(1.28435533880184,1.,1.48518817118891));
#25271=CARTESIAN_POINT('Ctrl Pts',(1.28194158939522,-1.,1.47980070347102));
#25272=CARTESIAN_POINT('Ctrl Pts',(1.28194158939522,1.,1.47980070347102));
#25273=CARTESIAN_POINT('Ctrl Pts',(1.27948918248524,-1.,1.4744717526711));
#25274=CARTESIAN_POINT('Ctrl Pts',(1.27948918248524,1.,1.4744717526711));
#25275=CARTESIAN_POINT('Ctrl Pts',(1.27696414831144,-1.,1.46916035917197));
#25276=CARTESIAN_POINT('Ctrl Pts',(1.27696414831144,1.,1.46916035917197));
#25277=CARTESIAN_POINT('Ctrl Pts',(1.27433119897877,-1.,1.4638243133254));
#25278=CARTESIAN_POINT('Ctrl Pts',(1.27433119897877,1.,1.4638243133254));
#25279=CARTESIAN_POINT('Ctrl Pts',(1.27156805265312,-1.,1.45843906294725));
#25280=CARTESIAN_POINT('Ctrl Pts',(1.27156805265312,1.,1.45843906294725));
#25281=CARTESIAN_POINT('Ctrl Pts',(1.26867786804854,-1.,1.45301422764205));
#25282=CARTESIAN_POINT('Ctrl Pts',(1.26867786804854,1.,1.45301422764205));
#25283=CARTESIAN_POINT('Ctrl Pts',(1.26570925118767,-1.,1.44761985001544));
#25284=CARTESIAN_POINT('Ctrl Pts',(1.26570925118767,1.,1.44761985001544));
#25285=CARTESIAN_POINT('Ctrl Pts',(1.26273903323723,-1.,1.44236470511145));
#25286=CARTESIAN_POINT('Ctrl Pts',(1.26273903323723,1.,1.44236470511145));
#25287=CARTESIAN_POINT('Ctrl Pts',(1.25983531011894,-1.,1.43734919180719));
#25288=CARTESIAN_POINT('Ctrl Pts',(1.25983531011894,1.,1.43734919180719));
#25289=CARTESIAN_POINT('Ctrl Pts',(1.25702687965744,-1.,1.43262645609679));
#25290=CARTESIAN_POINT('Ctrl Pts',(1.25702687965744,1.,1.43262645609679));
#25291=CARTESIAN_POINT('Ctrl Pts',(1.25426945222783,-1.,1.42815938799555));
#25292=CARTESIAN_POINT('Ctrl Pts',(1.25426945222783,1.,1.42815938799555));
#25293=CARTESIAN_POINT('Ctrl Pts',(1.25141455570299,-1.,1.42378102115911));
#25294=CARTESIAN_POINT('Ctrl Pts',(1.25141455570299,1.,1.42378102115911));
#25295=CARTESIAN_POINT('Ctrl Pts',(1.24824430986911,-1.,1.41923722596421));
#25296=CARTESIAN_POINT('Ctrl Pts',(1.24824430986911,1.,1.41923722596421));
#25297=CARTESIAN_POINT('Ctrl Pts',(1.24450600513278,-1.,1.41422913175437));
#25298=CARTESIAN_POINT('Ctrl Pts',(1.24450600513278,1.,1.41422913175437));
#25299=CARTESIAN_POINT('Ctrl Pts',(1.23994455029421,-1.,1.40845295531151));
#25300=CARTESIAN_POINT('Ctrl Pts',(1.23994455029421,1.,1.40845295531151));
#25301=CARTESIAN_POINT('Ctrl Pts',(1.23434087289768,-1.,1.40164708205345));
#25302=CARTESIAN_POINT('Ctrl Pts',(1.23434087289768,1.,1.40164708205345));
#25303=CARTESIAN_POINT('Ctrl Pts',(1.22752961898063,-1.,1.39361389567257));
#25304=CARTESIAN_POINT('Ctrl Pts',(1.22752961898063,1.,1.39361389567257));
#25305=CARTESIAN_POINT('Ctrl Pts',(1.21938737278853,-1.,1.38420564525391));
#25306=CARTESIAN_POINT('Ctrl Pts',(1.21938737278853,1.,1.38420564525391));
#25307=CARTESIAN_POINT('Ctrl Pts',(1.20982812923113,-1.,1.37331915604962));
#25308=CARTESIAN_POINT('Ctrl Pts',(1.20982812923113,1.,1.37331915604962));
#25309=CARTESIAN_POINT('Ctrl Pts',(1.1987959077656,-1.,1.36088705040677));
#25310=CARTESIAN_POINT('Ctrl Pts',(1.1987959077656,1.,1.36088705040677));
#25311=CARTESIAN_POINT('Ctrl Pts',(1.18625865664915,-1.,1.34687053998157));
#25312=CARTESIAN_POINT('Ctrl Pts',(1.18625865664915,1.,1.34687053998157));
#25313=CARTESIAN_POINT('Ctrl Pts',(1.17501305787994,-1.,1.33437539344842));
#25314=CARTESIAN_POINT('Ctrl Pts',(1.17501305787994,1.,1.33437539344842));
#25315=CARTESIAN_POINT('Ctrl Pts',(1.16589330092532,-1.,1.32428080720544));
#25316=CARTESIAN_POINT('Ctrl Pts',(1.16589330092532,1.,1.32428080720544));
#25317=CARTESIAN_POINT('Ctrl Pts',(1.15950888730433,-1.,1.3172297721596));
#25318=CARTESIAN_POINT('Ctrl Pts',(1.15950888730433,1.,1.3172297721596));
#25319=CARTESIAN_POINT('Ctrl Pts',(1.15624053661742,-1.,1.31362392696033));
#25320=CARTESIAN_POINT('Ctrl Pts',(1.15624053661742,1.,1.31362392696033));
#25321=CARTESIAN_POINT('',(1.34869019493419,1.,1.73811241238545));
#25322=CARTESIAN_POINT('Ctrl Pts',(1.34869019493419,1.,1.73811241238545));
#25323=CARTESIAN_POINT('Ctrl Pts',(1.34854391898145,1.,1.73682580585819));
#25324=CARTESIAN_POINT('Ctrl Pts',(1.34824783113158,1.,1.73425417886255));
#25325=CARTESIAN_POINT('Ctrl Pts',(1.3477930915247,1.,1.73040149654497));
#25326=CARTESIAN_POINT('Ctrl Pts',(1.34716554820013,1.,1.72527410681298));
#25327=CARTESIAN_POINT('Ctrl Pts',(1.34634568653586,1.,1.7188807715095));
#25328=CARTESIAN_POINT('Ctrl Pts',(1.34549029589563,1.,1.71250340687011));
#25329=CARTESIAN_POINT('Ctrl Pts',(1.34459924533783,1.,1.70614212266676));
#25330=CARTESIAN_POINT('Ctrl Pts',(1.34367237124322,1.,1.69979707754221));
#25331=CARTESIAN_POINT('Ctrl Pts',(1.34270948206139,1.,1.6934684849664));
#25332=CARTESIAN_POINT('Ctrl Pts',(1.34171037484673,1.,1.68715660868602));
#25333=CARTESIAN_POINT('Ctrl Pts',(1.3406748518516,1.,1.68086176030308));
#25334=CARTESIAN_POINT('Ctrl Pts',(1.33960273470372,1.,1.67458429426126));
#25335=CARTESIAN_POINT('Ctrl Pts',(1.33849388654458,1.,1.66832460784078));
#25336=CARTESIAN_POINT('Ctrl Pts',(1.33734820885331,1.,1.66208312542073));
#25337=CARTESIAN_POINT('Ctrl Pts',(1.33616559745217,1.,1.65586025952651));
#25338=CARTESIAN_POINT('Ctrl Pts',(1.33494590468003,1.,1.64965637286843));
#25339=CARTESIAN_POINT('Ctrl Pts',(1.33368890676554,1.,1.64347174856007));
#25340=CARTESIAN_POINT('Ctrl Pts',(1.33239425103694,1.,1.6373065347505));
#25341=CARTESIAN_POINT('Ctrl Pts',(1.33106149345618,1.,1.63116079730887));
#25342=CARTESIAN_POINT('Ctrl Pts',(1.32969019505665,1.,1.62503464209777));
#25343=CARTESIAN_POINT('Ctrl Pts',(1.32828000610448,1.,1.61892832270723));
#25344=CARTESIAN_POINT('Ctrl Pts',(1.32683074483365,1.,1.61284234015762));
#25345=CARTESIAN_POINT('Ctrl Pts',(1.32534250785794,1.,1.6067775829097));
#25346=CARTESIAN_POINT('Ctrl Pts',(1.32381550858266,1.,1.600735118587));
#25347=CARTESIAN_POINT('Ctrl Pts',(1.32224985747686,1.,1.59471591079408));
#25348=CARTESIAN_POINT('Ctrl Pts',(1.32064537110891,1.,1.58872057258244));
#25349=CARTESIAN_POINT('Ctrl Pts',(1.31900135021428,1.,1.58274907898829));
#25350=CARTESIAN_POINT('Ctrl Pts',(1.31731642317183,1.,1.57680056505585));
#25351=CARTESIAN_POINT('Ctrl Pts',(1.31558903860015,1.,1.57087397835721));
#25352=CARTESIAN_POINT('Ctrl Pts',(1.31381795281002,1.,1.56496872402352));
#25353=CARTESIAN_POINT('Ctrl Pts',(1.31200264341696,1.,1.55908521254822));
#25354=CARTESIAN_POINT('Ctrl Pts',(1.31014393684221,1.,1.55322568759481));
#25355=CARTESIAN_POINT('Ctrl Pts',(1.30824393907471,1.,1.54739413957183));
#25356=CARTESIAN_POINT('Ctrl Pts',(1.30630475189553,1.,1.54159462645428));
#25357=CARTESIAN_POINT('Ctrl Pts',(1.30432735639487,1.,1.53582981268976));
#25358=CARTESIAN_POINT('Ctrl Pts',(1.3023106439557,1.,1.53009970283893));
#25359=CARTESIAN_POINT('Ctrl Pts',(1.30024984366334,1.,1.5243995786107));
#25360=CARTESIAN_POINT('Ctrl Pts',(1.29813791800757,1.,1.51872184912735));
#25361=CARTESIAN_POINT('Ctrl Pts',(1.29596850710518,1.,1.51305994241412));
#25362=CARTESIAN_POINT('Ctrl Pts',(1.29373841372843,1.,1.50741159078367));
#25363=CARTESIAN_POINT('Ctrl Pts',(1.29145022885171,1.,1.50178230149764));
#25364=CARTESIAN_POINT('Ctrl Pts',(1.28911506584232,1.,1.49618896881729));
#25365=CARTESIAN_POINT('Ctrl Pts',(1.28674676116415,1.,1.4906522831275));
#25366=CARTESIAN_POINT('Ctrl Pts',(1.28435533880184,1.,1.48518817118891));
#25367=CARTESIAN_POINT('Ctrl Pts',(1.28194158939522,1.,1.47980070347102));
#25368=CARTESIAN_POINT('Ctrl Pts',(1.27948918248524,1.,1.4744717526711));
#25369=CARTESIAN_POINT('Ctrl Pts',(1.27696414831144,1.,1.46916035917197));
#25370=CARTESIAN_POINT('Ctrl Pts',(1.27433119897877,1.,1.4638243133254));
#25371=CARTESIAN_POINT('Ctrl Pts',(1.27156805265312,1.,1.45843906294725));
#25372=CARTESIAN_POINT('Ctrl Pts',(1.26867786804854,1.,1.45301422764205));
#25373=CARTESIAN_POINT('Ctrl Pts',(1.26570925118767,1.,1.44761985001544));
#25374=CARTESIAN_POINT('Ctrl Pts',(1.26273903323723,1.,1.44236470511145));
#25375=CARTESIAN_POINT('Ctrl Pts',(1.25983531011894,1.,1.43734919180719));
#25376=CARTESIAN_POINT('Ctrl Pts',(1.25702687965744,1.,1.43262645609679));
#25377=CARTESIAN_POINT('Ctrl Pts',(1.25426945222783,1.,1.42815938799555));
#25378=CARTESIAN_POINT('Ctrl Pts',(1.25141455570299,1.,1.42378102115911));
#25379=CARTESIAN_POINT('Ctrl Pts',(1.24824430986911,1.,1.41923722596421));
#25380=CARTESIAN_POINT('Ctrl Pts',(1.24450600513278,1.,1.41422913175437));
#25381=CARTESIAN_POINT('Ctrl Pts',(1.23994455029421,1.,1.40845295531151));
#25382=CARTESIAN_POINT('Ctrl Pts',(1.23434087289768,1.,1.40164708205345));
#25383=CARTESIAN_POINT('Ctrl Pts',(1.22752961898063,1.,1.39361389567257));
#25384=CARTESIAN_POINT('Ctrl Pts',(1.21938737278853,1.,1.38420564525391));
#25385=CARTESIAN_POINT('Ctrl Pts',(1.20982812923113,1.,1.37331915604962));
#25386=CARTESIAN_POINT('Ctrl Pts',(1.1987959077656,1.,1.36088705040677));
#25387=CARTESIAN_POINT('Ctrl Pts',(1.18625865664915,1.,1.34687053998157));
#25388=CARTESIAN_POINT('Ctrl Pts',(1.17501305787994,1.,1.33437539344842));
#25389=CARTESIAN_POINT('Ctrl Pts',(1.16589330092532,1.,1.32428080720544));
#25390=CARTESIAN_POINT('Ctrl Pts',(1.15950888730433,1.,1.3172297721596));
#25391=CARTESIAN_POINT('Ctrl Pts',(1.15624053661742,1.,1.31362392696033));
#25392=CARTESIAN_POINT('',(1.34869019493419,0.,1.73811241238545));
#25393=CARTESIAN_POINT('Origin',(1.23627494547115,0.,1.81978687191668));
#25394=CARTESIAN_POINT('',(1.23627494547115,1.,1.81978687191668));
#25395=CARTESIAN_POINT('',(1.34869019493419,1.,1.73811241238545));
#25396=CARTESIAN_POINT('',(1.23627494547115,0.,1.81978687191668));
#25397=CARTESIAN_POINT('Ctrl Pts',(0.892032620296855,-1.,1.5055822144029));
#25398=CARTESIAN_POINT('Ctrl Pts',(0.892032620296855,1.,1.5055822144029));
#25399=CARTESIAN_POINT('Ctrl Pts',(0.894452006967538,-1.,1.50980486807181));
#25400=CARTESIAN_POINT('Ctrl Pts',(0.894452006967538,1.,1.50980486807181));
#25401=CARTESIAN_POINT('Ctrl Pts',(0.89918504749193,-1.,1.51805569591479));
#25402=CARTESIAN_POINT('Ctrl Pts',(0.89918504749193,1.,1.51805569591479));
#25403=CARTESIAN_POINT('Ctrl Pts',(0.905967409640498,-1.,1.52984849890434));
#25404=CARTESIAN_POINT('Ctrl Pts',(0.905967409640498,1.,1.52984849890434));
#25405=CARTESIAN_POINT('Ctrl Pts',(0.914375919046579,-1.,1.54440491152808));
#25406=CARTESIAN_POINT('Ctrl Pts',(0.914375919046579,1.,1.54440491152808));
#25407=CARTESIAN_POINT('Ctrl Pts',(0.923832188966322,-1.,1.56065988582509));
#25408=CARTESIAN_POINT('Ctrl Pts',(0.923832188966322,1.,1.56065988582509));
#25409=CARTESIAN_POINT('Ctrl Pts',(0.932246680128848,-1.,1.57499388385561));
#25410=CARTESIAN_POINT('Ctrl Pts',(0.932246680128848,1.,1.57499388385561));
#25411=CARTESIAN_POINT('Ctrl Pts',(0.939646377909319,-1.,1.58744937489796));
#25412=CARTESIAN_POINT('Ctrl Pts',(0.939646377909319,1.,1.58744937489796));
#25413=CARTESIAN_POINT('Ctrl Pts',(0.946078063325795,-1.,1.59810042045408));
#25414=CARTESIAN_POINT('Ctrl Pts',(0.946078063325795,1.,1.59810042045408));
#25415=CARTESIAN_POINT('Ctrl Pts',(0.951613284361247,-1.,1.60706069897794));
#25416=CARTESIAN_POINT('Ctrl Pts',(0.951613284361247,1.,1.60706069897794));
#25417=CARTESIAN_POINT('Ctrl Pts',(0.956354422921572,-1.,1.61449324337233));
#25418=CARTESIAN_POINT('Ctrl Pts',(0.956354422921572,1.,1.61449324337233));
#25419=CARTESIAN_POINT('Ctrl Pts',(0.960438326099958,-1.,1.62061638139929));
#25420=CARTESIAN_POINT('Ctrl Pts',(0.960438326099958,1.,1.62061638139929));
#25421=CARTESIAN_POINT('Ctrl Pts',(0.964046107037821,-1.,1.6257193066974));
#25422=CARTESIAN_POINT('Ctrl Pts',(0.964046107037821,1.,1.6257193066974));
#25423=CARTESIAN_POINT('Ctrl Pts',(0.967387853228041,-1.,1.63013849959083));
#25424=CARTESIAN_POINT('Ctrl Pts',(0.967387853228041,1.,1.63013849959083));
#25425=CARTESIAN_POINT('Ctrl Pts',(0.970669715996356,-1.,1.63420665729609));
#25426=CARTESIAN_POINT('Ctrl Pts',(0.970669715996356,1.,1.63420665729609));
#25427=CARTESIAN_POINT('Ctrl Pts',(0.974066058287501,-1.,1.63820952658157));
#25428=CARTESIAN_POINT('Ctrl Pts',(0.974066058287501,1.,1.63820952658157));
#25429=CARTESIAN_POINT('Ctrl Pts',(0.977689794120296,-1.,1.64233990826831));
#25430=CARTESIAN_POINT('Ctrl Pts',(0.977689794120296,1.,1.64233990826831));
#25431=CARTESIAN_POINT('Ctrl Pts',(0.981562530940574,-1.,1.64665139190834));
#25432=CARTESIAN_POINT('Ctrl Pts',(0.981562530940574,1.,1.64665139190834));
#25433=CARTESIAN_POINT('Ctrl Pts',(0.985642622921626,-1.,1.6511001661277));
#25434=CARTESIAN_POINT('Ctrl Pts',(0.985642622921626,1.,1.6511001661277));
#25435=CARTESIAN_POINT('Ctrl Pts',(0.98985562785445,-1.,1.65559044289746));
#25436=CARTESIAN_POINT('Ctrl Pts',(0.98985562785445,1.,1.65559044289746));
#25437=CARTESIAN_POINT('Ctrl Pts',(0.994121836661115,-1.,1.66001553809916));
#25438=CARTESIAN_POINT('Ctrl Pts',(0.994121836661115,1.,1.66001553809916));
#25439=CARTESIAN_POINT('Ctrl Pts',(0.998389654952317,-1.,1.66430758030304));
#25440=CARTESIAN_POINT('Ctrl Pts',(0.998389654952317,1.,1.66430758030304));
#25441=CARTESIAN_POINT('Ctrl Pts',(1.00265091003682,-1.,1.66846059277231));
#25442=CARTESIAN_POINT('Ctrl Pts',(1.00265091003682,1.,1.66846059277231));
#25443=CARTESIAN_POINT('Ctrl Pts',(1.00692206696387,-1.,1.67250335383248));
#25444=CARTESIAN_POINT('Ctrl Pts',(1.00692206696387,1.,1.67250335383248));
#25445=CARTESIAN_POINT('Ctrl Pts',(1.01123236493507,-1.,1.67648246776457));
#25446=CARTESIAN_POINT('Ctrl Pts',(1.01123236493507,1.,1.67648246776457));
#25447=CARTESIAN_POINT('Ctrl Pts',(1.01561026162786,-1.,1.6804428989482));
#25448=CARTESIAN_POINT('Ctrl Pts',(1.01561026162786,1.,1.6804428989482));
#25449=CARTESIAN_POINT('Ctrl Pts',(1.02006795074222,-1.,1.68440578021739));
#25450=CARTESIAN_POINT('Ctrl Pts',(1.02006795074222,1.,1.68440578021739));
#25451=CARTESIAN_POINT('Ctrl Pts',(1.02460180535272,-1.,1.68836910178475));
#25452=CARTESIAN_POINT('Ctrl Pts',(1.02460180535272,1.,1.68836910178475));
#25453=CARTESIAN_POINT('Ctrl Pts',(1.02919977579155,-1.,1.69231840863471));
#25454=CARTESIAN_POINT('Ctrl Pts',(1.02919977579155,1.,1.69231840863471));
#25455=CARTESIAN_POINT('Ctrl Pts',(1.03384646003587,-1.,1.69623414782769));
#25456=CARTESIAN_POINT('Ctrl Pts',(1.03384646003587,1.,1.69623414782769));
#25457=CARTESIAN_POINT('Ctrl Pts',(1.03852922490782,-1.,1.70010052930951));
#25458=CARTESIAN_POINT('Ctrl Pts',(1.03852922490782,1.,1.70010052930951));
#25459=CARTESIAN_POINT('Ctrl Pts',(1.04324363334546,-1.,1.70391338707969));
#25460=CARTESIAN_POINT('Ctrl Pts',(1.04324363334546,1.,1.70391338707969));
#25461=CARTESIAN_POINT('Ctrl Pts',(1.0479908540499,-1.,1.70767646263641));
#25462=CARTESIAN_POINT('Ctrl Pts',(1.0479908540499,1.,1.70767646263641));
#25463=CARTESIAN_POINT('Ctrl Pts',(1.05277517202853,-1.,1.71139783543986));
#25464=CARTESIAN_POINT('Ctrl Pts',(1.05277517202853,1.,1.71139783543986));
#25465=CARTESIAN_POINT('Ctrl Pts',(1.05760163192481,-1.,1.71508654427022));
#25466=CARTESIAN_POINT('Ctrl Pts',(1.05760163192481,1.,1.71508654427022));
#25467=CARTESIAN_POINT('Ctrl Pts',(1.06247324680649,-1.,1.71874858456908));
#25468=CARTESIAN_POINT('Ctrl Pts',(1.06247324680649,1.,1.71874858456908));
#25469=CARTESIAN_POINT('Ctrl Pts',(1.06738966975463,-1.,1.72238500928456));
#25470=CARTESIAN_POINT('Ctrl Pts',(1.06738966975463,1.,1.72238500928456));
#25471=CARTESIAN_POINT('Ctrl Pts',(1.07234866990252,-1.,1.72599406198489));
#25472=CARTESIAN_POINT('Ctrl Pts',(1.07234866990252,1.,1.72599406198489));
#25473=CARTESIAN_POINT('Ctrl Pts',(1.0773470373727,-1.,1.72957248977424));
#25474=CARTESIAN_POINT('Ctrl Pts',(1.0773470373727,1.,1.72957248977424));
#25475=CARTESIAN_POINT('Ctrl Pts',(1.08238162784749,-1.,1.73311705663407));
#25476=CARTESIAN_POINT('Ctrl Pts',(1.08238162784749,1.,1.73311705663407));
#25477=CARTESIAN_POINT('Ctrl Pts',(1.08745056285429,-1.,1.73662628326093));
#25478=CARTESIAN_POINT('Ctrl Pts',(1.08745056285429,1.,1.73662628326093));
#25479=CARTESIAN_POINT('Ctrl Pts',(1.09255329056496,-1.,1.74010053962252));
#25480=CARTESIAN_POINT('Ctrl Pts',(1.09255329056496,1.,1.74010053962252));
#25481=CARTESIAN_POINT('Ctrl Pts',(1.09768999241229,-1.,1.74354119236212));
#25482=CARTESIAN_POINT('Ctrl Pts',(1.09768999241229,1.,1.74354119236212));
#25483=CARTESIAN_POINT('Ctrl Pts',(1.10286118991144,-1.,1.74695004214924));
#25484=CARTESIAN_POINT('Ctrl Pts',(1.10286118991144,1.,1.74695004214924));
#25485=CARTESIAN_POINT('Ctrl Pts',(1.10806728183003,-1.,1.75032866075914));
#25486=CARTESIAN_POINT('Ctrl Pts',(1.10806728183003,1.,1.75032866075914));
#25487=CARTESIAN_POINT('Ctrl Pts',(1.11330807582542,-1.,1.75367772094617));
#25488=CARTESIAN_POINT('Ctrl Pts',(1.11330807582542,1.,1.75367772094617));
#25489=CARTESIAN_POINT('Ctrl Pts',(1.11858293216752,-1.,1.75699720772089));
#25490=CARTESIAN_POINT('Ctrl Pts',(1.11858293216752,1.,1.75699720772089));
#25491=CARTESIAN_POINT('Ctrl Pts',(1.12389096855078,-1.,1.76028671825084));
#25492=CARTESIAN_POINT('Ctrl Pts',(1.12389096855078,1.,1.76028671825084));
#25493=CARTESIAN_POINT('Ctrl Pts',(1.12923123555076,-1.,1.76354571966171));
#25494=CARTESIAN_POINT('Ctrl Pts',(1.12923123555076,1.,1.76354571966171));
#25495=CARTESIAN_POINT('Ctrl Pts',(1.13460291804634,-1.,1.76677384551883));
#25496=CARTESIAN_POINT('Ctrl Pts',(1.13460291804634,1.,1.76677384551883));
#25497=CARTESIAN_POINT('Ctrl Pts',(1.14000548337,-1.,1.76997111386806));
#25498=CARTESIAN_POINT('Ctrl Pts',(1.14000548337,1.,1.76997111386806));
#25499=CARTESIAN_POINT('Ctrl Pts',(1.14543858226948,-1.,1.77313777896234));
#25500=CARTESIAN_POINT('Ctrl Pts',(1.14543858226948,1.,1.77313777896234));
#25501=CARTESIAN_POINT('Ctrl Pts',(1.15090197841531,-1.,1.77627422557034));
#25502=CARTESIAN_POINT('Ctrl Pts',(1.15090197841531,1.,1.77627422557034));
#25503=CARTESIAN_POINT('Ctrl Pts',(1.15639547194689,-1.,1.77938085564261));
#25504=CARTESIAN_POINT('Ctrl Pts',(1.15639547194689,1.,1.77938085564261));
#25505=CARTESIAN_POINT('Ctrl Pts',(1.16191881298458,-1.,1.78245795880949));
#25506=CARTESIAN_POINT('Ctrl Pts',(1.16191881298458,1.,1.78245795880949));
#25507=CARTESIAN_POINT('Ctrl Pts',(1.16747166312239,-1.,1.78550566040349));
#25508=CARTESIAN_POINT('Ctrl Pts',(1.16747166312239,1.,1.78550566040349));
#25509=CARTESIAN_POINT('Ctrl Pts',(1.17305363177265,-1.,1.78852398877523));
#25510=CARTESIAN_POINT('Ctrl Pts',(1.17305363177265,1.,1.78852398877523));
#25511=CARTESIAN_POINT('Ctrl Pts',(1.17866429440781,-1.,1.79151291552646));
#25512=CARTESIAN_POINT('Ctrl Pts',(1.17866429440781,1.,1.79151291552646));
#25513=CARTESIAN_POINT('Ctrl Pts',(1.18430321697471,-1.,1.79447240321572));
#25514=CARTESIAN_POINT('Ctrl Pts',(1.18430321697471,1.,1.79447240321572));
#25515=CARTESIAN_POINT('Ctrl Pts',(1.1899699793456,-1.,1.79740245923649));
#25516=CARTESIAN_POINT('Ctrl Pts',(1.1899699793456,1.,1.79740245923649));
#25517=CARTESIAN_POINT('Ctrl Pts',(1.19566418930405,-1.,1.80030314370121));
#25518=CARTESIAN_POINT('Ctrl Pts',(1.19566418930405,1.,1.80030314370121));
#25519=CARTESIAN_POINT('Ctrl Pts',(1.2013854893912,-1.,1.8031745483882));
#25520=CARTESIAN_POINT('Ctrl Pts',(1.2013854893912,1.,1.8031745483882));
#25521=CARTESIAN_POINT('Ctrl Pts',(1.20713356605519,-1.,1.80601678480772));
#25522=CARTESIAN_POINT('Ctrl Pts',(1.20713356605519,1.,1.80601678480772));
#25523=CARTESIAN_POINT('Ctrl Pts',(1.2129081570818,-1.,1.80882996916931));
#25524=CARTESIAN_POINT('Ctrl Pts',(1.2129081570818,1.,1.80882996916931));
#25525=CARTESIAN_POINT('Ctrl Pts',(1.2187090610323,-1.,1.81161420806172));
#25526=CARTESIAN_POINT('Ctrl Pts',(1.2187090610323,1.,1.81161420806172));
#25527=CARTESIAN_POINT('Ctrl Pts',(1.22453613304507,-1.,1.81436959209778));
#25528=CARTESIAN_POINT('Ctrl Pts',(1.22453613304507,1.,1.81436959209778));
#25529=CARTESIAN_POINT('Ctrl Pts',(1.22921864890975,-1.,1.81655087183054));
#25530=CARTESIAN_POINT('Ctrl Pts',(1.22921864890975,1.,1.81655087183054));
#25531=CARTESIAN_POINT('Ctrl Pts',(1.23274224526804,-1.,1.81817389920914));
#25532=CARTESIAN_POINT('Ctrl Pts',(1.23274224526804,1.,1.81817389920914));
#25533=CARTESIAN_POINT('Ctrl Pts',(1.23509651170384,-1.,1.81925017193531));
#25534=CARTESIAN_POINT('Ctrl Pts',(1.23509651170384,1.,1.81925017193531));
#25535=CARTESIAN_POINT('Ctrl Pts',(1.23627494547115,-1.,1.81978687191668));
#25536=CARTESIAN_POINT('Ctrl Pts',(1.23627494547115,1.,1.81978687191668));
#25537=CARTESIAN_POINT('',(0.892032620296855,1.,1.5055822144029));
#25538=CARTESIAN_POINT('Ctrl Pts',(0.892032620296855,1.,1.5055822144029));
#25539=CARTESIAN_POINT('Ctrl Pts',(0.894452006967538,1.,1.50980486807181));
#25540=CARTESIAN_POINT('Ctrl Pts',(0.89918504749193,1.,1.51805569591479));
#25541=CARTESIAN_POINT('Ctrl Pts',(0.905967409640498,1.,1.52984849890434));
#25542=CARTESIAN_POINT('Ctrl Pts',(0.914375919046579,1.,1.54440491152808));
#25543=CARTESIAN_POINT('Ctrl Pts',(0.923832188966322,1.,1.56065988582509));
#25544=CARTESIAN_POINT('Ctrl Pts',(0.932246680128848,1.,1.57499388385561));
#25545=CARTESIAN_POINT('Ctrl Pts',(0.939646377909319,1.,1.58744937489796));
#25546=CARTESIAN_POINT('Ctrl Pts',(0.946078063325795,1.,1.59810042045408));
#25547=CARTESIAN_POINT('Ctrl Pts',(0.951613284361247,1.,1.60706069897794));
#25548=CARTESIAN_POINT('Ctrl Pts',(0.956354422921572,1.,1.61449324337233));
#25549=CARTESIAN_POINT('Ctrl Pts',(0.960438326099958,1.,1.62061638139929));
#25550=CARTESIAN_POINT('Ctrl Pts',(0.964046107037821,1.,1.6257193066974));
#25551=CARTESIAN_POINT('Ctrl Pts',(0.967387853228041,1.,1.63013849959083));
#25552=CARTESIAN_POINT('Ctrl Pts',(0.970669715996356,1.,1.63420665729609));
#25553=CARTESIAN_POINT('Ctrl Pts',(0.974066058287501,1.,1.63820952658157));
#25554=CARTESIAN_POINT('Ctrl Pts',(0.977689794120296,1.,1.64233990826831));
#25555=CARTESIAN_POINT('Ctrl Pts',(0.981562530940574,1.,1.64665139190834));
#25556=CARTESIAN_POINT('Ctrl Pts',(0.985642622921626,1.,1.6511001661277));
#25557=CARTESIAN_POINT('Ctrl Pts',(0.98985562785445,1.,1.65559044289746));
#25558=CARTESIAN_POINT('Ctrl Pts',(0.994121836661115,1.,1.66001553809916));
#25559=CARTESIAN_POINT('Ctrl Pts',(0.998389654952317,1.,1.66430758030304));
#25560=CARTESIAN_POINT('Ctrl Pts',(1.00265091003682,1.,1.66846059277231));
#25561=CARTESIAN_POINT('Ctrl Pts',(1.00692206696387,1.,1.67250335383248));
#25562=CARTESIAN_POINT('Ctrl Pts',(1.01123236493507,1.,1.67648246776457));
#25563=CARTESIAN_POINT('Ctrl Pts',(1.01561026162786,1.,1.6804428989482));
#25564=CARTESIAN_POINT('Ctrl Pts',(1.02006795074222,1.,1.68440578021739));
#25565=CARTESIAN_POINT('Ctrl Pts',(1.02460180535272,1.,1.68836910178475));
#25566=CARTESIAN_POINT('Ctrl Pts',(1.02919977579155,1.,1.69231840863471));
#25567=CARTESIAN_POINT('Ctrl Pts',(1.03384646003587,1.,1.69623414782769));
#25568=CARTESIAN_POINT('Ctrl Pts',(1.03852922490782,1.,1.70010052930951));
#25569=CARTESIAN_POINT('Ctrl Pts',(1.04324363334546,1.,1.70391338707969));
#25570=CARTESIAN_POINT('Ctrl Pts',(1.0479908540499,1.,1.70767646263641));
#25571=CARTESIAN_POINT('Ctrl Pts',(1.05277517202853,1.,1.71139783543986));
#25572=CARTESIAN_POINT('Ctrl Pts',(1.05760163192481,1.,1.71508654427022));
#25573=CARTESIAN_POINT('Ctrl Pts',(1.06247324680649,1.,1.71874858456908));
#25574=CARTESIAN_POINT('Ctrl Pts',(1.06738966975463,1.,1.72238500928456));
#25575=CARTESIAN_POINT('Ctrl Pts',(1.07234866990252,1.,1.72599406198489));
#25576=CARTESIAN_POINT('Ctrl Pts',(1.0773470373727,1.,1.72957248977424));
#25577=CARTESIAN_POINT('Ctrl Pts',(1.08238162784749,1.,1.73311705663407));
#25578=CARTESIAN_POINT('Ctrl Pts',(1.08745056285429,1.,1.73662628326093));
#25579=CARTESIAN_POINT('Ctrl Pts',(1.09255329056496,1.,1.74010053962252));
#25580=CARTESIAN_POINT('Ctrl Pts',(1.09768999241229,1.,1.74354119236212));
#25581=CARTESIAN_POINT('Ctrl Pts',(1.10286118991144,1.,1.74695004214924));
#25582=CARTESIAN_POINT('Ctrl Pts',(1.10806728183003,1.,1.75032866075914));
#25583=CARTESIAN_POINT('Ctrl Pts',(1.11330807582542,1.,1.75367772094617));
#25584=CARTESIAN_POINT('Ctrl Pts',(1.11858293216752,1.,1.75699720772089));
#25585=CARTESIAN_POINT('Ctrl Pts',(1.12389096855078,1.,1.76028671825084));
#25586=CARTESIAN_POINT('Ctrl Pts',(1.12923123555076,1.,1.76354571966171));
#25587=CARTESIAN_POINT('Ctrl Pts',(1.13460291804634,1.,1.76677384551883));
#25588=CARTESIAN_POINT('Ctrl Pts',(1.14000548337,1.,1.76997111386806));
#25589=CARTESIAN_POINT('Ctrl Pts',(1.14543858226948,1.,1.77313777896234));
#25590=CARTESIAN_POINT('Ctrl Pts',(1.15090197841531,1.,1.77627422557034));
#25591=CARTESIAN_POINT('Ctrl Pts',(1.15639547194689,1.,1.77938085564261));
#25592=CARTESIAN_POINT('Ctrl Pts',(1.16191881298458,1.,1.78245795880949));
#25593=CARTESIAN_POINT('Ctrl Pts',(1.16747166312239,1.,1.78550566040349));
#25594=CARTESIAN_POINT('Ctrl Pts',(1.17305363177265,1.,1.78852398877523));
#25595=CARTESIAN_POINT('Ctrl Pts',(1.17866429440781,1.,1.79151291552646));
#25596=CARTESIAN_POINT('Ctrl Pts',(1.18430321697471,1.,1.79447240321572));
#25597=CARTESIAN_POINT('Ctrl Pts',(1.1899699793456,1.,1.79740245923649));
#25598=CARTESIAN_POINT('Ctrl Pts',(1.19566418930405,1.,1.80030314370121));
#25599=CARTESIAN_POINT('Ctrl Pts',(1.2013854893912,1.,1.8031745483882));
#25600=CARTESIAN_POINT('Ctrl Pts',(1.20713356605519,1.,1.80601678480772));
#25601=CARTESIAN_POINT('Ctrl Pts',(1.2129081570818,1.,1.80882996916931));
#25602=CARTESIAN_POINT('Ctrl Pts',(1.2187090610323,1.,1.81161420806172));
#25603=CARTESIAN_POINT('Ctrl Pts',(1.22453613304507,1.,1.81436959209778));
#25604=CARTESIAN_POINT('Ctrl Pts',(1.22921864890975,1.,1.81655087183054));
#25605=CARTESIAN_POINT('Ctrl Pts',(1.23274224526804,1.,1.81817389920914));
#25606=CARTESIAN_POINT('Ctrl Pts',(1.23509651170384,1.,1.81925017193531));
#25607=CARTESIAN_POINT('Ctrl Pts',(1.23627494547115,1.,1.81978687191668));
#25608=CARTESIAN_POINT('',(0.892032620296854,0.,1.5055822144029));
#25609=CARTESIAN_POINT('Origin',(0.,0.,0.));
#25610=CARTESIAN_POINT('',(0.693717979106305,1.,1.60662857109684));
#25611=CARTESIAN_POINT('Origin',(0.,1.,0.));
#25612=CARTESIAN_POINT('',(0.693717979106305,0.,1.60662857109684));
#25613=CARTESIAN_POINT('Ctrl Pts',(0.7455743247944,-1.,2.0698113262342));
#25614=CARTESIAN_POINT('Ctrl Pts',(0.7455743247944,1.,2.0698113262342));
#25615=CARTESIAN_POINT('Ctrl Pts',(0.745832791378367,-1.,2.06854248895728));
#25616=CARTESIAN_POINT('Ctrl Pts',(0.745832791378367,1.,2.06854248895728));
#25617=CARTESIAN_POINT('Ctrl Pts',(0.7463458715442,-1.,2.06600523016815));
#25618=CARTESIAN_POINT('Ctrl Pts',(0.7463458715442,1.,2.06600523016815));
#25619=CARTESIAN_POINT('Ctrl Pts',(0.747103932787919,-1.,2.06220058927826));
#25620=CARTESIAN_POINT('Ctrl Pts',(0.747103932787919,1.,2.06220058927826));
#25621=CARTESIAN_POINT('Ctrl Pts',(0.748091554183802,-1.,2.05713023031007));
#25622=CARTESIAN_POINT('Ctrl Pts',(0.748091554183802,1.,2.05713023031007));
#25623=CARTESIAN_POINT('Ctrl Pts',(0.749287468665046,-1.,2.05079645592154));
#25624=CARTESIAN_POINT('Ctrl Pts',(0.749287468665046,1.,2.05079645592154));
#25625=CARTESIAN_POINT('Ctrl Pts',(0.750444657875575,-1.,2.04446689147979));
#25626=CARTESIAN_POINT('Ctrl Pts',(0.750444657875575,1.,2.04446689147979));
#25627=CARTESIAN_POINT('Ctrl Pts',(0.751562963361115,-1.,2.03814160092099));
#25628=CARTESIAN_POINT('Ctrl Pts',(0.751562963361115,1.,2.03814160092099));
#25629=CARTESIAN_POINT('Ctrl Pts',(0.75264218048721,-1.,2.03182068456221));
#25630=CARTESIAN_POINT('Ctrl Pts',(0.75264218048721,1.,2.03182068456221));
#25631=CARTESIAN_POINT('Ctrl Pts',(0.753682061112768,-1.,2.02550428623313));
#25632=CARTESIAN_POINT('Ctrl Pts',(0.753682061112768,1.,2.02550428623313));
#25633=CARTESIAN_POINT('Ctrl Pts',(0.754682330722816,-1.,2.01919259405809));
#25634=CARTESIAN_POINT('Ctrl Pts',(0.754682330722816,1.,2.01919259405809));
#25635=CARTESIAN_POINT('Ctrl Pts',(0.755642704957865,-1.,2.01288584328084));
#25636=CARTESIAN_POINT('Ctrl Pts',(0.755642704957865,1.,2.01288584328084));
#25637=CARTESIAN_POINT('Ctrl Pts',(0.75656290464667,-1.,2.0065843158773));
#25638=CARTESIAN_POINT('Ctrl Pts',(0.75656290464667,1.,2.0065843158773));
#25639=CARTESIAN_POINT('Ctrl Pts',(0.757442676862724,-1.,2.00028834739178));
#25640=CARTESIAN_POINT('Ctrl Pts',(0.757442676862724,1.,2.00028834739178));
#25641=CARTESIAN_POINT('Ctrl Pts',(0.758281796766761,-1.,1.99399831098817));
#25642=CARTESIAN_POINT('Ctrl Pts',(0.758281796766761,1.,1.99399831098817));
#25643=CARTESIAN_POINT('Ctrl Pts',(0.759080037802488,-1.,1.98771456680874));
#25644=CARTESIAN_POINT('Ctrl Pts',(0.759080037802488,1.,1.98771456680874));
#25645=CARTESIAN_POINT('Ctrl Pts',(0.75983714745219,-1.,1.98143741418172));
#25646=CARTESIAN_POINT('Ctrl Pts',(0.75983714745219,1.,1.98143741418172));
#25647=CARTESIAN_POINT('Ctrl Pts',(0.760552825409757,-1.,1.97516705321494));
#25648=CARTESIAN_POINT('Ctrl Pts',(0.760552825409757,1.,1.97516705321494));
#25649=CARTESIAN_POINT('Ctrl Pts',(0.76122669048382,-1.,1.96890351582499));
#25650=CARTESIAN_POINT('Ctrl Pts',(0.76122669048382,1.,1.96890351582499));
#25651=CARTESIAN_POINT('Ctrl Pts',(0.761858300014423,-1.,1.96264672744186));
#25652=CARTESIAN_POINT('Ctrl Pts',(0.761858300014423,1.,1.96264672744186));
#25653=CARTESIAN_POINT('Ctrl Pts',(0.762447203806178,-1.,1.95639665309869));
#25654=CARTESIAN_POINT('Ctrl Pts',(0.762447203806178,1.,1.95639665309869));
#25655=CARTESIAN_POINT('Ctrl Pts',(0.762992990878769,-1.,1.95015342590024));
#25656=CARTESIAN_POINT('Ctrl Pts',(0.762992990878769,1.,1.95015342590024));
#25657=CARTESIAN_POINT('Ctrl Pts',(0.763495333538629,-1.,1.9439174661764));
#25658=CARTESIAN_POINT('Ctrl Pts',(0.763495333538629,1.,1.9439174661764));
#25659=CARTESIAN_POINT('Ctrl Pts',(0.763954049121458,-1.,1.93768964875886));
#25660=CARTESIAN_POINT('Ctrl Pts',(0.763954049121458,1.,1.93768964875886));
#25661=CARTESIAN_POINT('Ctrl Pts',(0.76436901067394,-1.,1.93147105496382));
#25662=CARTESIAN_POINT('Ctrl Pts',(0.76436901067394,1.,1.93147105496382));
#25663=CARTESIAN_POINT('Ctrl Pts',(0.764740025488211,-1.,1.92526263537048));
#25664=CARTESIAN_POINT('Ctrl Pts',(0.764740025488211,1.,1.92526263537048));
#25665=CARTESIAN_POINT('Ctrl Pts',(0.765066729667088,-1.,1.91906491634196));
#25666=CARTESIAN_POINT('Ctrl Pts',(0.765066729667088,1.,1.91906491634196));
#25667=CARTESIAN_POINT('Ctrl Pts',(0.765348465884722,-1.,1.91287765805169));
#25668=CARTESIAN_POINT('Ctrl Pts',(0.765348465884722,1.,1.91287765805169));
#25669=CARTESIAN_POINT('Ctrl Pts',(0.765584196937919,-1.,1.90669961402356));
#25670=CARTESIAN_POINT('Ctrl Pts',(0.765584196937919,1.,1.90669961402356));
#25671=CARTESIAN_POINT('Ctrl Pts',(0.765772772593386,-1.,1.90052930393596));
#25672=CARTESIAN_POINT('Ctrl Pts',(0.765772772593386,1.,1.90052930393596));
#25673=CARTESIAN_POINT('Ctrl Pts',(0.765913193856978,-1.,1.89436577771388));
#25674=CARTESIAN_POINT('Ctrl Pts',(0.765913193856978,1.,1.89436577771388));
#25675=CARTESIAN_POINT('Ctrl Pts',(0.766004837062091,-1.,1.88820926433409));
#25676=CARTESIAN_POINT('Ctrl Pts',(0.766004837062091,1.,1.88820926433409));
#25677=CARTESIAN_POINT('Ctrl Pts',(0.766047794851864,-1.,1.88206215302561));
#25678=CARTESIAN_POINT('Ctrl Pts',(0.766047794851864,1.,1.88206215302561));
#25679=CARTESIAN_POINT('Ctrl Pts',(0.766042837036744,-1.,1.87592888967883));
#25680=CARTESIAN_POINT('Ctrl Pts',(0.766042837036744,1.,1.87592888967883));
#25681=CARTESIAN_POINT('Ctrl Pts',(0.765990708546091,-1.,1.86981398314341));
#25682=CARTESIAN_POINT('Ctrl Pts',(0.765990708546091,1.,1.86981398314341));
#25683=CARTESIAN_POINT('Ctrl Pts',(0.765891519092547,-1.,1.86372027063312));
#25684=CARTESIAN_POINT('Ctrl Pts',(0.765891519092547,1.,1.86372027063312));
#25685=CARTESIAN_POINT('Ctrl Pts',(0.765744212909318,-1.,1.85764741390394));
#25686=CARTESIAN_POINT('Ctrl Pts',(0.765744212909318,1.,1.85764741390394));
#25687=CARTESIAN_POINT('Ctrl Pts',(0.765545710619062,-1.,1.85158945130063));
#25688=CARTESIAN_POINT('Ctrl Pts',(0.765545710619062,1.,1.85158945130063));
#25689=CARTESIAN_POINT('Ctrl Pts',(0.765291664862029,-1.,1.84553698875924));
#25690=CARTESIAN_POINT('Ctrl Pts',(0.765291664862029,1.,1.84553698875924));
#25691=CARTESIAN_POINT('Ctrl Pts',(0.764978057881737,-1.,1.83948181064835));
#25692=CARTESIAN_POINT('Ctrl Pts',(0.764978057881737,1.,1.83948181064835));
#25693=CARTESIAN_POINT('Ctrl Pts',(0.764602549687853,-1.,1.83342077227142));
#25694=CARTESIAN_POINT('Ctrl Pts',(0.764602549687853,1.,1.83342077227142));
#25695=CARTESIAN_POINT('Ctrl Pts',(0.764165902605995,-1.,1.82735991200065));
#25696=CARTESIAN_POINT('Ctrl Pts',(0.764165902605995,1.,1.82735991200065));
#25697=CARTESIAN_POINT('Ctrl Pts',(0.763673465462726,-1.,1.82131873145266));
#25698=CARTESIAN_POINT('Ctrl Pts',(0.763673465462726,1.,1.82131873145266));
#25699=CARTESIAN_POINT('Ctrl Pts',(0.763132003836634,-1.,1.8153211840553));
#25700=CARTESIAN_POINT('Ctrl Pts',(0.763132003836634,1.,1.8153211840553));
#25701=CARTESIAN_POINT('Ctrl Pts',(0.762546129463938,-1.,1.80938551463965));
#25702=CARTESIAN_POINT('Ctrl Pts',(0.762546129463938,1.,1.80938551463965));
#25703=CARTESIAN_POINT('Ctrl Pts',(0.761915336443547,-1.,1.80351583877342));
#25704=CARTESIAN_POINT('Ctrl Pts',(0.761915336443547,1.,1.80351583877342));
#25705=CARTESIAN_POINT('Ctrl Pts',(0.761229695230558,-1.,1.79768986997783));
#25706=CARTESIAN_POINT('Ctrl Pts',(0.761229695230558,1.,1.79768986997783));
#25707=CARTESIAN_POINT('Ctrl Pts',(0.760469555880749,-1.,1.7918581561088));
#25708=CARTESIAN_POINT('Ctrl Pts',(0.760469555880749,1.,1.7918581561088));
#25709=CARTESIAN_POINT('Ctrl Pts',(0.759614401110189,-1.,1.78596964884604));
#25710=CARTESIAN_POINT('Ctrl Pts',(0.759614401110189,1.,1.78596964884604));
#25711=CARTESIAN_POINT('Ctrl Pts',(0.758650626677518,-1.,1.77999411220945));
#25712=CARTESIAN_POINT('Ctrl Pts',(0.758650626677518,1.,1.77999411220945));
#25713=CARTESIAN_POINT('Ctrl Pts',(0.757578264077028,-1.,1.77394167108292));
#25714=CARTESIAN_POINT('Ctrl Pts',(0.757578264077028,1.,1.77394167108292));
#25715=CARTESIAN_POINT('Ctrl Pts',(0.75642189602781,-1.,1.76789396002998));
#25716=CARTESIAN_POINT('Ctrl Pts',(0.75642189602781,1.,1.76789396002998));
#25717=CARTESIAN_POINT('Ctrl Pts',(0.755220979974461,-1.,1.76197817240128));
#25718=CARTESIAN_POINT('Ctrl Pts',(0.755220979974461,1.,1.76197817240128));
#25719=CARTESIAN_POINT('Ctrl Pts',(0.754009254027828,-1.,1.75631083600019));
#25720=CARTESIAN_POINT('Ctrl Pts',(0.754009254027828,1.,1.75631083600019));
#25721=CARTESIAN_POINT('Ctrl Pts',(0.752797683531314,-1.,1.75095139468794));
#25722=CARTESIAN_POINT('Ctrl Pts',(0.752797683531314,1.,1.75095139468794));
#25723=CARTESIAN_POINT('Ctrl Pts',(0.751555614164482,-1.,1.74585086852502));
#25724=CARTESIAN_POINT('Ctrl Pts',(0.751555614164482,1.,1.74585086852502));
#25725=CARTESIAN_POINT('Ctrl Pts',(0.750193435981249,-1.,1.74080458267114));
#25726=CARTESIAN_POINT('Ctrl Pts',(0.750193435981249,1.,1.74080458267114));
#25727=CARTESIAN_POINT('Ctrl Pts',(0.74858246295687,-1.,1.7355035168033));
#25728=CARTESIAN_POINT('Ctrl Pts',(0.74858246295687,1.,1.7355035168033));
#25729=CARTESIAN_POINT('Ctrl Pts',(0.746574710097752,-1.,1.72958533647714));
#25730=CARTESIAN_POINT('Ctrl Pts',(0.746574710097752,1.,1.72958533647714));
#25731=CARTESIAN_POINT('Ctrl Pts',(0.744021445433093,-1.,1.72268229916769));
#25732=CARTESIAN_POINT('Ctrl Pts',(0.744021445433093,1.,1.72268229916769));
#25733=CARTESIAN_POINT('Ctrl Pts',(0.74079516202821,-1.,1.71447789751001));
#25734=CARTESIAN_POINT('Ctrl Pts',(0.74079516202821,1.,1.71447789751001));
#25735=CARTESIAN_POINT('Ctrl Pts',(0.736799665716932,-1.,1.70473309004249));
#25736=CARTESIAN_POINT('Ctrl Pts',(0.736799665716932,1.,1.70473309004249));
#25737=CARTESIAN_POINT('Ctrl Pts',(0.731963238685357,-1.,1.69326921972915));
#25738=CARTESIAN_POINT('Ctrl Pts',(0.731963238685357,1.,1.69326921972915));
#25739=CARTESIAN_POINT('Ctrl Pts',(0.726235967982445,-1.,1.67996158451922));
#25740=CARTESIAN_POINT('Ctrl Pts',(0.726235967982445,1.,1.67996158451922));
#25741=CARTESIAN_POINT('Ctrl Pts',(0.719585433787949,-1.,1.66472880551777));
#25742=CARTESIAN_POINT('Ctrl Pts',(0.719585433787949,1.,1.66472880551777));
#25743=CARTESIAN_POINT('Ctrl Pts',(0.711993139340447,-1.,1.64752408828442));
#25744=CARTESIAN_POINT('Ctrl Pts',(0.711993139340447,1.,1.64752408828442));
#25745=CARTESIAN_POINT('Ctrl Pts',(0.705159151977294,-1.,1.6321654166204));
#25746=CARTESIAN_POINT('Ctrl Pts',(0.705159151977294,1.,1.6321654166204));
#25747=CARTESIAN_POINT('Ctrl Pts',(0.699605146398836,-1.,1.61974673471117));
#25748=CARTESIAN_POINT('Ctrl Pts',(0.699605146398836,1.,1.61974673471117));
#25749=CARTESIAN_POINT('Ctrl Pts',(0.69571209787897,-1.,1.61106790957619));
#25750=CARTESIAN_POINT('Ctrl Pts',(0.69571209787897,1.,1.61106790957619));
#25751=CARTESIAN_POINT('Ctrl Pts',(0.693717979106305,-1.,1.60662857109684));
#25752=CARTESIAN_POINT('Ctrl Pts',(0.693717979106305,1.,1.60662857109684));
#25753=CARTESIAN_POINT('',(0.7455743247944,1.,2.0698113262342));
#25754=CARTESIAN_POINT('Ctrl Pts',(0.7455743247944,1.,2.0698113262342));
#25755=CARTESIAN_POINT('Ctrl Pts',(0.745832791378367,1.,2.06854248895728));
#25756=CARTESIAN_POINT('Ctrl Pts',(0.7463458715442,1.,2.06600523016815));
#25757=CARTESIAN_POINT('Ctrl Pts',(0.747103932787919,1.,2.06220058927826));
#25758=CARTESIAN_POINT('Ctrl Pts',(0.748091554183802,1.,2.05713023031007));
#25759=CARTESIAN_POINT('Ctrl Pts',(0.749287468665046,1.,2.05079645592154));
#25760=CARTESIAN_POINT('Ctrl Pts',(0.750444657875575,1.,2.04446689147979));
#25761=CARTESIAN_POINT('Ctrl Pts',(0.751562963361115,1.,2.03814160092099));
#25762=CARTESIAN_POINT('Ctrl Pts',(0.75264218048721,1.,2.03182068456221));
#25763=CARTESIAN_POINT('Ctrl Pts',(0.753682061112768,1.,2.02550428623313));
#25764=CARTESIAN_POINT('Ctrl Pts',(0.754682330722816,1.,2.01919259405809));
#25765=CARTESIAN_POINT('Ctrl Pts',(0.755642704957865,1.,2.01288584328084));
#25766=CARTESIAN_POINT('Ctrl Pts',(0.75656290464667,1.,2.0065843158773));
#25767=CARTESIAN_POINT('Ctrl Pts',(0.757442676862724,1.,2.00028834739178));
#25768=CARTESIAN_POINT('Ctrl Pts',(0.758281796766761,1.,1.99399831098817));
#25769=CARTESIAN_POINT('Ctrl Pts',(0.759080037802488,1.,1.98771456680874));
#25770=CARTESIAN_POINT('Ctrl Pts',(0.75983714745219,1.,1.98143741418172));
#25771=CARTESIAN_POINT('Ctrl Pts',(0.760552825409757,1.,1.97516705321494));
#25772=CARTESIAN_POINT('Ctrl Pts',(0.76122669048382,1.,1.96890351582499));
#25773=CARTESIAN_POINT('Ctrl Pts',(0.761858300014423,1.,1.96264672744186));
#25774=CARTESIAN_POINT('Ctrl Pts',(0.762447203806178,1.,1.95639665309869));
#25775=CARTESIAN_POINT('Ctrl Pts',(0.762992990878769,1.,1.95015342590024));
#25776=CARTESIAN_POINT('Ctrl Pts',(0.763495333538629,1.,1.9439174661764));
#25777=CARTESIAN_POINT('Ctrl Pts',(0.763954049121458,1.,1.93768964875886));
#25778=CARTESIAN_POINT('Ctrl Pts',(0.76436901067394,1.,1.93147105496382));
#25779=CARTESIAN_POINT('Ctrl Pts',(0.764740025488211,1.,1.92526263537048));
#25780=CARTESIAN_POINT('Ctrl Pts',(0.765066729667088,1.,1.91906491634196));
#25781=CARTESIAN_POINT('Ctrl Pts',(0.765348465884722,1.,1.91287765805169));
#25782=CARTESIAN_POINT('Ctrl Pts',(0.765584196937919,1.,1.90669961402356));
#25783=CARTESIAN_POINT('Ctrl Pts',(0.765772772593386,1.,1.90052930393596));
#25784=CARTESIAN_POINT('Ctrl Pts',(0.765913193856978,1.,1.89436577771388));
#25785=CARTESIAN_POINT('Ctrl Pts',(0.766004837062091,1.,1.88820926433409));
#25786=CARTESIAN_POINT('Ctrl Pts',(0.766047794851864,1.,1.88206215302561));
#25787=CARTESIAN_POINT('Ctrl Pts',(0.766042837036744,1.,1.87592888967883));
#25788=CARTESIAN_POINT('Ctrl Pts',(0.765990708546091,1.,1.86981398314341));
#25789=CARTESIAN_POINT('Ctrl Pts',(0.765891519092547,1.,1.86372027063312));
#25790=CARTESIAN_POINT('Ctrl Pts',(0.765744212909318,1.,1.85764741390394));
#25791=CARTESIAN_POINT('Ctrl Pts',(0.765545710619062,1.,1.85158945130063));
#25792=CARTESIAN_POINT('Ctrl Pts',(0.765291664862029,1.,1.84553698875924));
#25793=CARTESIAN_POINT('Ctrl Pts',(0.764978057881737,1.,1.83948181064835));
#25794=CARTESIAN_POINT('Ctrl Pts',(0.764602549687853,1.,1.83342077227142));
#25795=CARTESIAN_POINT('Ctrl Pts',(0.764165902605995,1.,1.82735991200065));
#25796=CARTESIAN_POINT('Ctrl Pts',(0.763673465462726,1.,1.82131873145266));
#25797=CARTESIAN_POINT('Ctrl Pts',(0.763132003836634,1.,1.8153211840553));
#25798=CARTESIAN_POINT('Ctrl Pts',(0.762546129463938,1.,1.80938551463965));
#25799=CARTESIAN_POINT('Ctrl Pts',(0.761915336443547,1.,1.80351583877342));
#25800=CARTESIAN_POINT('Ctrl Pts',(0.761229695230558,1.,1.79768986997783));
#25801=CARTESIAN_POINT('Ctrl Pts',(0.760469555880749,1.,1.7918581561088));
#25802=CARTESIAN_POINT('Ctrl Pts',(0.759614401110189,1.,1.78596964884604));
#25803=CARTESIAN_POINT('Ctrl Pts',(0.758650626677518,1.,1.77999411220945));
#25804=CARTESIAN_POINT('Ctrl Pts',(0.757578264077028,1.,1.77394167108292));
#25805=CARTESIAN_POINT('Ctrl Pts',(0.75642189602781,1.,1.76789396002998));
#25806=CARTESIAN_POINT('Ctrl Pts',(0.755220979974461,1.,1.76197817240128));
#25807=CARTESIAN_POINT('Ctrl Pts',(0.754009254027828,1.,1.75631083600019));
#25808=CARTESIAN_POINT('Ctrl Pts',(0.752797683531314,1.,1.75095139468794));
#25809=CARTESIAN_POINT('Ctrl Pts',(0.751555614164482,1.,1.74585086852502));
#25810=CARTESIAN_POINT('Ctrl Pts',(0.750193435981249,1.,1.74080458267114));
#25811=CARTESIAN_POINT('Ctrl Pts',(0.74858246295687,1.,1.7355035168033));
#25812=CARTESIAN_POINT('Ctrl Pts',(0.746574710097752,1.,1.72958533647714));
#25813=CARTESIAN_POINT('Ctrl Pts',(0.744021445433093,1.,1.72268229916769));
#25814=CARTESIAN_POINT('Ctrl Pts',(0.74079516202821,1.,1.71447789751001));
#25815=CARTESIAN_POINT('Ctrl Pts',(0.736799665716932,1.,1.70473309004249));
#25816=CARTESIAN_POINT('Ctrl Pts',(0.731963238685357,1.,1.69326921972915));
#25817=CARTESIAN_POINT('Ctrl Pts',(0.726235967982445,1.,1.67996158451922));
#25818=CARTESIAN_POINT('Ctrl Pts',(0.719585433787949,1.,1.66472880551777));
#25819=CARTESIAN_POINT('Ctrl Pts',(0.711993139340447,1.,1.64752408828442));
#25820=CARTESIAN_POINT('Ctrl Pts',(0.705159151977294,1.,1.6321654166204));
#25821=CARTESIAN_POINT('Ctrl Pts',(0.699605146398836,1.,1.61974673471117));
#25822=CARTESIAN_POINT('Ctrl Pts',(0.69571209787897,1.,1.61106790957619));
#25823=CARTESIAN_POINT('Ctrl Pts',(0.693717979106305,1.,1.60662857109684));
#25824=CARTESIAN_POINT('',(0.7455743247944,0.,2.0698113262342));
#25825=CARTESIAN_POINT('Origin',(0.61342227326009,0.,2.11275013067528));
#25826=CARTESIAN_POINT('',(0.61342227326009,1.,2.11275013067528));
#25827=CARTESIAN_POINT('',(0.7455743247944,1.,2.0698113262342));
#25828=CARTESIAN_POINT('',(0.61342227326009,0.,2.11275013067528));
#25829=CARTESIAN_POINT('Ctrl Pts',(0.383122945602004,-1.,1.7075470150345));
#25830=CARTESIAN_POINT('Ctrl Pts',(0.383122945602004,1.,1.7075470150345));
#25831=CARTESIAN_POINT('Ctrl Pts',(0.384119047315541,-1.,1.71231062891958));
#25832=CARTESIAN_POINT('Ctrl Pts',(0.384119047315541,1.,1.71231062891958));
#25833=CARTESIAN_POINT('Ctrl Pts',(0.38607079032701,-1.,1.72162022246158));
#25834=CARTESIAN_POINT('Ctrl Pts',(0.38607079032701,1.,1.72162022246158));
#25835=CARTESIAN_POINT('Ctrl Pts',(0.388877023509191,-1.,1.7349317097561));
#25836=CARTESIAN_POINT('Ctrl Pts',(0.388877023509191,1.,1.7349317097561));
#25837=CARTESIAN_POINT('Ctrl Pts',(0.392375812294307,-1.,1.75137405313962));
#25838=CARTESIAN_POINT('Ctrl Pts',(0.392375812294307,1.,1.75137405313962));
#25839=CARTESIAN_POINT('Ctrl Pts',(0.39634619612042,-1.,1.7697556004756));
#25840=CARTESIAN_POINT('Ctrl Pts',(0.39634619612042,1.,1.7697556004756));
#25841=CARTESIAN_POINT('Ctrl Pts',(0.39991940378308,-1.,1.78598826347533));
#25842=CARTESIAN_POINT('Ctrl Pts',(0.39991940378308,1.,1.78598826347533));
#25843=CARTESIAN_POINT('Ctrl Pts',(0.403107976170441,-1.,1.80012077176221));
#25844=CARTESIAN_POINT('Ctrl Pts',(0.403107976170441,1.,1.80012077176221));
#25845=CARTESIAN_POINT('Ctrl Pts',(0.405933518411838,-1.,1.81223801813988));
#25846=CARTESIAN_POINT('Ctrl Pts',(0.405933518411838,1.,1.81223801813988));
#25847=CARTESIAN_POINT('Ctrl Pts',(0.408428948108533,-1.,1.8224702267854));
#25848=CARTESIAN_POINT('Ctrl Pts',(0.408428948108533,1.,1.8224702267854));
#25849=CARTESIAN_POINT('Ctrl Pts',(0.410641256301674,-1.,1.83100408895216));
#25850=CARTESIAN_POINT('Ctrl Pts',(0.410641256301674,1.,1.83100408895216));
#25851=CARTESIAN_POINT('Ctrl Pts',(0.412633125322161,-1.,1.83808953475839));
#25852=CARTESIAN_POINT('Ctrl Pts',(0.412633125322161,1.,1.83808953475839));
#25853=CARTESIAN_POINT('Ctrl Pts',(0.41448743825434,-1.,1.8440575707371));
#25854=CARTESIAN_POINT('Ctrl Pts',(0.41448743825434,1.,1.8440575707371));
#25855=CARTESIAN_POINT('Ctrl Pts',(0.416300022038864,-1.,1.84929312929882));
#25856=CARTESIAN_POINT('Ctrl Pts',(0.416300022038864,1.,1.84929312929882));
#25857=CARTESIAN_POINT('Ctrl Pts',(0.418164129143534,-1.,1.85417632856234));
#25858=CARTESIAN_POINT('Ctrl Pts',(0.418164129143534,1.,1.85417632856234));
#25859=CARTESIAN_POINT('Ctrl Pts',(0.420157287975619,-1.,1.85903281096686));
#25860=CARTESIAN_POINT('Ctrl Pts',(0.420157287975619,1.,1.85903281096686));
#25861=CARTESIAN_POINT('Ctrl Pts',(0.422327307418275,-1.,1.86408083334028));
#25862=CARTESIAN_POINT('Ctrl Pts',(0.422327307418275,1.,1.86408083334028));
#25863=CARTESIAN_POINT('Ctrl Pts',(0.424678177291358,-1.,1.86937803944323));
#25864=CARTESIAN_POINT('Ctrl Pts',(0.424678177291358,1.,1.86937803944323));
#25865=CARTESIAN_POINT('Ctrl Pts',(0.427183828519102,-1.,1.87486989291484));
#25866=CARTESIAN_POINT('Ctrl Pts',(0.427183828519102,1.,1.87486989291484));
#25867=CARTESIAN_POINT('Ctrl Pts',(0.429803062482344,-1.,1.88044229001832));
#25868=CARTESIAN_POINT('Ctrl Pts',(0.429803062482344,1.,1.88044229001832));
#25869=CARTESIAN_POINT('Ctrl Pts',(0.432493038548748,-1.,1.88596913666793));
#25870=CARTESIAN_POINT('Ctrl Pts',(0.432493038548748,1.,1.88596913666793));
#25871=CARTESIAN_POINT('Ctrl Pts',(0.435225660963383,-1.,1.89136993975504));
#25872=CARTESIAN_POINT('Ctrl Pts',(0.435225660963383,1.,1.89136993975504));
#25873=CARTESIAN_POINT('Ctrl Pts',(0.437995003948244,-1.,1.89663648956466));
#25874=CARTESIAN_POINT('Ctrl Pts',(0.437995003948244,1.,1.89663648956466));
#25875=CARTESIAN_POINT('Ctrl Pts',(0.440807833704038,-1.,1.90180124389086));
#25876=CARTESIAN_POINT('Ctrl Pts',(0.440807833704038,1.,1.90180124389086));
#25877=CARTESIAN_POINT('Ctrl Pts',(0.44367755684915,-1.,1.90691756144898));
#25878=CARTESIAN_POINT('Ctrl Pts',(0.44367755684915,1.,1.90691756144898));
#25879=CARTESIAN_POINT('Ctrl Pts',(0.446617343485711,-1.,1.9120369998112));
#25880=CARTESIAN_POINT('Ctrl Pts',(0.446617343485711,1.,1.9120369998112));
#25881=CARTESIAN_POINT('Ctrl Pts',(0.449632260106662,-1.,1.91718342555755));
#25882=CARTESIAN_POINT('Ctrl Pts',(0.449632260106662,1.,1.91718342555755));
#25883=CARTESIAN_POINT('Ctrl Pts',(0.452719478359432,-1.,1.92235380648502));
#25884=CARTESIAN_POINT('Ctrl Pts',(0.452719478359432,1.,1.92235380648502));
#25885=CARTESIAN_POINT('Ctrl Pts',(0.45587200517437,-1.,1.92753067150476));
#25886=CARTESIAN_POINT('Ctrl Pts',(0.45587200517437,1.,1.92753067150476));
#25887=CARTESIAN_POINT('Ctrl Pts',(0.459081234547926,-1.,1.93269066517934));
#25888=CARTESIAN_POINT('Ctrl Pts',(0.459081234547926,1.,1.93269066517934));
#25889=CARTESIAN_POINT('Ctrl Pts',(0.462340031009056,-1.,1.93781486640821));
#25890=CARTESIAN_POINT('Ctrl Pts',(0.462340031009056,1.,1.93781486640821));
#25891=CARTESIAN_POINT('Ctrl Pts',(0.46564546202603,-1.,1.9428979419619));
#25892=CARTESIAN_POINT('Ctrl Pts',(0.46564546202603,1.,1.9428979419619));
#25893=CARTESIAN_POINT('Ctrl Pts',(0.468997482913135,-1.,1.94794381136514));
#25894=CARTESIAN_POINT('Ctrl Pts',(0.468997482913135,1.,1.94794381136514));
#25895=CARTESIAN_POINT('Ctrl Pts',(0.472397672264072,-1.,1.95296148278133));
#25896=CARTESIAN_POINT('Ctrl Pts',(0.472397672264072,1.,1.95296148278133));
#25897=CARTESIAN_POINT('Ctrl Pts',(0.475848034683176,-1.,1.95796111148177));
#25898=CARTESIAN_POINT('Ctrl Pts',(0.475848034683176,1.,1.95796111148177));
#25899=CARTESIAN_POINT('Ctrl Pts',(0.479349583074855,-1.,1.96294933055943));
#25900=CARTESIAN_POINT('Ctrl Pts',(0.479349583074855,1.,1.96294933055943));
#25901=CARTESIAN_POINT('Ctrl Pts',(0.48290166212069,-1.,1.96792703422362));
#25902=CARTESIAN_POINT('Ctrl Pts',(0.48290166212069,1.,1.96792703422362));
#25903=CARTESIAN_POINT('Ctrl Pts',(0.486502692907658,-1.,1.97289186263272));
#25904=CARTESIAN_POINT('Ctrl Pts',(0.486502692907658,1.,1.97289186263272));
#25905=CARTESIAN_POINT('Ctrl Pts',(0.490150627860952,-1.,1.97783973019229));
#25906=CARTESIAN_POINT('Ctrl Pts',(0.490150627860952,1.,1.97783973019229));
#25907=CARTESIAN_POINT('Ctrl Pts',(0.493843476541494,-1.,1.98276658761821));
#25908=CARTESIAN_POINT('Ctrl Pts',(0.493843476541494,1.,1.98276658761821));
#25909=CARTESIAN_POINT('Ctrl Pts',(0.497579909545574,-1.,1.98767044752932));
#25910=CARTESIAN_POINT('Ctrl Pts',(0.497579909545574,1.,1.98767044752932));
#25911=CARTESIAN_POINT('Ctrl Pts',(0.501359287727146,-1.,1.99255149126155));
#25912=CARTESIAN_POINT('Ctrl Pts',(0.501359287727146,1.,1.99255149126155));
#25913=CARTESIAN_POINT('Ctrl Pts',(0.505181361323026,-1.,1.99741107463572));
#25914=CARTESIAN_POINT('Ctrl Pts',(0.505181361323026,1.,1.99741107463572));
#25915=CARTESIAN_POINT('Ctrl Pts',(0.509046069886157,-1.,2.00225107134734));
#25916=CARTESIAN_POINT('Ctrl Pts',(0.509046069886157,1.,2.00225107134734));
#25917=CARTESIAN_POINT('Ctrl Pts',(0.512953306961792,-1.,2.00707309946949));
#25918=CARTESIAN_POINT('Ctrl Pts',(0.512953306961792,1.,2.00707309946949));
#25919=CARTESIAN_POINT('Ctrl Pts',(0.516902681728687,-1.,2.01187773939242));
#25920=CARTESIAN_POINT('Ctrl Pts',(0.516902681728687,1.,2.01187773939242));
#25921=CARTESIAN_POINT('Ctrl Pts',(0.52089359039937,-1.,2.01666477917286));
#25922=CARTESIAN_POINT('Ctrl Pts',(0.52089359039937,1.,2.01666477917286));
#25923=CARTESIAN_POINT('Ctrl Pts',(0.524925318333476,-1.,2.02143356304698));
#25924=CARTESIAN_POINT('Ctrl Pts',(0.524925318333476,1.,2.02143356304698));
#25925=CARTESIAN_POINT('Ctrl Pts',(0.528997127241914,-1.,2.0261832908329));
#25926=CARTESIAN_POINT('Ctrl Pts',(0.528997127241914,1.,2.0261832908329));
#25927=CARTESIAN_POINT('Ctrl Pts',(0.533108355132976,-1.,2.03091336214426));
#25928=CARTESIAN_POINT('Ctrl Pts',(0.533108355132976,1.,2.03091336214426));
#25929=CARTESIAN_POINT('Ctrl Pts',(0.537258489833262,-1.,2.03562362954037));
#25930=CARTESIAN_POINT('Ctrl Pts',(0.537258489833262,1.,2.03562362954037));
#25931=CARTESIAN_POINT('Ctrl Pts',(0.541447120615659,-1.,2.04031422690527));
#25932=CARTESIAN_POINT('Ctrl Pts',(0.541447120615659,1.,2.04031422690527));
#25933=CARTESIAN_POINT('Ctrl Pts',(0.54567390381743,-1.,2.04498544714588));
#25934=CARTESIAN_POINT('Ctrl Pts',(0.54567390381743,1.,2.04498544714588));
#25935=CARTESIAN_POINT('Ctrl Pts',(0.549938525150295,-1.,2.04963761077958));
#25936=CARTESIAN_POINT('Ctrl Pts',(0.549938525150295,1.,2.04963761077958));
#25937=CARTESIAN_POINT('Ctrl Pts',(0.554240657463906,-1.,2.05427091604413));
#25938=CARTESIAN_POINT('Ctrl Pts',(0.554240657463906,1.,2.05427091604413));
#25939=CARTESIAN_POINT('Ctrl Pts',(0.558579940185151,-1.,2.05888537756462));
#25940=CARTESIAN_POINT('Ctrl Pts',(0.558579940185151,1.,2.05888537756462));
#25941=CARTESIAN_POINT('Ctrl Pts',(0.562955993082261,-1.,2.06348090160589));
#25942=CARTESIAN_POINT('Ctrl Pts',(0.562955993082261,1.,2.06348090160589));
#25943=CARTESIAN_POINT('Ctrl Pts',(0.567368421181087,-1.,2.06805732997334));
#25944=CARTESIAN_POINT('Ctrl Pts',(0.567368421181087,1.,2.06805732997334));
#25945=CARTESIAN_POINT('Ctrl Pts',(0.571816823242602,-1.,2.07261449292824));
#25946=CARTESIAN_POINT('Ctrl Pts',(0.571816823242602,1.,2.07261449292824));
#25947=CARTESIAN_POINT('Ctrl Pts',(0.576300797416844,-1.,2.07715226767559));
#25948=CARTESIAN_POINT('Ctrl Pts',(0.576300797416844,1.,2.07715226767559));
#25949=CARTESIAN_POINT('Ctrl Pts',(0.580819952108063,-1.,2.08167059018418));
#25950=CARTESIAN_POINT('Ctrl Pts',(0.580819952108063,1.,2.08167059018418));
#25951=CARTESIAN_POINT('Ctrl Pts',(0.585373918991617,-1.,2.08616943727951));
#25952=CARTESIAN_POINT('Ctrl Pts',(0.585373918991617,1.,2.08616943727951));
#25953=CARTESIAN_POINT('Ctrl Pts',(0.589962365403406,-1.,2.09064881812129));
#25954=CARTESIAN_POINT('Ctrl Pts',(0.589962365403406,1.,2.09064881812129));
#25955=CARTESIAN_POINT('Ctrl Pts',(0.594585006052162,-1.,2.0951087622027));
#25956=CARTESIAN_POINT('Ctrl Pts',(0.594585006052162,1.,2.0951087622027));
#25957=CARTESIAN_POINT('Ctrl Pts',(0.599241616420533,-1.,2.0995493086477));
#25958=CARTESIAN_POINT('Ctrl Pts',(0.599241616420533,1.,2.0995493086477));
#25959=CARTESIAN_POINT('Ctrl Pts',(0.60393203073603,-1.,2.10397049886949));
#25960=CARTESIAN_POINT('Ctrl Pts',(0.60393203073603,1.,2.10397049886949));
#25961=CARTESIAN_POINT('Ctrl Pts',(0.607711315454876,-1.,2.1074919961518));
#25962=CARTESIAN_POINT('Ctrl Pts',(0.607711315454876,1.,2.1074919961518));
#25963=CARTESIAN_POINT('Ctrl Pts',(0.610560911689898,-1.,2.11012443807238));
#25964=CARTESIAN_POINT('Ctrl Pts',(0.610560911689898,1.,2.11012443807238));
#25965=CARTESIAN_POINT('Ctrl Pts',(0.6124673655618,-1.,2.11187554259986));
#25966=CARTESIAN_POINT('Ctrl Pts',(0.6124673655618,1.,2.11187554259986));
#25967=CARTESIAN_POINT('Ctrl Pts',(0.61342227326009,-1.,2.11275013067528));
#25968=CARTESIAN_POINT('Ctrl Pts',(0.61342227326009,1.,2.11275013067528));
#25969=CARTESIAN_POINT('',(0.383122945602004,1.,1.7075470150345));
#25970=CARTESIAN_POINT('Ctrl Pts',(0.383122945602004,1.,1.7075470150345));
#25971=CARTESIAN_POINT('Ctrl Pts',(0.384119047315541,1.,1.71231062891958));
#25972=CARTESIAN_POINT('Ctrl Pts',(0.38607079032701,1.,1.72162022246158));
#25973=CARTESIAN_POINT('Ctrl Pts',(0.388877023509191,1.,1.7349317097561));
#25974=CARTESIAN_POINT('Ctrl Pts',(0.392375812294307,1.,1.75137405313962));
#25975=CARTESIAN_POINT('Ctrl Pts',(0.39634619612042,1.,1.7697556004756));
#25976=CARTESIAN_POINT('Ctrl Pts',(0.39991940378308,1.,1.78598826347533));
#25977=CARTESIAN_POINT('Ctrl Pts',(0.403107976170441,1.,1.80012077176221));
#25978=CARTESIAN_POINT('Ctrl Pts',(0.405933518411838,1.,1.81223801813988));
#25979=CARTESIAN_POINT('Ctrl Pts',(0.408428948108533,1.,1.8224702267854));
#25980=CARTESIAN_POINT('Ctrl Pts',(0.410641256301674,1.,1.83100408895216));
#25981=CARTESIAN_POINT('Ctrl Pts',(0.412633125322161,1.,1.83808953475839));
#25982=CARTESIAN_POINT('Ctrl Pts',(0.41448743825434,1.,1.8440575707371));
#25983=CARTESIAN_POINT('Ctrl Pts',(0.416300022038864,1.,1.84929312929882));
#25984=CARTESIAN_POINT('Ctrl Pts',(0.418164129143534,1.,1.85417632856234));
#25985=CARTESIAN_POINT('Ctrl Pts',(0.420157287975619,1.,1.85903281096686));
#25986=CARTESIAN_POINT('Ctrl Pts',(0.422327307418275,1.,1.86408083334028));
#25987=CARTESIAN_POINT('Ctrl Pts',(0.424678177291358,1.,1.86937803944323));
#25988=CARTESIAN_POINT('Ctrl Pts',(0.427183828519102,1.,1.87486989291484));
#25989=CARTESIAN_POINT('Ctrl Pts',(0.429803062482344,1.,1.88044229001832));
#25990=CARTESIAN_POINT('Ctrl Pts',(0.432493038548748,1.,1.88596913666793));
#25991=CARTESIAN_POINT('Ctrl Pts',(0.435225660963383,1.,1.89136993975504));
#25992=CARTESIAN_POINT('Ctrl Pts',(0.437995003948244,1.,1.89663648956466));
#25993=CARTESIAN_POINT('Ctrl Pts',(0.440807833704038,1.,1.90180124389086));
#25994=CARTESIAN_POINT('Ctrl Pts',(0.44367755684915,1.,1.90691756144898));
#25995=CARTESIAN_POINT('Ctrl Pts',(0.446617343485711,1.,1.9120369998112));
#25996=CARTESIAN_POINT('Ctrl Pts',(0.449632260106662,1.,1.91718342555755));
#25997=CARTESIAN_POINT('Ctrl Pts',(0.452719478359432,1.,1.92235380648502));
#25998=CARTESIAN_POINT('Ctrl Pts',(0.45587200517437,1.,1.92753067150476));
#25999=CARTESIAN_POINT('Ctrl Pts',(0.459081234547926,1.,1.93269066517934));
#26000=CARTESIAN_POINT('Ctrl Pts',(0.462340031009056,1.,1.93781486640821));
#26001=CARTESIAN_POINT('Ctrl Pts',(0.46564546202603,1.,1.9428979419619));
#26002=CARTESIAN_POINT('Ctrl Pts',(0.468997482913135,1.,1.94794381136514));
#26003=CARTESIAN_POINT('Ctrl Pts',(0.472397672264072,1.,1.95296148278133));
#26004=CARTESIAN_POINT('Ctrl Pts',(0.475848034683176,1.,1.95796111148177));
#26005=CARTESIAN_POINT('Ctrl Pts',(0.479349583074855,1.,1.96294933055943));
#26006=CARTESIAN_POINT('Ctrl Pts',(0.48290166212069,1.,1.96792703422362));
#26007=CARTESIAN_POINT('Ctrl Pts',(0.486502692907658,1.,1.97289186263272));
#26008=CARTESIAN_POINT('Ctrl Pts',(0.490150627860952,1.,1.97783973019229));
#26009=CARTESIAN_POINT('Ctrl Pts',(0.493843476541494,1.,1.98276658761821));
#26010=CARTESIAN_POINT('Ctrl Pts',(0.497579909545574,1.,1.98767044752932));
#26011=CARTESIAN_POINT('Ctrl Pts',(0.501359287727146,1.,1.99255149126155));
#26012=CARTESIAN_POINT('Ctrl Pts',(0.505181361323026,1.,1.99741107463572));
#26013=CARTESIAN_POINT('Ctrl Pts',(0.509046069886157,1.,2.00225107134734));
#26014=CARTESIAN_POINT('Ctrl Pts',(0.512953306961792,1.,2.00707309946949));
#26015=CARTESIAN_POINT('Ctrl Pts',(0.516902681728687,1.,2.01187773939242));
#26016=CARTESIAN_POINT('Ctrl Pts',(0.52089359039937,1.,2.01666477917286));
#26017=CARTESIAN_POINT('Ctrl Pts',(0.524925318333476,1.,2.02143356304698));
#26018=CARTESIAN_POINT('Ctrl Pts',(0.528997127241914,1.,2.0261832908329));
#26019=CARTESIAN_POINT('Ctrl Pts',(0.533108355132976,1.,2.03091336214426));
#26020=CARTESIAN_POINT('Ctrl Pts',(0.537258489833262,1.,2.03562362954037));
#26021=CARTESIAN_POINT('Ctrl Pts',(0.541447120615659,1.,2.04031422690527));
#26022=CARTESIAN_POINT('Ctrl Pts',(0.54567390381743,1.,2.04498544714588));
#26023=CARTESIAN_POINT('Ctrl Pts',(0.549938525150295,1.,2.04963761077958));
#26024=CARTESIAN_POINT('Ctrl Pts',(0.554240657463906,1.,2.05427091604413));
#26025=CARTESIAN_POINT('Ctrl Pts',(0.558579940185151,1.,2.05888537756462));
#26026=CARTESIAN_POINT('Ctrl Pts',(0.562955993082261,1.,2.06348090160589));
#26027=CARTESIAN_POINT('Ctrl Pts',(0.567368421181087,1.,2.06805732997334));
#26028=CARTESIAN_POINT('Ctrl Pts',(0.571816823242602,1.,2.07261449292824));
#26029=CARTESIAN_POINT('Ctrl Pts',(0.576300797416844,1.,2.07715226767559));
#26030=CARTESIAN_POINT('Ctrl Pts',(0.580819952108063,1.,2.08167059018418));
#26031=CARTESIAN_POINT('Ctrl Pts',(0.585373918991617,1.,2.08616943727951));
#26032=CARTESIAN_POINT('Ctrl Pts',(0.589962365403406,1.,2.09064881812129));
#26033=CARTESIAN_POINT('Ctrl Pts',(0.594585006052162,1.,2.0951087622027));
#26034=CARTESIAN_POINT('Ctrl Pts',(0.599241616420533,1.,2.0995493086477));
#26035=CARTESIAN_POINT('Ctrl Pts',(0.60393203073603,1.,2.10397049886949));
#26036=CARTESIAN_POINT('Ctrl Pts',(0.607711315454876,1.,2.1074919961518));
#26037=CARTESIAN_POINT('Ctrl Pts',(0.610560911689898,1.,2.11012443807238));
#26038=CARTESIAN_POINT('Ctrl Pts',(0.6124673655618,1.,2.11187554259986));
#26039=CARTESIAN_POINT('Ctrl Pts',(0.61342227326009,1.,2.11275013067528));
#26040=CARTESIAN_POINT('',(0.383122945602003,0.,1.7075470150345));
#26041=CARTESIAN_POINT('Origin',(0.,0.,0.));
#26042=CARTESIAN_POINT('',(0.163289472382896,1.,1.74236521665491));
#26043=CARTESIAN_POINT('Origin',(0.,1.,0.));
#26044=CARTESIAN_POINT('',(0.163289472382896,0.,1.74236521665491));
#26045=CARTESIAN_POINT('Ctrl Pts',(0.0694764450219578,-1.,2.19890268624765));
#26046=CARTESIAN_POINT('Ctrl Pts',(0.0694764450219578,1.,2.19890268624765));
#26047=CARTESIAN_POINT('Ctrl Pts',(0.0701143536325487,-1.,2.19777582085423));
#26048=CARTESIAN_POINT('Ctrl Pts',(0.0701143536325487,1.,2.19777582085423));
#26049=CARTESIAN_POINT('Ctrl Pts',(0.0713863779526151,-1.,2.19552129484002));
#26050=CARTESIAN_POINT('Ctrl Pts',(0.0713863779526151,1.,2.19552129484002));
#26051=CARTESIAN_POINT('Ctrl Pts',(0.0732830357306722,-1.,2.19213712013662));
#26052=CARTESIAN_POINT('Ctrl Pts',(0.0732830357306722,1.,2.19213712013662));
#26053=CARTESIAN_POINT('Ctrl Pts',(0.0757891465836145,-1.,2.1876201139953));
#26054=CARTESIAN_POINT('Ctrl Pts',(0.0757891465836145,1.,2.1876201139953));
#26055=CARTESIAN_POINT('Ctrl Pts',(0.078883772768524,-1.,2.18196589448887));
#26056=CARTESIAN_POINT('Ctrl Pts',(0.078883772768524,1.,2.18196589448887));
#26057=CARTESIAN_POINT('Ctrl Pts',(0.0819402680872763,-1.,2.176303712113));
#26058=CARTESIAN_POINT('Ctrl Pts',(0.0819402680872763,1.,2.176303712113));
#26059=CARTESIAN_POINT('Ctrl Pts',(0.084958462083537,-1.,2.17063357870952));
#26060=CARTESIAN_POINT('Ctrl Pts',(0.084958462083537,1.,2.17063357870952));
#26061=CARTESIAN_POINT('Ctrl Pts',(0.087938129138692,-1.,2.16495552645014));
#26062=CARTESIAN_POINT('Ctrl Pts',(0.087938129138692,1.,2.16495552645014));
#26063=CARTESIAN_POINT('Ctrl Pts',(0.0908789888107263,-1.,2.15926961544516));
#26064=CARTESIAN_POINT('Ctrl Pts',(0.0908789888107263,1.,2.15926961544516));
#26065=CARTESIAN_POINT('Ctrl Pts',(0.0937807218867641,-1.,2.1535759397817));
#26066=CARTESIAN_POINT('Ctrl Pts',(0.0937807218867641,1.,2.1535759397817));
#26067=CARTESIAN_POINT('Ctrl Pts',(0.0966429852305456,-1.,2.14787463531795));
#26068=CARTESIAN_POINT('Ctrl Pts',(0.0966429852305456,1.,2.14787463531795));
#26069=CARTESIAN_POINT('Ctrl Pts',(0.0994654261990913,-1.,2.14216588396025));
#26070=CARTESIAN_POINT('Ctrl Pts',(0.0994654261990913,1.,2.14216588396025));
#26071=CARTESIAN_POINT('Ctrl Pts',(0.1022477005561,-1.,2.13644992667165));
#26072=CARTESIAN_POINT('Ctrl Pts',(0.1022477005561,1.,2.13644992667165));
#26073=CARTESIAN_POINT('Ctrl Pts',(0.104989479152739,-1.,2.13072704887293));
#26074=CARTESIAN_POINT('Ctrl Pts',(0.104989479152739,1.,2.13072704887293));
#26075=CARTESIAN_POINT('Ctrl Pts',(0.10769043523109,-1.,2.12499752307));
#26076=CARTESIAN_POINT('Ctrl Pts',(0.10769043523109,1.,2.12499752307));
#26077=CARTESIAN_POINT('Ctrl Pts',(0.110350236135025,-1.,2.11926155590865));
#26078=CARTESIAN_POINT('Ctrl Pts',(0.110350236135025,1.,2.11926155590865));
#26079=CARTESIAN_POINT('Ctrl Pts',(0.112968534419737,-1.,2.11351924490306));
#26080=CARTESIAN_POINT('Ctrl Pts',(0.112968534419737,1.,2.11351924490306));
#26081=CARTESIAN_POINT('Ctrl Pts',(0.115544957687926,-1.,2.10777050261309));
#26082=CARTESIAN_POINT('Ctrl Pts',(0.115544957687926,1.,2.10777050261309));
#26083=CARTESIAN_POINT('Ctrl Pts',(0.118079107988355,-1.,2.102015121329));
#26084=CARTESIAN_POINT('Ctrl Pts',(0.118079107988355,1.,2.102015121329));
#26085=CARTESIAN_POINT('Ctrl Pts',(0.120570567965122,-1.,2.0962529286773));
#26086=CARTESIAN_POINT('Ctrl Pts',(0.120570567965122,1.,2.0962529286773));
#26087=CARTESIAN_POINT('Ctrl Pts',(0.123018905621083,-1.,2.09048392424825));
#26088=CARTESIAN_POINT('Ctrl Pts',(0.123018905621083,1.,2.09048392424825));
#26089=CARTESIAN_POINT('Ctrl Pts',(0.125423679412061,-1.,2.08470840653643));
#26090=CARTESIAN_POINT('Ctrl Pts',(0.125423679412061,1.,2.08470840653643));
#26091=CARTESIAN_POINT('Ctrl Pts',(0.12778444527612,-1.,2.07892715110987));
#26092=CARTESIAN_POINT('Ctrl Pts',(0.12778444527612,1.,2.07892715110987));
#26093=CARTESIAN_POINT('Ctrl Pts',(0.130100748328403,-1.,2.07314114713063));
#26094=CARTESIAN_POINT('Ctrl Pts',(0.130100748328403,1.,2.07314114713063));
#26095=CARTESIAN_POINT('Ctrl Pts',(0.13237211154771,-1.,2.06735123910326));
#26096=CARTESIAN_POINT('Ctrl Pts',(0.13237211154771,1.,2.06735123910326));
#26097=CARTESIAN_POINT('Ctrl Pts',(0.134598026192106,-1.,2.06155781517842));
#26098=CARTESIAN_POINT('Ctrl Pts',(0.134598026192106,1.,2.06155781517842));
#26099=CARTESIAN_POINT('Ctrl Pts',(0.136777941218043,-1.,2.05576044414264));
#26100=CARTESIAN_POINT('Ctrl Pts',(0.136777941218043,1.,2.05576044414264));
#26101=CARTESIAN_POINT('Ctrl Pts',(0.138911255368966,-1.,2.04995762001328));
#26102=CARTESIAN_POINT('Ctrl Pts',(0.138911255368966,1.,2.04995762001328));
#26103=CARTESIAN_POINT('Ctrl Pts',(0.140997332152546,-1.,2.04414757947916));
#26104=CARTESIAN_POINT('Ctrl Pts',(0.140997332152546,1.,2.04414757947916));
#26105=CARTESIAN_POINT('Ctrl Pts',(0.143035515058208,-1.,2.03832911025912));
#26106=CARTESIAN_POINT('Ctrl Pts',(0.143035515058208,1.,2.03832911025912));
#26107=CARTESIAN_POINT('Ctrl Pts',(0.145025140186057,-1.,2.03250223739942));
#26108=CARTESIAN_POINT('Ctrl Pts',(0.145025140186057,1.,2.03250223739942));
#26109=CARTESIAN_POINT('Ctrl Pts',(0.146965557332583,-1.,2.02666926182017));
#26110=CARTESIAN_POINT('Ctrl Pts',(0.146965557332583,1.,2.02666926182017));
#26111=CARTESIAN_POINT('Ctrl Pts',(0.148856124775337,-1.,2.02083464969894));
#26112=CARTESIAN_POINT('Ctrl Pts',(0.148856124775337,1.,2.02083464969894));
#26113=CARTESIAN_POINT('Ctrl Pts',(0.150696157673078,-1.,2.01500291940238));
#26114=CARTESIAN_POINT('Ctrl Pts',(0.150696157673078,1.,2.01500291940238));
#26115=CARTESIAN_POINT('Ctrl Pts',(0.152484883621449,-1.,2.00917680318424));
#26116=CARTESIAN_POINT('Ctrl Pts',(0.152484883621449,1.,2.00917680318424));
#26117=CARTESIAN_POINT('Ctrl Pts',(0.154221403049722,-1.,2.00335565310543));
#26118=CARTESIAN_POINT('Ctrl Pts',(0.154221403049722,1.,2.00335565310543));
#26119=CARTESIAN_POINT('Ctrl Pts',(0.155904629548783,-1.,1.99753284771497));
#26120=CARTESIAN_POINT('Ctrl Pts',(0.155904629548783,1.,1.99753284771497));
#26121=CARTESIAN_POINT('Ctrl Pts',(0.157533331459227,-1.,1.99169810931908));
#26122=CARTESIAN_POINT('Ctrl Pts',(0.157533331459227,1.,1.99169810931908));
#26123=CARTESIAN_POINT('Ctrl Pts',(0.159106226437299,-1.,1.98584238283292));
#26124=CARTESIAN_POINT('Ctrl Pts',(0.159106226437299,1.,1.98584238283292));
#26125=CARTESIAN_POINT('Ctrl Pts',(0.160622060784611,-1.,1.97996195437559));
#26126=CARTESIAN_POINT('Ctrl Pts',(0.160622060784611,1.,1.97996195437559));
#26127=CARTESIAN_POINT('Ctrl Pts',(0.162079693556288,-1.,1.97406280235188));
#26128=CARTESIAN_POINT('Ctrl Pts',(0.162079693556288,1.,1.97406280235188));
#26129=CARTESIAN_POINT('Ctrl Pts',(0.163478185457734,-1.,1.96816512677967));
#26130=CARTESIAN_POINT('Ctrl Pts',(0.163478185457734,1.,1.96816512677967));
#26131=CARTESIAN_POINT('Ctrl Pts',(0.164816568920269,-1.,1.96229379940136));
#26132=CARTESIAN_POINT('Ctrl Pts',(0.164816568920269,1.,1.96229379940136));
#26133=CARTESIAN_POINT('Ctrl Pts',(0.166093592002812,-1.,1.9564675971873));
#26134=CARTESIAN_POINT('Ctrl Pts',(0.166093592002812,1.,1.9564675971873));
#26135=CARTESIAN_POINT('Ctrl Pts',(0.167307501784475,-1.,1.95069027794294));
#26136=CARTESIAN_POINT('Ctrl Pts',(0.167307501784475,1.,1.95069027794294));
#26137=CARTESIAN_POINT('Ctrl Pts',(0.168455741607556,-1.,1.94493757756931));
#26138=CARTESIAN_POINT('Ctrl Pts',(0.168455741607556,1.,1.94493757756931));
#26139=CARTESIAN_POINT('Ctrl Pts',(0.16953490481749,-1.,1.93915639211581));
#26140=CARTESIAN_POINT('Ctrl Pts',(0.16953490481749,1.,1.93915639211581));
#26141=CARTESIAN_POINT('Ctrl Pts',(0.170541253116201,-1.,1.93329183155539));
#26142=CARTESIAN_POINT('Ctrl Pts',(0.170541253116201,1.,1.93329183155539));
#26143=CARTESIAN_POINT('Ctrl Pts',(0.171471191532988,-1.,1.92731093582036));
#26144=CARTESIAN_POINT('Ctrl Pts',(0.171471191532988,1.,1.92731093582036));
#26145=CARTESIAN_POINT('Ctrl Pts',(0.172321621259513,-1.,1.9212233439798));
#26146=CARTESIAN_POINT('Ctrl Pts',(0.172321621259513,1.,1.9212233439798));
#26147=CARTESIAN_POINT('Ctrl Pts',(0.173090695383496,-1.,1.91511429159527));
#26148=CARTESIAN_POINT('Ctrl Pts',(0.173090695383496,1.,1.91511429159527));
#26149=CARTESIAN_POINT('Ctrl Pts',(0.173776635257816,-1.,1.90911693975267));
#26150=CARTESIAN_POINT('Ctrl Pts',(0.173776635257816,1.,1.90911693975267));
#26151=CARTESIAN_POINT('Ctrl Pts',(0.174375518661085,-1.,1.90335253862834));
#26152=CARTESIAN_POINT('Ctrl Pts',(0.174375518661085,1.,1.90335253862834));
#26153=CARTESIAN_POINT('Ctrl Pts',(0.174879405091263,-1.,1.89788101117132));
#26154=CARTESIAN_POINT('Ctrl Pts',(0.174879405091263,1.,1.89788101117132));
#26155=CARTESIAN_POINT('Ctrl Pts',(0.175274276190844,-1.,1.892646301985));
#26156=CARTESIAN_POINT('Ctrl Pts',(0.175274276190844,1.,1.892646301985));
#26157=CARTESIAN_POINT('Ctrl Pts',(0.175538155840648,-1.,1.88742606273259));
#26158=CARTESIAN_POINT('Ctrl Pts',(0.175538155840648,1.,1.88742606273259));
#26159=CARTESIAN_POINT('Ctrl Pts',(0.175644148889698,-1.,1.88188663145367));
#26160=CARTESIAN_POINT('Ctrl Pts',(0.175644148889698,1.,1.88188663145367));
#26161=CARTESIAN_POINT('Ctrl Pts',(0.175563480746485,-1.,1.87563767773588));
#26162=CARTESIAN_POINT('Ctrl Pts',(0.175563480746485,1.,1.87563767773588));
#26163=CARTESIAN_POINT('Ctrl Pts',(0.175268337590757,-1.,1.86828349694799));
#26164=CARTESIAN_POINT('Ctrl Pts',(0.175268337590757,1.,1.86828349694799));
#26165=CARTESIAN_POINT('Ctrl Pts',(0.17473525927603,-1.,1.85948367088837));
#26166=CARTESIAN_POINT('Ctrl Pts',(0.17473525927603,1.,1.85948367088837));
#26167=CARTESIAN_POINT('Ctrl Pts',(0.173946627587731,-1.,1.8489811319852));
#26168=CARTESIAN_POINT('Ctrl Pts',(0.173946627587731,1.,1.8489811319852));
#26169=CARTESIAN_POINT('Ctrl Pts',(0.1728894428919,-1.,1.83658380527692));
#26170=CARTESIAN_POINT('Ctrl Pts',(0.1728894428919,1.,1.83658380527692));
#26171=CARTESIAN_POINT('Ctrl Pts',(0.171554770204119,-1.,1.82215766811545));
#26172=CARTESIAN_POINT('Ctrl Pts',(0.171554770204119,1.,1.82215766811545));
#26173=CARTESIAN_POINT('Ctrl Pts',(0.169936923904608,-1.,1.80561530629706));
#26174=CARTESIAN_POINT('Ctrl Pts',(0.169936923904608,1.,1.80561530629706));
#26175=CARTESIAN_POINT('Ctrl Pts',(0.168032772805197,-1.,1.7869064998507));
#26176=CARTESIAN_POINT('Ctrl Pts',(0.168032772805197,1.,1.7869064998507));
#26177=CARTESIAN_POINT('Ctrl Pts',(0.1662793551464,-1.,1.77018771684844));
#26178=CARTESIAN_POINT('Ctrl Pts',(0.1662793551464,1.,1.77018771684844));
#26179=CARTESIAN_POINT('Ctrl Pts',(0.164834765707158,-1.,1.75666056638427));
#26180=CARTESIAN_POINT('Ctrl Pts',(0.164834765707158,1.,1.75666056638427));
#26181=CARTESIAN_POINT('Ctrl Pts',(0.163814161002002,-1.,1.7472034950333));
#26182=CARTESIAN_POINT('Ctrl Pts',(0.163814161002002,1.,1.7472034950333));
#26183=CARTESIAN_POINT('Ctrl Pts',(0.163289472382896,-1.,1.74236521665491));
#26184=CARTESIAN_POINT('Ctrl Pts',(0.163289472382896,1.,1.74236521665491));
#26185=CARTESIAN_POINT('',(0.0694764450219578,1.,2.19890268624765));
#26186=CARTESIAN_POINT('Ctrl Pts',(0.0694764450219578,1.,2.19890268624765));
#26187=CARTESIAN_POINT('Ctrl Pts',(0.0701143536325487,1.,2.19777582085423));
#26188=CARTESIAN_POINT('Ctrl Pts',(0.0713863779526151,1.,2.19552129484002));
#26189=CARTESIAN_POINT('Ctrl Pts',(0.0732830357306722,1.,2.19213712013662));
#26190=CARTESIAN_POINT('Ctrl Pts',(0.0757891465836145,1.,2.1876201139953));
#26191=CARTESIAN_POINT('Ctrl Pts',(0.078883772768524,1.,2.18196589448887));
#26192=CARTESIAN_POINT('Ctrl Pts',(0.0819402680872763,1.,2.176303712113));
#26193=CARTESIAN_POINT('Ctrl Pts',(0.084958462083537,1.,2.17063357870952));
#26194=CARTESIAN_POINT('Ctrl Pts',(0.087938129138692,1.,2.16495552645014));
#26195=CARTESIAN_POINT('Ctrl Pts',(0.0908789888107263,1.,2.15926961544516));
#26196=CARTESIAN_POINT('Ctrl Pts',(0.0937807218867641,1.,2.1535759397817));
#26197=CARTESIAN_POINT('Ctrl Pts',(0.0966429852305456,1.,2.14787463531795));
#26198=CARTESIAN_POINT('Ctrl Pts',(0.0994654261990913,1.,2.14216588396025));
#26199=CARTESIAN_POINT('Ctrl Pts',(0.1022477005561,1.,2.13644992667165));
#26200=CARTESIAN_POINT('Ctrl Pts',(0.104989479152739,1.,2.13072704887293));
#26201=CARTESIAN_POINT('Ctrl Pts',(0.10769043523109,1.,2.12499752307));
#26202=CARTESIAN_POINT('Ctrl Pts',(0.110350236135025,1.,2.11926155590865));
#26203=CARTESIAN_POINT('Ctrl Pts',(0.112968534419737,1.,2.11351924490306));
#26204=CARTESIAN_POINT('Ctrl Pts',(0.115544957687926,1.,2.10777050261309));
#26205=CARTESIAN_POINT('Ctrl Pts',(0.118079107988355,1.,2.102015121329));
#26206=CARTESIAN_POINT('Ctrl Pts',(0.120570567965122,1.,2.0962529286773));
#26207=CARTESIAN_POINT('Ctrl Pts',(0.123018905621083,1.,2.09048392424825));
#26208=CARTESIAN_POINT('Ctrl Pts',(0.125423679412061,1.,2.08470840653643));
#26209=CARTESIAN_POINT('Ctrl Pts',(0.12778444527612,1.,2.07892715110987));
#26210=CARTESIAN_POINT('Ctrl Pts',(0.130100748328403,1.,2.07314114713063));
#26211=CARTESIAN_POINT('Ctrl Pts',(0.13237211154771,1.,2.06735123910326));
#26212=CARTESIAN_POINT('Ctrl Pts',(0.134598026192106,1.,2.06155781517842));
#26213=CARTESIAN_POINT('Ctrl Pts',(0.136777941218043,1.,2.05576044414264));
#26214=CARTESIAN_POINT('Ctrl Pts',(0.138911255368966,1.,2.04995762001328));
#26215=CARTESIAN_POINT('Ctrl Pts',(0.140997332152546,1.,2.04414757947916));
#26216=CARTESIAN_POINT('Ctrl Pts',(0.143035515058208,1.,2.03832911025912));
#26217=CARTESIAN_POINT('Ctrl Pts',(0.145025140186057,1.,2.03250223739942));
#26218=CARTESIAN_POINT('Ctrl Pts',(0.146965557332583,1.,2.02666926182017));
#26219=CARTESIAN_POINT('Ctrl Pts',(0.148856124775337,1.,2.02083464969894));
#26220=CARTESIAN_POINT('Ctrl Pts',(0.150696157673078,1.,2.01500291940238));
#26221=CARTESIAN_POINT('Ctrl Pts',(0.152484883621449,1.,2.00917680318424));
#26222=CARTESIAN_POINT('Ctrl Pts',(0.154221403049722,1.,2.00335565310543));
#26223=CARTESIAN_POINT('Ctrl Pts',(0.155904629548783,1.,1.99753284771497));
#26224=CARTESIAN_POINT('Ctrl Pts',(0.157533331459227,1.,1.99169810931908));
#26225=CARTESIAN_POINT('Ctrl Pts',(0.159106226437299,1.,1.98584238283292));
#26226=CARTESIAN_POINT('Ctrl Pts',(0.160622060784611,1.,1.97996195437559));
#26227=CARTESIAN_POINT('Ctrl Pts',(0.162079693556288,1.,1.97406280235188));
#26228=CARTESIAN_POINT('Ctrl Pts',(0.163478185457734,1.,1.96816512677967));
#26229=CARTESIAN_POINT('Ctrl Pts',(0.164816568920269,1.,1.96229379940136));
#26230=CARTESIAN_POINT('Ctrl Pts',(0.166093592002812,1.,1.9564675971873));
#26231=CARTESIAN_POINT('Ctrl Pts',(0.167307501784475,1.,1.95069027794294));
#26232=CARTESIAN_POINT('Ctrl Pts',(0.168455741607556,1.,1.94493757756931));
#26233=CARTESIAN_POINT('Ctrl Pts',(0.16953490481749,1.,1.93915639211581));
#26234=CARTESIAN_POINT('Ctrl Pts',(0.170541253116201,1.,1.93329183155539));
#26235=CARTESIAN_POINT('Ctrl Pts',(0.171471191532988,1.,1.92731093582036));
#26236=CARTESIAN_POINT('Ctrl Pts',(0.172321621259513,1.,1.9212233439798));
#26237=CARTESIAN_POINT('Ctrl Pts',(0.173090695383496,1.,1.91511429159527));
#26238=CARTESIAN_POINT('Ctrl Pts',(0.173776635257816,1.,1.90911693975267));
#26239=CARTESIAN_POINT('Ctrl Pts',(0.174375518661085,1.,1.90335253862834));
#26240=CARTESIAN_POINT('Ctrl Pts',(0.174879405091263,1.,1.89788101117132));
#26241=CARTESIAN_POINT('Ctrl Pts',(0.175274276190844,1.,1.892646301985));
#26242=CARTESIAN_POINT('Ctrl Pts',(0.175538155840648,1.,1.88742606273259));
#26243=CARTESIAN_POINT('Ctrl Pts',(0.175644148889698,1.,1.88188663145367));
#26244=CARTESIAN_POINT('Ctrl Pts',(0.175563480746485,1.,1.87563767773588));
#26245=CARTESIAN_POINT('Ctrl Pts',(0.175268337590757,1.,1.86828349694799));
#26246=CARTESIAN_POINT('Ctrl Pts',(0.17473525927603,1.,1.85948367088837));
#26247=CARTESIAN_POINT('Ctrl Pts',(0.173946627587731,1.,1.8489811319852));
#26248=CARTESIAN_POINT('Ctrl Pts',(0.1728894428919,1.,1.83658380527692));
#26249=CARTESIAN_POINT('Ctrl Pts',(0.171554770204119,1.,1.82215766811545));
#26250=CARTESIAN_POINT('Ctrl Pts',(0.169936923904608,1.,1.80561530629706));
#26251=CARTESIAN_POINT('Ctrl Pts',(0.168032772805197,1.,1.7869064998507));
#26252=CARTESIAN_POINT('Ctrl Pts',(0.1662793551464,1.,1.77018771684844));
#26253=CARTESIAN_POINT('Ctrl Pts',(0.164834765707158,1.,1.75666056638427));
#26254=CARTESIAN_POINT('Ctrl Pts',(0.163814161002002,1.,1.7472034950333));
#26255=CARTESIAN_POINT('Ctrl Pts',(0.163289472382896,1.,1.74236521665491));
#26256=CARTESIAN_POINT('',(0.0694764450219578,0.,2.19890268624765));
#26257=CARTESIAN_POINT('Origin',(-0.0694764450219586,0.,2.19890268624765));
#26258=CARTESIAN_POINT('',(-0.0694764450219586,1.,2.19890268624765));
#26259=CARTESIAN_POINT('',(0.0694764450219578,1.,2.19890268624765));
#26260=CARTESIAN_POINT('',(-0.0694764450219586,0.,2.19890268624765));
#26261=CARTESIAN_POINT('Ctrl Pts',(-0.163289472382896,-1.,1.74236521665491));
#26262=CARTESIAN_POINT('Ctrl Pts',(-0.163289472382896,1.,1.74236521665491));
#26263=CARTESIAN_POINT('Ctrl Pts',(-0.163814161002474,-1.,1.74720349503904));
#26264=CARTESIAN_POINT('Ctrl Pts',(-0.163814161002474,1.,1.74720349503904));
#26265=CARTESIAN_POINT('Ctrl Pts',(-0.164834765708484,-1.,1.75666056640041));
#26266=CARTESIAN_POINT('Ctrl Pts',(-0.164834765708484,1.,1.75666056640041));
#26267=CARTESIAN_POINT('Ctrl Pts',(-0.166279355148738,-1.,1.77018771687692));
#26268=CARTESIAN_POINT('Ctrl Pts',(-0.166279355148738,1.,1.77018771687692));
#26269=CARTESIAN_POINT('Ctrl Pts',(-0.16803277280837,-1.,1.78690649988931));
#26270=CARTESIAN_POINT('Ctrl Pts',(-0.16803277280837,1.,1.78690649988931));
#26271=CARTESIAN_POINT('Ctrl Pts',(-0.169936923908078,-1.,1.80561530633924));
#26272=CARTESIAN_POINT('Ctrl Pts',(-0.169936923908078,1.,1.80561530633924));
#26273=CARTESIAN_POINT('Ctrl Pts',(-0.171554770207306,-1.,1.82215766815414));
#26274=CARTESIAN_POINT('Ctrl Pts',(-0.171554770207306,1.,1.82215766815414));
#26275=CARTESIAN_POINT('Ctrl Pts',(-0.17288944289442,-1.,1.83658380530747));
#26276=CARTESIAN_POINT('Ctrl Pts',(-0.17288944289442,1.,1.83658380530747));
#26277=CARTESIAN_POINT('Ctrl Pts',(-0.173946627589401,-1.,1.84898113200543));
#26278=CARTESIAN_POINT('Ctrl Pts',(-0.173946627589401,1.,1.84898113200543));
#26279=CARTESIAN_POINT('Ctrl Pts',(-0.174735259276856,-1.,1.85948367089838));
#26280=CARTESIAN_POINT('Ctrl Pts',(-0.174735259276856,1.,1.85948367089838));
#26281=CARTESIAN_POINT('Ctrl Pts',(-0.175268337590901,-1.,1.86828349694972));
#26282=CARTESIAN_POINT('Ctrl Pts',(-0.175268337590901,1.,1.86828349694972));
#26283=CARTESIAN_POINT('Ctrl Pts',(-0.175563480746206,-1.,1.87563767773249));
#26284=CARTESIAN_POINT('Ctrl Pts',(-0.175563480746206,1.,1.87563767773249));
#26285=CARTESIAN_POINT('Ctrl Pts',(-0.175644148889271,-1.,1.88188663144846));
#26286=CARTESIAN_POINT('Ctrl Pts',(-0.175644148889271,1.,1.88188663144846));
#26287=CARTESIAN_POINT('Ctrl Pts',(-0.175538155840286,-1.,1.88742606272818));
#26288=CARTESIAN_POINT('Ctrl Pts',(-0.175538155840286,1.,1.88742606272818));
#26289=CARTESIAN_POINT('Ctrl Pts',(-0.175274276190664,-1.,1.89264630198279));
#26290=CARTESIAN_POINT('Ctrl Pts',(-0.175274276190664,1.,1.89264630198279));
#26291=CARTESIAN_POINT('Ctrl Pts',(-0.174879405091277,-1.,1.89788101117148));
#26292=CARTESIAN_POINT('Ctrl Pts',(-0.174879405091277,1.,1.89788101117148));
#26293=CARTESIAN_POINT('Ctrl Pts',(-0.174375518661222,-1.,1.90335253863003));
#26294=CARTESIAN_POINT('Ctrl Pts',(-0.174375518661222,1.,1.90335253863003));
#26295=CARTESIAN_POINT('Ctrl Pts',(-0.173776635257984,-1.,1.90911693975475));
#26296=CARTESIAN_POINT('Ctrl Pts',(-0.173776635257984,1.,1.90911693975475));
#26297=CARTESIAN_POINT('Ctrl Pts',(-0.173090695383619,-1.,1.91511429159681));
#26298=CARTESIAN_POINT('Ctrl Pts',(-0.173090695383619,1.,1.91511429159681));
#26299=CARTESIAN_POINT('Ctrl Pts',(-0.172321621259557,-1.,1.92122334398034));
#26300=CARTESIAN_POINT('Ctrl Pts',(-0.172321621259557,1.,1.92122334398034));
#26301=CARTESIAN_POINT('Ctrl Pts',(-0.17147119153296,-1.,1.92731093582));
#26302=CARTESIAN_POINT('Ctrl Pts',(-0.17147119153296,1.,1.92731093582));
#26303=CARTESIAN_POINT('Ctrl Pts',(-0.170541253116136,-1.,1.93329183155455));
#26304=CARTESIAN_POINT('Ctrl Pts',(-0.170541253116136,1.,1.93329183155455));
#26305=CARTESIAN_POINT('Ctrl Pts',(-0.169534904817425,-1.,1.93915639211497));
#26306=CARTESIAN_POINT('Ctrl Pts',(-0.169534904817425,1.,1.93915639211497));
#26307=CARTESIAN_POINT('Ctrl Pts',(-0.168455741607516,-1.,1.94493757756879));
#26308=CARTESIAN_POINT('Ctrl Pts',(-0.168455741607516,1.,1.94493757756879));
#26309=CARTESIAN_POINT('Ctrl Pts',(-0.167307501784469,-1.,1.95069027794286));
#26310=CARTESIAN_POINT('Ctrl Pts',(-0.167307501784469,1.,1.95069027794286));
#26311=CARTESIAN_POINT('Ctrl Pts',(-0.166093592002833,-1.,1.95646759718755));
#26312=CARTESIAN_POINT('Ctrl Pts',(-0.166093592002833,1.,1.95646759718755));
#26313=CARTESIAN_POINT('Ctrl Pts',(-0.1648165689203,-1.,1.96229379940174));
#26314=CARTESIAN_POINT('Ctrl Pts',(-0.1648165689203,1.,1.96229379940174));
#26315=CARTESIAN_POINT('Ctrl Pts',(-0.16347818545776,-1.,1.96816512678));
#26316=CARTESIAN_POINT('Ctrl Pts',(-0.16347818545776,1.,1.96816512678));
#26317=CARTESIAN_POINT('Ctrl Pts',(-0.162079693556302,-1.,1.97406280235204));
#26318=CARTESIAN_POINT('Ctrl Pts',(-0.162079693556302,1.,1.97406280235204));
#26319=CARTESIAN_POINT('Ctrl Pts',(-0.16062206078461,-1.,1.97996195437557));
#26320=CARTESIAN_POINT('Ctrl Pts',(-0.16062206078461,1.,1.97996195437557));
#26321=CARTESIAN_POINT('Ctrl Pts',(-0.159106226437289,-1.,1.98584238283279));
#26322=CARTESIAN_POINT('Ctrl Pts',(-0.159106226437289,1.,1.98584238283279));
#26323=CARTESIAN_POINT('Ctrl Pts',(-0.157533331459215,-1.,1.99169810931893));
#26324=CARTESIAN_POINT('Ctrl Pts',(-0.157533331459215,1.,1.99169810931893));
#26325=CARTESIAN_POINT('Ctrl Pts',(-0.155904629548775,-1.,1.99753284771487));
#26326=CARTESIAN_POINT('Ctrl Pts',(-0.155904629548775,1.,1.99753284771487));
#26327=CARTESIAN_POINT('Ctrl Pts',(-0.154221403049719,-1.,2.00335565310539));
#26328=CARTESIAN_POINT('Ctrl Pts',(-0.154221403049719,1.,2.00335565310539));
#26329=CARTESIAN_POINT('Ctrl Pts',(-0.152484883621452,-1.,2.00917680318426));
#26330=CARTESIAN_POINT('Ctrl Pts',(-0.152484883621452,1.,2.00917680318426));
#26331=CARTESIAN_POINT('Ctrl Pts',(-0.150696157673084,-1.,2.01500291940243));
#26332=CARTESIAN_POINT('Ctrl Pts',(-0.150696157673084,1.,2.01500291940243));
#26333=CARTESIAN_POINT('Ctrl Pts',(-0.148856124775343,-1.,2.02083464969897));
#26334=CARTESIAN_POINT('Ctrl Pts',(-0.148856124775343,1.,2.02083464969897));
#26335=CARTESIAN_POINT('Ctrl Pts',(-0.146965557332586,-1.,2.02666926182017));
#26336=CARTESIAN_POINT('Ctrl Pts',(-0.146965557332586,1.,2.02666926182017));
#26337=CARTESIAN_POINT('Ctrl Pts',(-0.145025140186058,-1.,2.03250223739941));
#26338=CARTESIAN_POINT('Ctrl Pts',(-0.145025140186058,1.,2.03250223739941));
#26339=CARTESIAN_POINT('Ctrl Pts',(-0.143035515058208,-1.,2.03832911025913));
#26340=CARTESIAN_POINT('Ctrl Pts',(-0.143035515058208,1.,2.03832911025913));
#26341=CARTESIAN_POINT('Ctrl Pts',(-0.140997332152546,-1.,2.04414757947919));
#26342=CARTESIAN_POINT('Ctrl Pts',(-0.140997332152546,1.,2.04414757947919));
#26343=CARTESIAN_POINT('Ctrl Pts',(-0.138911255368966,-1.,2.04995762001333));
#26344=CARTESIAN_POINT('Ctrl Pts',(-0.138911255368966,1.,2.04995762001333));
#26345=CARTESIAN_POINT('Ctrl Pts',(-0.136777941218044,-1.,2.0557604441427));
#26346=CARTESIAN_POINT('Ctrl Pts',(-0.136777941218044,1.,2.0557604441427));
#26347=CARTESIAN_POINT('Ctrl Pts',(-0.134598026192107,-1.,2.06155781517844));
#26348=CARTESIAN_POINT('Ctrl Pts',(-0.134598026192107,1.,2.06155781517844));
#26349=CARTESIAN_POINT('Ctrl Pts',(-0.13237211154771,-1.,2.06735123910319));
#26350=CARTESIAN_POINT('Ctrl Pts',(-0.13237211154771,1.,2.06735123910319));
#26351=CARTESIAN_POINT('Ctrl Pts',(-0.130100748328401,-1.,2.07314114713047));
#26352=CARTESIAN_POINT('Ctrl Pts',(-0.130100748328401,1.,2.07314114713047));
#26353=CARTESIAN_POINT('Ctrl Pts',(-0.127784445276116,-1.,2.07892715110967));
#26354=CARTESIAN_POINT('Ctrl Pts',(-0.127784445276116,1.,2.07892715110967));
#26355=CARTESIAN_POINT('Ctrl Pts',(-0.125423679412058,-1.,2.08470840653628));
#26356=CARTESIAN_POINT('Ctrl Pts',(-0.125423679412058,1.,2.08470840653628));
#26357=CARTESIAN_POINT('Ctrl Pts',(-0.123018905621083,-1.,2.09048392424826));
#26358=CARTESIAN_POINT('Ctrl Pts',(-0.123018905621083,1.,2.09048392424826));
#26359=CARTESIAN_POINT('Ctrl Pts',(-0.120570567965129,-1.,2.09625292867756));
#26360=CARTESIAN_POINT('Ctrl Pts',(-0.120570567965129,1.,2.09625292867756));
#26361=CARTESIAN_POINT('Ctrl Pts',(-0.118079107988368,-1.,2.10201512132945));
#26362=CARTESIAN_POINT('Ctrl Pts',(-0.118079107988368,1.,2.10201512132945));
#26363=CARTESIAN_POINT('Ctrl Pts',(-0.115544957687941,-1.,2.10777050261359));
#26364=CARTESIAN_POINT('Ctrl Pts',(-0.115544957687941,1.,2.10777050261359));
#26365=CARTESIAN_POINT('Ctrl Pts',(-0.112968534419746,-1.,2.11351924490335));
#26366=CARTESIAN_POINT('Ctrl Pts',(-0.112968534419746,1.,2.11351924490335));
#26367=CARTESIAN_POINT('Ctrl Pts',(-0.11035023613502,-1.,2.11926155590849));
#26368=CARTESIAN_POINT('Ctrl Pts',(-0.11035023613502,1.,2.11926155590849));
#26369=CARTESIAN_POINT('Ctrl Pts',(-0.107690435231068,-1.,2.12499752306927));
#26370=CARTESIAN_POINT('Ctrl Pts',(-0.107690435231068,1.,2.12499752306927));
#26371=CARTESIAN_POINT('Ctrl Pts',(-0.104989479152703,-1.,2.1307270488718));
#26372=CARTESIAN_POINT('Ctrl Pts',(-0.104989479152703,1.,2.1307270488718));
#26373=CARTESIAN_POINT('Ctrl Pts',(-0.102247700556064,-1.,2.13644992667052));
#26374=CARTESIAN_POINT('Ctrl Pts',(-0.102247700556064,1.,2.13644992667052));
#26375=CARTESIAN_POINT('Ctrl Pts',(-0.0994654261990745,-1.,2.14216588395974));
#26376=CARTESIAN_POINT('Ctrl Pts',(-0.0994654261990745,1.,2.14216588395974));
#26377=CARTESIAN_POINT('Ctrl Pts',(-0.0966429852305691,-1.,2.14787463531864));
#26378=CARTESIAN_POINT('Ctrl Pts',(-0.0966429852305691,1.,2.14787463531864));
#26379=CARTESIAN_POINT('Ctrl Pts',(-0.0937807218868348,-1.,2.15357593978377));
#26380=CARTESIAN_POINT('Ctrl Pts',(-0.0937807218868348,1.,2.15357593978377));
#26381=CARTESIAN_POINT('Ctrl Pts',(-0.0908789888108269,-1.,2.15926961544808));
#26382=CARTESIAN_POINT('Ctrl Pts',(-0.0908789888108269,1.,2.15926961544808));
#26383=CARTESIAN_POINT('Ctrl Pts',(-0.0879381291387825,-1.,2.16495552645275));
#26384=CARTESIAN_POINT('Ctrl Pts',(-0.0879381291387825,1.,2.16495552645275));
#26385=CARTESIAN_POINT('Ctrl Pts',(-0.0849584620835646,-1.,2.17063357871031));
#26386=CARTESIAN_POINT('Ctrl Pts',(-0.0849584620835646,1.,2.17063357871031));
#26387=CARTESIAN_POINT('Ctrl Pts',(-0.0819402680871942,-1.,2.1763037121106));
#26388=CARTESIAN_POINT('Ctrl Pts',(-0.0819402680871942,1.,2.1763037121106));
#26389=CARTESIAN_POINT('Ctrl Pts',(-0.078883772768323,-1.,2.18196589448304));
#26390=CARTESIAN_POINT('Ctrl Pts',(-0.078883772768323,1.,2.18196589448304));
#26391=CARTESIAN_POINT('Ctrl Pts',(-0.0757891465833414,-1.,2.1876201139874));
#26392=CARTESIAN_POINT('Ctrl Pts',(-0.0757891465833414,1.,2.1876201139874));
#26393=CARTESIAN_POINT('Ctrl Pts',(-0.0732830357304279,-1.,2.19213712012956));
#26394=CARTESIAN_POINT('Ctrl Pts',(-0.0732830357304279,1.,2.19213712012956));
#26395=CARTESIAN_POINT('Ctrl Pts',(-0.071386377952463,-1.,2.19552129483562));
#26396=CARTESIAN_POINT('Ctrl Pts',(-0.071386377952463,1.,2.19552129483562));
#26397=CARTESIAN_POINT('Ctrl Pts',(-0.0701143536324929,-1.,2.19777582085261));
#26398=CARTESIAN_POINT('Ctrl Pts',(-0.0701143536324929,1.,2.19777582085261));
#26399=CARTESIAN_POINT('Ctrl Pts',(-0.0694764450219586,-1.,2.19890268624765));
#26400=CARTESIAN_POINT('Ctrl Pts',(-0.0694764450219586,1.,2.19890268624765));
#26401=CARTESIAN_POINT('',(-0.163289472382896,1.,1.74236521665491));
#26402=CARTESIAN_POINT('Ctrl Pts',(-0.163289472382896,1.,1.74236521665491));
#26403=CARTESIAN_POINT('Ctrl Pts',(-0.163814161002474,1.,1.74720349503904));
#26404=CARTESIAN_POINT('Ctrl Pts',(-0.164834765708484,1.,1.75666056640041));
#26405=CARTESIAN_POINT('Ctrl Pts',(-0.166279355148738,1.,1.77018771687692));
#26406=CARTESIAN_POINT('Ctrl Pts',(-0.16803277280837,1.,1.78690649988931));
#26407=CARTESIAN_POINT('Ctrl Pts',(-0.169936923908078,1.,1.80561530633924));
#26408=CARTESIAN_POINT('Ctrl Pts',(-0.171554770207306,1.,1.82215766815414));
#26409=CARTESIAN_POINT('Ctrl Pts',(-0.17288944289442,1.,1.83658380530747));
#26410=CARTESIAN_POINT('Ctrl Pts',(-0.173946627589401,1.,1.84898113200543));
#26411=CARTESIAN_POINT('Ctrl Pts',(-0.174735259276856,1.,1.85948367089838));
#26412=CARTESIAN_POINT('Ctrl Pts',(-0.175268337590901,1.,1.86828349694972));
#26413=CARTESIAN_POINT('Ctrl Pts',(-0.175563480746206,1.,1.87563767773249));
#26414=CARTESIAN_POINT('Ctrl Pts',(-0.175644148889271,1.,1.88188663144846));
#26415=CARTESIAN_POINT('Ctrl Pts',(-0.175538155840286,1.,1.88742606272818));
#26416=CARTESIAN_POINT('Ctrl Pts',(-0.175274276190664,1.,1.89264630198279));
#26417=CARTESIAN_POINT('Ctrl Pts',(-0.174879405091277,1.,1.89788101117148));
#26418=CARTESIAN_POINT('Ctrl Pts',(-0.174375518661222,1.,1.90335253863003));
#26419=CARTESIAN_POINT('Ctrl Pts',(-0.173776635257984,1.,1.90911693975475));
#26420=CARTESIAN_POINT('Ctrl Pts',(-0.173090695383619,1.,1.91511429159681));
#26421=CARTESIAN_POINT('Ctrl Pts',(-0.172321621259557,1.,1.92122334398034));
#26422=CARTESIAN_POINT('Ctrl Pts',(-0.17147119153296,1.,1.92731093582));
#26423=CARTESIAN_POINT('Ctrl Pts',(-0.170541253116136,1.,1.93329183155455));
#26424=CARTESIAN_POINT('Ctrl Pts',(-0.169534904817425,1.,1.93915639211497));
#26425=CARTESIAN_POINT('Ctrl Pts',(-0.168455741607516,1.,1.94493757756879));
#26426=CARTESIAN_POINT('Ctrl Pts',(-0.167307501784469,1.,1.95069027794286));
#26427=CARTESIAN_POINT('Ctrl Pts',(-0.166093592002833,1.,1.95646759718755));
#26428=CARTESIAN_POINT('Ctrl Pts',(-0.1648165689203,1.,1.96229379940174));
#26429=CARTESIAN_POINT('Ctrl Pts',(-0.16347818545776,1.,1.96816512678));
#26430=CARTESIAN_POINT('Ctrl Pts',(-0.162079693556302,1.,1.97406280235204));
#26431=CARTESIAN_POINT('Ctrl Pts',(-0.16062206078461,1.,1.97996195437557));
#26432=CARTESIAN_POINT('Ctrl Pts',(-0.159106226437289,1.,1.98584238283279));
#26433=CARTESIAN_POINT('Ctrl Pts',(-0.157533331459215,1.,1.99169810931893));
#26434=CARTESIAN_POINT('Ctrl Pts',(-0.155904629548775,1.,1.99753284771487));
#26435=CARTESIAN_POINT('Ctrl Pts',(-0.154221403049719,1.,2.00335565310539));
#26436=CARTESIAN_POINT('Ctrl Pts',(-0.152484883621452,1.,2.00917680318426));
#26437=CARTESIAN_POINT('Ctrl Pts',(-0.150696157673084,1.,2.01500291940243));
#26438=CARTESIAN_POINT('Ctrl Pts',(-0.148856124775343,1.,2.02083464969897));
#26439=CARTESIAN_POINT('Ctrl Pts',(-0.146965557332586,1.,2.02666926182017));
#26440=CARTESIAN_POINT('Ctrl Pts',(-0.145025140186058,1.,2.03250223739941));
#26441=CARTESIAN_POINT('Ctrl Pts',(-0.143035515058208,1.,2.03832911025913));
#26442=CARTESIAN_POINT('Ctrl Pts',(-0.140997332152546,1.,2.04414757947919));
#26443=CARTESIAN_POINT('Ctrl Pts',(-0.138911255368966,1.,2.04995762001333));
#26444=CARTESIAN_POINT('Ctrl Pts',(-0.136777941218044,1.,2.0557604441427));
#26445=CARTESIAN_POINT('Ctrl Pts',(-0.134598026192107,1.,2.06155781517844));
#26446=CARTESIAN_POINT('Ctrl Pts',(-0.13237211154771,1.,2.06735123910319));
#26447=CARTESIAN_POINT('Ctrl Pts',(-0.130100748328401,1.,2.07314114713047));
#26448=CARTESIAN_POINT('Ctrl Pts',(-0.127784445276116,1.,2.07892715110967));
#26449=CARTESIAN_POINT('Ctrl Pts',(-0.125423679412058,1.,2.08470840653628));
#26450=CARTESIAN_POINT('Ctrl Pts',(-0.123018905621083,1.,2.09048392424826));
#26451=CARTESIAN_POINT('Ctrl Pts',(-0.120570567965129,1.,2.09625292867756));
#26452=CARTESIAN_POINT('Ctrl Pts',(-0.118079107988368,1.,2.10201512132945));
#26453=CARTESIAN_POINT('Ctrl Pts',(-0.115544957687941,1.,2.10777050261359));
#26454=CARTESIAN_POINT('Ctrl Pts',(-0.112968534419746,1.,2.11351924490335));
#26455=CARTESIAN_POINT('Ctrl Pts',(-0.11035023613502,1.,2.11926155590849));
#26456=CARTESIAN_POINT('Ctrl Pts',(-0.107690435231068,1.,2.12499752306927));
#26457=CARTESIAN_POINT('Ctrl Pts',(-0.104989479152703,1.,2.1307270488718));
#26458=CARTESIAN_POINT('Ctrl Pts',(-0.102247700556064,1.,2.13644992667052));
#26459=CARTESIAN_POINT('Ctrl Pts',(-0.0994654261990745,1.,2.14216588395974));
#26460=CARTESIAN_POINT('Ctrl Pts',(-0.0966429852305691,1.,2.14787463531864));
#26461=CARTESIAN_POINT('Ctrl Pts',(-0.0937807218868348,1.,2.15357593978377));
#26462=CARTESIAN_POINT('Ctrl Pts',(-0.0908789888108269,1.,2.15926961544808));
#26463=CARTESIAN_POINT('Ctrl Pts',(-0.0879381291387825,1.,2.16495552645275));
#26464=CARTESIAN_POINT('Ctrl Pts',(-0.0849584620835646,1.,2.17063357871031));
#26465=CARTESIAN_POINT('Ctrl Pts',(-0.0819402680871942,1.,2.1763037121106));
#26466=CARTESIAN_POINT('Ctrl Pts',(-0.078883772768323,1.,2.18196589448304));
#26467=CARTESIAN_POINT('Ctrl Pts',(-0.0757891465833414,1.,2.1876201139874));
#26468=CARTESIAN_POINT('Ctrl Pts',(-0.0732830357304279,1.,2.19213712012956));
#26469=CARTESIAN_POINT('Ctrl Pts',(-0.071386377952463,1.,2.19552129483562));
#26470=CARTESIAN_POINT('Ctrl Pts',(-0.0701143536324929,1.,2.19777582085261));
#26471=CARTESIAN_POINT('Ctrl Pts',(-0.0694764450219586,1.,2.19890268624765));
#26472=CARTESIAN_POINT('',(-0.163289472382897,0.,1.74236521665491));
#26473=CARTESIAN_POINT('Origin',(0.,0.,0.));
#26474=CARTESIAN_POINT('',(-0.383122945602004,1.,1.7075470150345));
#26475=CARTESIAN_POINT('Origin',(0.,1.,0.));
#26476=CARTESIAN_POINT('',(-0.383122945602004,0.,1.7075470150345));
#26477=CARTESIAN_POINT('Ctrl Pts',(-0.61342227326009,-1.,2.11275013067528));
#26478=CARTESIAN_POINT('Ctrl Pts',(-0.61342227326009,1.,2.11275013067528));
#26479=CARTESIAN_POINT('Ctrl Pts',(-0.61246736556225,-1.,2.11187554260142));
#26480=CARTESIAN_POINT('Ctrl Pts',(-0.61246736556225,1.,2.11187554260142));
#26481=CARTESIAN_POINT('Ctrl Pts',(-0.610560911691113,-1.,2.11012443807661));
#26482=CARTESIAN_POINT('Ctrl Pts',(-0.610560911691113,1.,2.11012443807661));
#26483=CARTESIAN_POINT('Ctrl Pts',(-0.607711315456826,-1.,2.10749199615859));
#26484=CARTESIAN_POINT('Ctrl Pts',(-0.607711315456826,1.,2.10749199615859));
#26485=CARTESIAN_POINT('Ctrl Pts',(-0.603932030738212,-1.,2.10397049887709));
#26486=CARTESIAN_POINT('Ctrl Pts',(-0.603932030738212,1.,2.10397049887709));
#26487=CARTESIAN_POINT('Ctrl Pts',(-0.599241616422144,-1.,2.09954930865331));
#26488=CARTESIAN_POINT('Ctrl Pts',(-0.599241616422144,1.,2.09954930865331));
#26489=CARTESIAN_POINT('Ctrl Pts',(-0.594585006052824,-1.,2.09510876220501));
#26490=CARTESIAN_POINT('Ctrl Pts',(-0.594585006052824,1.,2.09510876220501));
#26491=CARTESIAN_POINT('Ctrl Pts',(-0.589962365403189,-1.,2.09064881812053));
#26492=CARTESIAN_POINT('Ctrl Pts',(-0.589962365403189,1.,2.09064881812053));
#26493=CARTESIAN_POINT('Ctrl Pts',(-0.585373918990895,-1.,2.086169437277));
#26494=CARTESIAN_POINT('Ctrl Pts',(-0.585373918990895,1.,2.086169437277));
#26495=CARTESIAN_POINT('Ctrl Pts',(-0.580819952107257,-1.,2.08167059018138));
#26496=CARTESIAN_POINT('Ctrl Pts',(-0.580819952107257,1.,2.08167059018138));
#26497=CARTESIAN_POINT('Ctrl Pts',(-0.576300797416275,-1.,2.07715226767361));
#26498=CARTESIAN_POINT('Ctrl Pts',(-0.576300797416275,1.,2.07715226767361));
#26499=CARTESIAN_POINT('Ctrl Pts',(-0.571816823242411,-1.,2.07261449292757));
#26500=CARTESIAN_POINT('Ctrl Pts',(-0.571816823242411,1.,2.07261449292757));
#26501=CARTESIAN_POINT('Ctrl Pts',(-0.567368421181229,-1.,2.06805732997383));
#26502=CARTESIAN_POINT('Ctrl Pts',(-0.567368421181229,1.,2.06805732997383));
#26503=CARTESIAN_POINT('Ctrl Pts',(-0.562955993082574,-1.,2.06348090160697));
#26504=CARTESIAN_POINT('Ctrl Pts',(-0.562955993082574,1.,2.06348090160697));
#26505=CARTESIAN_POINT('Ctrl Pts',(-0.558579940185467,-1.,2.05888537756571));
#26506=CARTESIAN_POINT('Ctrl Pts',(-0.558579940185467,1.,2.05888537756571));
#26507=CARTESIAN_POINT('Ctrl Pts',(-0.55424065746411,-1.,2.05427091604482));
#26508=CARTESIAN_POINT('Ctrl Pts',(-0.55424065746411,1.,2.05427091604482));
#26509=CARTESIAN_POINT('Ctrl Pts',(-0.549938525150342,-1.,2.04963761077974));
#26510=CARTESIAN_POINT('Ctrl Pts',(-0.549938525150342,1.,2.04963761077974));
#26511=CARTESIAN_POINT('Ctrl Pts',(-0.545673903817348,-1.,2.0449854471456));
#26512=CARTESIAN_POINT('Ctrl Pts',(-0.545673903817348,1.,2.0449854471456));
#26513=CARTESIAN_POINT('Ctrl Pts',(-0.54144712061552,-1.,2.0403142269048));
#26514=CARTESIAN_POINT('Ctrl Pts',(-0.54144712061552,1.,2.0403142269048));
#26515=CARTESIAN_POINT('Ctrl Pts',(-0.537258489833134,-1.,2.03562362953993));
#26516=CARTESIAN_POINT('Ctrl Pts',(-0.537258489833134,1.,2.03562362953993));
#26517=CARTESIAN_POINT('Ctrl Pts',(-0.533108355132905,-1.,2.03091336214401));
#26518=CARTESIAN_POINT('Ctrl Pts',(-0.533108355132905,1.,2.03091336214401));
#26519=CARTESIAN_POINT('Ctrl Pts',(-0.528997127241911,-1.,2.02618329083289));
#26520=CARTESIAN_POINT('Ctrl Pts',(-0.528997127241911,1.,2.02618329083289));
#26521=CARTESIAN_POINT('Ctrl Pts',(-0.524925318333518,-1.,2.02143356304712));
#26522=CARTESIAN_POINT('Ctrl Pts',(-0.524925318333518,1.,2.02143356304712));
#26523=CARTESIAN_POINT('Ctrl Pts',(-0.520893590399428,-1.,2.01666477917305));
#26524=CARTESIAN_POINT('Ctrl Pts',(-0.520893590399428,1.,2.01666477917305));
#26525=CARTESIAN_POINT('Ctrl Pts',(-0.516902681728733,-1.,2.01187773939257));
#26526=CARTESIAN_POINT('Ctrl Pts',(-0.516902681728733,1.,2.01187773939257));
#26527=CARTESIAN_POINT('Ctrl Pts',(-0.512953306961814,-1.,2.00707309946955));
#26528=CARTESIAN_POINT('Ctrl Pts',(-0.512953306961814,1.,2.00707309946955));
#26529=CARTESIAN_POINT('Ctrl Pts',(-0.509046069886152,-1.,2.00225107134733));
#26530=CARTESIAN_POINT('Ctrl Pts',(-0.509046069886152,1.,2.00225107134733));
#26531=CARTESIAN_POINT('Ctrl Pts',(-0.505181361323011,-1.,1.99741107463567));
#26532=CARTESIAN_POINT('Ctrl Pts',(-0.505181361323011,1.,1.99741107463567));
#26533=CARTESIAN_POINT('Ctrl Pts',(-0.501359287727129,-1.,1.9925514912615));
#26534=CARTESIAN_POINT('Ctrl Pts',(-0.501359287727129,1.,1.9925514912615));
#26535=CARTESIAN_POINT('Ctrl Pts',(-0.497579909545564,-1.,1.98767044752929));
#26536=CARTESIAN_POINT('Ctrl Pts',(-0.497579909545564,1.,1.98767044752929));
#26537=CARTESIAN_POINT('Ctrl Pts',(-0.493843476541492,-1.,1.9827665876182));
#26538=CARTESIAN_POINT('Ctrl Pts',(-0.493843476541492,1.,1.9827665876182));
#26539=CARTESIAN_POINT('Ctrl Pts',(-0.490150627860955,-1.,1.97783973019229));
#26540=CARTESIAN_POINT('Ctrl Pts',(-0.490150627860955,1.,1.97783973019229));
#26541=CARTESIAN_POINT('Ctrl Pts',(-0.486502692907661,-1.,1.97289186263272));
#26542=CARTESIAN_POINT('Ctrl Pts',(-0.486502692907661,1.,1.97289186263272));
#26543=CARTESIAN_POINT('Ctrl Pts',(-0.482901662120687,-1.,1.96792703422358));
#26544=CARTESIAN_POINT('Ctrl Pts',(-0.482901662120687,1.,1.96792703422358));
#26545=CARTESIAN_POINT('Ctrl Pts',(-0.479349583074846,-1.,1.96294933055938));
#26546=CARTESIAN_POINT('Ctrl Pts',(-0.479349583074846,1.,1.96294933055938));
#26547=CARTESIAN_POINT('Ctrl Pts',(-0.475848034683172,-1.,1.95796111148175));
#26548=CARTESIAN_POINT('Ctrl Pts',(-0.475848034683172,1.,1.95796111148175));
#26549=CARTESIAN_POINT('Ctrl Pts',(-0.47239767226408,-1.,1.95296148278136));
#26550=CARTESIAN_POINT('Ctrl Pts',(-0.47239767226408,1.,1.95296148278136));
#26551=CARTESIAN_POINT('Ctrl Pts',(-0.468997482913158,-1.,1.94794381136524));
#26552=CARTESIAN_POINT('Ctrl Pts',(-0.468997482913158,1.,1.94794381136524));
#26553=CARTESIAN_POINT('Ctrl Pts',(-0.465645462026065,-1.,1.94289794196205));
#26554=CARTESIAN_POINT('Ctrl Pts',(-0.465645462026065,1.,1.94289794196205));
#26555=CARTESIAN_POINT('Ctrl Pts',(-0.462340031009087,-1.,1.93781486640834));
#26556=CARTESIAN_POINT('Ctrl Pts',(-0.462340031009087,1.,1.93781486640834));
#26557=CARTESIAN_POINT('Ctrl Pts',(-0.459081234547931,-1.,1.93269066517936));
#26558=CARTESIAN_POINT('Ctrl Pts',(-0.459081234547931,1.,1.93269066517936));
#26559=CARTESIAN_POINT('Ctrl Pts',(-0.455872005174335,-1.,1.92753067150461));
#26560=CARTESIAN_POINT('Ctrl Pts',(-0.455872005174335,1.,1.92753067150461));
#26561=CARTESIAN_POINT('Ctrl Pts',(-0.452719478359356,-1.,1.9223538064847));
#26562=CARTESIAN_POINT('Ctrl Pts',(-0.452719478359356,1.,1.9223538064847));
#26563=CARTESIAN_POINT('Ctrl Pts',(-0.449632260106572,-1.,1.91718342555717));
#26564=CARTESIAN_POINT('Ctrl Pts',(-0.449632260106572,1.,1.91718342555717));
#26565=CARTESIAN_POINT('Ctrl Pts',(-0.446617343485651,-1.,1.91203699981095));
#26566=CARTESIAN_POINT('Ctrl Pts',(-0.446617343485651,1.,1.91203699981095));
#26567=CARTESIAN_POINT('Ctrl Pts',(-0.44367755684917,-1.,1.90691756144906));
#26568=CARTESIAN_POINT('Ctrl Pts',(-0.44367755684917,1.,1.90691756144906));
#26569=CARTESIAN_POINT('Ctrl Pts',(-0.440807833704161,-1.,1.90180124389137));
#26570=CARTESIAN_POINT('Ctrl Pts',(-0.440807833704161,1.,1.90180124389137));
#26571=CARTESIAN_POINT('Ctrl Pts',(-0.437995003948443,-1.,1.89663648956549));
#26572=CARTESIAN_POINT('Ctrl Pts',(-0.437995003948443,1.,1.89663648956549));
#26573=CARTESIAN_POINT('Ctrl Pts',(-0.43522566096358,-1.,1.89136993975585));
#26574=CARTESIAN_POINT('Ctrl Pts',(-0.43522566096358,1.,1.89136993975585));
#26575=CARTESIAN_POINT('Ctrl Pts',(-0.432493038548833,-1.,1.88596913666828));
#26576=CARTESIAN_POINT('Ctrl Pts',(-0.432493038548833,1.,1.88596913666828));
#26577=CARTESIAN_POINT('Ctrl Pts',(-0.429803062482217,-1.,1.88044229001778));
#26578=CARTESIAN_POINT('Ctrl Pts',(-0.429803062482217,1.,1.88044229001778));
#26579=CARTESIAN_POINT('Ctrl Pts',(-0.427183828518743,-1.,1.87486989291333));
#26580=CARTESIAN_POINT('Ctrl Pts',(-0.427183828518743,1.,1.87486989291333));
#26581=CARTESIAN_POINT('Ctrl Pts',(-0.424678177290876,-1.,1.8693780394412));
#26582=CARTESIAN_POINT('Ctrl Pts',(-0.424678177290876,1.,1.8693780394412));
#26583=CARTESIAN_POINT('Ctrl Pts',(-0.422327307417885,-1.,1.86408083333863));
#26584=CARTESIAN_POINT('Ctrl Pts',(-0.422327307417885,1.,1.86408083333863));
#26585=CARTESIAN_POINT('Ctrl Pts',(-0.420157287975583,-1.,1.8590328109667));
#26586=CARTESIAN_POINT('Ctrl Pts',(-0.420157287975583,1.,1.8590328109667));
#26587=CARTESIAN_POINT('Ctrl Pts',(-0.418164129144045,-1.,1.8541763285645));
#26588=CARTESIAN_POINT('Ctrl Pts',(-0.418164129144045,1.,1.8541763285645));
#26589=CARTESIAN_POINT('Ctrl Pts',(-0.416300022039885,-1.,1.84929312930314));
#26590=CARTESIAN_POINT('Ctrl Pts',(-0.416300022039885,1.,1.84929312930314));
#26591=CARTESIAN_POINT('Ctrl Pts',(-0.414487438255542,-1.,1.84405757074218));
#26592=CARTESIAN_POINT('Ctrl Pts',(-0.414487438255542,1.,1.84405757074218));
#26593=CARTESIAN_POINT('Ctrl Pts',(-0.412633125322945,-1.,1.8380895347617));
#26594=CARTESIAN_POINT('Ctrl Pts',(-0.412633125322945,1.,1.8380895347617));
#26595=CARTESIAN_POINT('Ctrl Pts',(-0.410641256301276,-1.,1.83100408895047));
#26596=CARTESIAN_POINT('Ctrl Pts',(-0.410641256301276,1.,1.83100408895047));
#26597=CARTESIAN_POINT('Ctrl Pts',(-0.408428948106227,-1.,1.82247022677562));
#26598=CARTESIAN_POINT('Ctrl Pts',(-0.408428948106227,1.,1.82247022677562));
#26599=CARTESIAN_POINT('Ctrl Pts',(-0.405933518407175,-1.,1.81223801812013));
#26600=CARTESIAN_POINT('Ctrl Pts',(-0.405933518407175,1.,1.81223801812013));
#26601=CARTESIAN_POINT('Ctrl Pts',(-0.403107976163396,-1.,1.80012077173238));
#26602=CARTESIAN_POINT('Ctrl Pts',(-0.403107976163396,1.,1.80012077173238));
#26603=CARTESIAN_POINT('Ctrl Pts',(-0.399919403774155,-1.,1.78598826343754));
#26604=CARTESIAN_POINT('Ctrl Pts',(-0.399919403774155,1.,1.78598826343754));
#26605=CARTESIAN_POINT('Ctrl Pts',(-0.396346196110688,-1.,1.76975560043442));
#26606=CARTESIAN_POINT('Ctrl Pts',(-0.396346196110688,1.,1.76975560043442));
#26607=CARTESIAN_POINT('Ctrl Pts',(-0.392375812285395,-1.,1.75137405310193));
#26608=CARTESIAN_POINT('Ctrl Pts',(-0.392375812285395,1.,1.75137405310193));
#26609=CARTESIAN_POINT('Ctrl Pts',(-0.388877023502615,-1.,1.73493170972829));
#26610=CARTESIAN_POINT('Ctrl Pts',(-0.388877023502615,1.,1.73493170972829));
#26611=CARTESIAN_POINT('Ctrl Pts',(-0.386070790323281,-1.,1.72162022244582));
#26612=CARTESIAN_POINT('Ctrl Pts',(-0.386070790323281,1.,1.72162022244582));
#26613=CARTESIAN_POINT('Ctrl Pts',(-0.384119047314215,-1.,1.71231062891398));
#26614=CARTESIAN_POINT('Ctrl Pts',(-0.384119047314215,1.,1.71231062891398));
#26615=CARTESIAN_POINT('Ctrl Pts',(-0.383122945602004,-1.,1.7075470150345));
#26616=CARTESIAN_POINT('Ctrl Pts',(-0.383122945602004,1.,1.7075470150345));
#26617=CARTESIAN_POINT('',(-0.61342227326009,1.,2.11275013067528));
#26618=CARTESIAN_POINT('Ctrl Pts',(-0.61342227326009,1.,2.11275013067528));
#26619=CARTESIAN_POINT('Ctrl Pts',(-0.61246736556225,1.,2.11187554260142));
#26620=CARTESIAN_POINT('Ctrl Pts',(-0.610560911691113,1.,2.11012443807661));
#26621=CARTESIAN_POINT('Ctrl Pts',(-0.607711315456826,1.,2.10749199615859));
#26622=CARTESIAN_POINT('Ctrl Pts',(-0.603932030738212,1.,2.10397049887709));
#26623=CARTESIAN_POINT('Ctrl Pts',(-0.599241616422144,1.,2.09954930865331));
#26624=CARTESIAN_POINT('Ctrl Pts',(-0.594585006052824,1.,2.09510876220501));
#26625=CARTESIAN_POINT('Ctrl Pts',(-0.589962365403189,1.,2.09064881812053));
#26626=CARTESIAN_POINT('Ctrl Pts',(-0.585373918990895,1.,2.086169437277));
#26627=CARTESIAN_POINT('Ctrl Pts',(-0.580819952107257,1.,2.08167059018138));
#26628=CARTESIAN_POINT('Ctrl Pts',(-0.576300797416275,1.,2.07715226767361));
#26629=CARTESIAN_POINT('Ctrl Pts',(-0.571816823242411,1.,2.07261449292757));
#26630=CARTESIAN_POINT('Ctrl Pts',(-0.567368421181229,1.,2.06805732997383));
#26631=CARTESIAN_POINT('Ctrl Pts',(-0.562955993082574,1.,2.06348090160697));
#26632=CARTESIAN_POINT('Ctrl Pts',(-0.558579940185467,1.,2.05888537756571));
#26633=CARTESIAN_POINT('Ctrl Pts',(-0.55424065746411,1.,2.05427091604482));
#26634=CARTESIAN_POINT('Ctrl Pts',(-0.549938525150342,1.,2.04963761077974));
#26635=CARTESIAN_POINT('Ctrl Pts',(-0.545673903817348,1.,2.0449854471456));
#26636=CARTESIAN_POINT('Ctrl Pts',(-0.54144712061552,1.,2.0403142269048));
#26637=CARTESIAN_POINT('Ctrl Pts',(-0.537258489833134,1.,2.03562362953993));
#26638=CARTESIAN_POINT('Ctrl Pts',(-0.533108355132905,1.,2.03091336214401));
#26639=CARTESIAN_POINT('Ctrl Pts',(-0.528997127241911,1.,2.02618329083289));
#26640=CARTESIAN_POINT('Ctrl Pts',(-0.524925318333518,1.,2.02143356304712));
#26641=CARTESIAN_POINT('Ctrl Pts',(-0.520893590399428,1.,2.01666477917305));
#26642=CARTESIAN_POINT('Ctrl Pts',(-0.516902681728733,1.,2.01187773939257));
#26643=CARTESIAN_POINT('Ctrl Pts',(-0.512953306961814,1.,2.00707309946955));
#26644=CARTESIAN_POINT('Ctrl Pts',(-0.509046069886152,1.,2.00225107134733));
#26645=CARTESIAN_POINT('Ctrl Pts',(-0.505181361323011,1.,1.99741107463567));
#26646=CARTESIAN_POINT('Ctrl Pts',(-0.501359287727129,1.,1.9925514912615));
#26647=CARTESIAN_POINT('Ctrl Pts',(-0.497579909545564,1.,1.98767044752929));
#26648=CARTESIAN_POINT('Ctrl Pts',(-0.493843476541492,1.,1.9827665876182));
#26649=CARTESIAN_POINT('Ctrl Pts',(-0.490150627860955,1.,1.97783973019229));
#26650=CARTESIAN_POINT('Ctrl Pts',(-0.486502692907661,1.,1.97289186263272));
#26651=CARTESIAN_POINT('Ctrl Pts',(-0.482901662120687,1.,1.96792703422358));
#26652=CARTESIAN_POINT('Ctrl Pts',(-0.479349583074846,1.,1.96294933055938));
#26653=CARTESIAN_POINT('Ctrl Pts',(-0.475848034683172,1.,1.95796111148175));
#26654=CARTESIAN_POINT('Ctrl Pts',(-0.47239767226408,1.,1.95296148278136));
#26655=CARTESIAN_POINT('Ctrl Pts',(-0.468997482913158,1.,1.94794381136524));
#26656=CARTESIAN_POINT('Ctrl Pts',(-0.465645462026065,1.,1.94289794196205));
#26657=CARTESIAN_POINT('Ctrl Pts',(-0.462340031009087,1.,1.93781486640834));
#26658=CARTESIAN_POINT('Ctrl Pts',(-0.459081234547931,1.,1.93269066517936));
#26659=CARTESIAN_POINT('Ctrl Pts',(-0.455872005174335,1.,1.92753067150461));
#26660=CARTESIAN_POINT('Ctrl Pts',(-0.452719478359356,1.,1.9223538064847));
#26661=CARTESIAN_POINT('Ctrl Pts',(-0.449632260106572,1.,1.91718342555717));
#26662=CARTESIAN_POINT('Ctrl Pts',(-0.446617343485651,1.,1.91203699981095));
#26663=CARTESIAN_POINT('Ctrl Pts',(-0.44367755684917,1.,1.90691756144906));
#26664=CARTESIAN_POINT('Ctrl Pts',(-0.440807833704161,1.,1.90180124389137));
#26665=CARTESIAN_POINT('Ctrl Pts',(-0.437995003948443,1.,1.89663648956549));
#26666=CARTESIAN_POINT('Ctrl Pts',(-0.43522566096358,1.,1.89136993975585));
#26667=CARTESIAN_POINT('Ctrl Pts',(-0.432493038548833,1.,1.88596913666828));
#26668=CARTESIAN_POINT('Ctrl Pts',(-0.429803062482217,1.,1.88044229001778));
#26669=CARTESIAN_POINT('Ctrl Pts',(-0.427183828518743,1.,1.87486989291333));
#26670=CARTESIAN_POINT('Ctrl Pts',(-0.424678177290876,1.,1.8693780394412));
#26671=CARTESIAN_POINT('Ctrl Pts',(-0.422327307417885,1.,1.86408083333863));
#26672=CARTESIAN_POINT('Ctrl Pts',(-0.420157287975583,1.,1.8590328109667));
#26673=CARTESIAN_POINT('Ctrl Pts',(-0.418164129144045,1.,1.8541763285645));
#26674=CARTESIAN_POINT('Ctrl Pts',(-0.416300022039885,1.,1.84929312930314));
#26675=CARTESIAN_POINT('Ctrl Pts',(-0.414487438255542,1.,1.84405757074218));
#26676=CARTESIAN_POINT('Ctrl Pts',(-0.412633125322945,1.,1.8380895347617));
#26677=CARTESIAN_POINT('Ctrl Pts',(-0.410641256301276,1.,1.83100408895047));
#26678=CARTESIAN_POINT('Ctrl Pts',(-0.408428948106227,1.,1.82247022677562));
#26679=CARTESIAN_POINT('Ctrl Pts',(-0.405933518407175,1.,1.81223801812013));
#26680=CARTESIAN_POINT('Ctrl Pts',(-0.403107976163396,1.,1.80012077173238));
#26681=CARTESIAN_POINT('Ctrl Pts',(-0.399919403774155,1.,1.78598826343754));
#26682=CARTESIAN_POINT('Ctrl Pts',(-0.396346196110688,1.,1.76975560043442));
#26683=CARTESIAN_POINT('Ctrl Pts',(-0.392375812285395,1.,1.75137405310193));
#26684=CARTESIAN_POINT('Ctrl Pts',(-0.388877023502615,1.,1.73493170972829));
#26685=CARTESIAN_POINT('Ctrl Pts',(-0.386070790323281,1.,1.72162022244582));
#26686=CARTESIAN_POINT('Ctrl Pts',(-0.384119047314215,1.,1.71231062891398));
#26687=CARTESIAN_POINT('Ctrl Pts',(-0.383122945602004,1.,1.7075470150345));
#26688=CARTESIAN_POINT('',(-0.61342227326009,0.,2.11275013067528));
#26689=CARTESIAN_POINT('Origin',(-0.745574324794401,0.,2.0698113262342));
#26690=CARTESIAN_POINT('',(-0.745574324794401,1.,2.0698113262342));
#26691=CARTESIAN_POINT('',(-0.61342227326009,1.,2.11275013067528));
#26692=CARTESIAN_POINT('',(-0.745574324794401,0.,2.0698113262342));
#26693=CARTESIAN_POINT('Ctrl Pts',(-0.693717979106306,-1.,1.60662857109684));
#26694=CARTESIAN_POINT('Ctrl Pts',(-0.693717979106306,1.,1.60662857109684));
#26695=CARTESIAN_POINT('Ctrl Pts',(-0.695712097881194,-1.,1.61106790958151));
#26696=CARTESIAN_POINT('Ctrl Pts',(-0.695712097881194,1.,1.61106790958151));
#26697=CARTESIAN_POINT('Ctrl Pts',(-0.699605146405088,-1.,1.61974673472612));
#26698=CARTESIAN_POINT('Ctrl Pts',(-0.699605146405088,1.,1.61974673472612));
#26699=CARTESIAN_POINT('Ctrl Pts',(-0.705159151988319,-1.,1.63216541664676));
#26700=CARTESIAN_POINT('Ctrl Pts',(-0.705159151988319,1.,1.63216541664676));
#26701=CARTESIAN_POINT('Ctrl Pts',(-0.711993139355394,-1.,1.64752408832016));
#26702=CARTESIAN_POINT('Ctrl Pts',(-0.711993139355394,1.,1.64752408832016));
#26703=CARTESIAN_POINT('Ctrl Pts',(-0.719585433804282,-1.,1.6647288055568));
#26704=CARTESIAN_POINT('Ctrl Pts',(-0.719585433804282,1.,1.6647288055568));
#26705=CARTESIAN_POINT('Ctrl Pts',(-0.726235967997433,-1.,1.67996158455503));
#26706=CARTESIAN_POINT('Ctrl Pts',(-0.726235967997433,1.,1.67996158455503));
#26707=CARTESIAN_POINT('Ctrl Pts',(-0.731963238697195,-1.,1.69326921975743));
#26708=CARTESIAN_POINT('Ctrl Pts',(-0.731963238697195,1.,1.69326921975743));
#26709=CARTESIAN_POINT('Ctrl Pts',(-0.736799665724771,-1.,1.70473309006121));
#26710=CARTESIAN_POINT('Ctrl Pts',(-0.736799665724771,1.,1.70473309006121));
#26711=CARTESIAN_POINT('Ctrl Pts',(-0.740795162032088,-1.,1.71447789751927));
#26712=CARTESIAN_POINT('Ctrl Pts',(-0.740795162032088,1.,1.71447789751927));
#26713=CARTESIAN_POINT('Ctrl Pts',(-0.744021445433764,-1.,1.7226822991693));
#26714=CARTESIAN_POINT('Ctrl Pts',(-0.744021445433764,1.,1.7226822991693));
#26715=CARTESIAN_POINT('Ctrl Pts',(-0.746574710096436,-1.,1.72958533647399));
#26716=CARTESIAN_POINT('Ctrl Pts',(-0.746574710096436,1.,1.72958533647399));
#26717=CARTESIAN_POINT('Ctrl Pts',(-0.748582462954855,-1.,1.73550351679848));
#26718=CARTESIAN_POINT('Ctrl Pts',(-0.748582462954855,1.,1.73550351679848));
#26719=CARTESIAN_POINT('Ctrl Pts',(-0.75019343597954,-1.,1.74080458266705));
#26720=CARTESIAN_POINT('Ctrl Pts',(-0.75019343597954,1.,1.74080458266705));
#26721=CARTESIAN_POINT('Ctrl Pts',(-0.751555614163629,-1.,1.74585086852298));
#26722=CARTESIAN_POINT('Ctrl Pts',(-0.751555614163629,1.,1.74585086852298));
#26723=CARTESIAN_POINT('Ctrl Pts',(-0.752797683531377,-1.,1.75095139468809));
#26724=CARTESIAN_POINT('Ctrl Pts',(-0.752797683531377,1.,1.75095139468809));
#26725=CARTESIAN_POINT('Ctrl Pts',(-0.75400925402848,-1.,1.75631083600175));
#26726=CARTESIAN_POINT('Ctrl Pts',(-0.75400925402848,1.,1.75631083600175));
#26727=CARTESIAN_POINT('Ctrl Pts',(-0.755220979975262,-1.,1.7619781724032));
#26728=CARTESIAN_POINT('Ctrl Pts',(-0.755220979975262,1.,1.7619781724032));
#26729=CARTESIAN_POINT('Ctrl Pts',(-0.756421896028403,-1.,1.76789396003141));
#26730=CARTESIAN_POINT('Ctrl Pts',(-0.756421896028403,1.,1.76789396003141));
#26731=CARTESIAN_POINT('Ctrl Pts',(-0.757578264077238,-1.,1.77394167108342));
#26732=CARTESIAN_POINT('Ctrl Pts',(-0.757578264077238,1.,1.77394167108342));
#26733=CARTESIAN_POINT('Ctrl Pts',(-0.75865062667738,-1.,1.77999411220912));
#26734=CARTESIAN_POINT('Ctrl Pts',(-0.75865062667738,1.,1.77999411220912));
#26735=CARTESIAN_POINT('Ctrl Pts',(-0.759614401109868,-1.,1.78596964884526));
#26736=CARTESIAN_POINT('Ctrl Pts',(-0.759614401109868,1.,1.78596964884526));
#26737=CARTESIAN_POINT('Ctrl Pts',(-0.760469555880425,-1.,1.79185815610802));
#26738=CARTESIAN_POINT('Ctrl Pts',(-0.760469555880425,1.,1.79185815610802));
#26739=CARTESIAN_POINT('Ctrl Pts',(-0.761229695230359,-1.,1.79768986997735));
#26740=CARTESIAN_POINT('Ctrl Pts',(-0.761229695230359,1.,1.79768986997735));
#26741=CARTESIAN_POINT('Ctrl Pts',(-0.761915336443516,-1.,1.80351583877334));
#26742=CARTESIAN_POINT('Ctrl Pts',(-0.761915336443516,1.,1.80351583877334));
#26743=CARTESIAN_POINT('Ctrl Pts',(-0.762546129464036,-1.,1.80938551463989));
#26744=CARTESIAN_POINT('Ctrl Pts',(-0.762546129464036,1.,1.80938551463989));
#26745=CARTESIAN_POINT('Ctrl Pts',(-0.763132003836783,-1.,1.81532118405566));
#26746=CARTESIAN_POINT('Ctrl Pts',(-0.763132003836783,1.,1.81532118405566));
#26747=CARTESIAN_POINT('Ctrl Pts',(-0.763673465462854,-1.,1.82131873145297));
#26748=CARTESIAN_POINT('Ctrl Pts',(-0.763673465462854,1.,1.82131873145297));
#26749=CARTESIAN_POINT('Ctrl Pts',(-0.764165902606055,-1.,1.8273599120008));
#26750=CARTESIAN_POINT('Ctrl Pts',(-0.764165902606055,1.,1.8273599120008));
#26751=CARTESIAN_POINT('Ctrl Pts',(-0.764602549687845,-1.,1.8334207722714));
#26752=CARTESIAN_POINT('Ctrl Pts',(-0.764602549687845,1.,1.8334207722714));
#26753=CARTESIAN_POINT('Ctrl Pts',(-0.764978057881687,-1.,1.83948181064823));
#26754=CARTESIAN_POINT('Ctrl Pts',(-0.764978057881687,1.,1.83948181064823));
#26755=CARTESIAN_POINT('Ctrl Pts',(-0.765291664861971,-1.,1.8455369887591));
#26756=CARTESIAN_POINT('Ctrl Pts',(-0.765291664861971,1.,1.8455369887591));
#26757=CARTESIAN_POINT('Ctrl Pts',(-0.765545710619023,-1.,1.85158945130054));
#26758=CARTESIAN_POINT('Ctrl Pts',(-0.765545710619023,1.,1.85158945130054));
#26759=CARTESIAN_POINT('Ctrl Pts',(-0.765744212909305,-1.,1.85764741390391));
#26760=CARTESIAN_POINT('Ctrl Pts',(-0.765744212909305,1.,1.85764741390391));
#26761=CARTESIAN_POINT('Ctrl Pts',(-0.765891519092557,-1.,1.86372027063314));
#26762=CARTESIAN_POINT('Ctrl Pts',(-0.765891519092557,1.,1.86372027063314));
#26763=CARTESIAN_POINT('Ctrl Pts',(-0.765990708546111,-1.,1.86981398314345));
#26764=CARTESIAN_POINT('Ctrl Pts',(-0.765990708546111,1.,1.86981398314345));
#26765=CARTESIAN_POINT('Ctrl Pts',(-0.766042837036759,-1.,1.87592888967886));
#26766=CARTESIAN_POINT('Ctrl Pts',(-0.766042837036759,1.,1.87592888967886));
#26767=CARTESIAN_POINT('Ctrl Pts',(-0.766047794851869,-1.,1.88206215302561));
#26768=CARTESIAN_POINT('Ctrl Pts',(-0.766047794851869,1.,1.88206215302561));
#26769=CARTESIAN_POINT('Ctrl Pts',(-0.76600483706209,-1.,1.88820926433409));
#26770=CARTESIAN_POINT('Ctrl Pts',(-0.76600483706209,1.,1.88820926433409));
#26771=CARTESIAN_POINT('Ctrl Pts',(-0.765913193856979,-1.,1.89436577771389));
#26772=CARTESIAN_POINT('Ctrl Pts',(-0.765913193856979,1.,1.89436577771389));
#26773=CARTESIAN_POINT('Ctrl Pts',(-0.765772772593395,-1.,1.90052930393599));
#26774=CARTESIAN_POINT('Ctrl Pts',(-0.765772772593395,1.,1.90052930393599));
#26775=CARTESIAN_POINT('Ctrl Pts',(-0.765584196937936,-1.,1.90669961402362));
#26776=CARTESIAN_POINT('Ctrl Pts',(-0.765584196937936,1.,1.90669961402362));
#26777=CARTESIAN_POINT('Ctrl Pts',(-0.765348465884739,-1.,1.91287765805174));
#26778=CARTESIAN_POINT('Ctrl Pts',(-0.765348465884739,1.,1.91287765805174));
#26779=CARTESIAN_POINT('Ctrl Pts',(-0.765066729667095,-1.,1.91906491634197));
#26780=CARTESIAN_POINT('Ctrl Pts',(-0.765066729667095,1.,1.91906491634197));
#26781=CARTESIAN_POINT('Ctrl Pts',(-0.764740025488189,-1.,1.92526263537041));
#26782=CARTESIAN_POINT('Ctrl Pts',(-0.764740025488189,1.,1.92526263537041));
#26783=CARTESIAN_POINT('Ctrl Pts',(-0.764369010673889,-1.,1.93147105496367));
#26784=CARTESIAN_POINT('Ctrl Pts',(-0.764369010673889,1.,1.93147105496367));
#26785=CARTESIAN_POINT('Ctrl Pts',(-0.763954049121393,-1.,1.93768964875867));
#26786=CARTESIAN_POINT('Ctrl Pts',(-0.763954049121393,1.,1.93768964875867));
#26787=CARTESIAN_POINT('Ctrl Pts',(-0.76349533353858,-1.,1.94391746617626));
#26788=CARTESIAN_POINT('Ctrl Pts',(-0.76349533353858,1.,1.94391746617626));
#26789=CARTESIAN_POINT('Ctrl Pts',(-0.762992990878774,-1.,1.95015342590025));
#26790=CARTESIAN_POINT('Ctrl Pts',(-0.762992990878774,1.,1.95015342590025));
#26791=CARTESIAN_POINT('Ctrl Pts',(-0.762447203806263,-1.,1.95639665309893));
#26792=CARTESIAN_POINT('Ctrl Pts',(-0.762447203806263,1.,1.95639665309893));
#26793=CARTESIAN_POINT('Ctrl Pts',(-0.761858300014575,-1.,1.96264672744229));
#26794=CARTESIAN_POINT('Ctrl Pts',(-0.761858300014575,1.,1.96264672744229));
#26795=CARTESIAN_POINT('Ctrl Pts',(-0.761226690483986,-1.,1.96890351582545));
#26796=CARTESIAN_POINT('Ctrl Pts',(-0.761226690483986,1.,1.96890351582545));
#26797=CARTESIAN_POINT('Ctrl Pts',(-0.760552825409855,-1.,1.97516705321521));
#26798=CARTESIAN_POINT('Ctrl Pts',(-0.760552825409855,1.,1.97516705321521));
#26799=CARTESIAN_POINT('Ctrl Pts',(-0.759837147452135,-1.,1.98143741418156));
#26800=CARTESIAN_POINT('Ctrl Pts',(-0.759837147452135,1.,1.98143741418156));
#26801=CARTESIAN_POINT('Ctrl Pts',(-0.759080037802243,-1.,1.98771456680806));
#26802=CARTESIAN_POINT('Ctrl Pts',(-0.759080037802243,1.,1.98771456680806));
#26803=CARTESIAN_POINT('Ctrl Pts',(-0.758281796766377,-1.,1.9939983109871));
#26804=CARTESIAN_POINT('Ctrl Pts',(-0.758281796766377,1.,1.9939983109871));
#26805=CARTESIAN_POINT('Ctrl Pts',(-0.757442676862341,-1.,2.00028834739072));
#26806=CARTESIAN_POINT('Ctrl Pts',(-0.757442676862341,1.,2.00028834739072));
#26807=CARTESIAN_POINT('Ctrl Pts',(-0.756562904646496,-1.,2.00658431587682));
#26808=CARTESIAN_POINT('Ctrl Pts',(-0.756562904646496,1.,2.00658431587682));
#26809=CARTESIAN_POINT('Ctrl Pts',(-0.7556427049581,-1.,2.01288584328149));
#26810=CARTESIAN_POINT('Ctrl Pts',(-0.7556427049581,1.,2.01288584328149));
#26811=CARTESIAN_POINT('Ctrl Pts',(-0.75468233072352,-1.,2.01919259406003));
#26812=CARTESIAN_POINT('Ctrl Pts',(-0.75468233072352,1.,2.01919259406003));
#26813=CARTESIAN_POINT('Ctrl Pts',(-0.753682061113766,-1.,2.02550428623587));
#26814=CARTESIAN_POINT('Ctrl Pts',(-0.753682061113766,1.,2.02550428623587));
#26815=CARTESIAN_POINT('Ctrl Pts',(-0.752642180488104,-1.,2.03182068456467));
#26816=CARTESIAN_POINT('Ctrl Pts',(-0.752642180488104,1.,2.03182068456467));
#26817=CARTESIAN_POINT('Ctrl Pts',(-0.751562963361384,-1.,2.03814160092173));
#26818=CARTESIAN_POINT('Ctrl Pts',(-0.751562963361384,1.,2.03814160092173));
#26819=CARTESIAN_POINT('Ctrl Pts',(-0.750444657874758,-1.,2.04446689147754));
#26820=CARTESIAN_POINT('Ctrl Pts',(-0.750444657874758,1.,2.04446689147754));
#26821=CARTESIAN_POINT('Ctrl Pts',(-0.749287468663053,-1.,2.05079645591606));
#26822=CARTESIAN_POINT('Ctrl Pts',(-0.749287468663053,1.,2.05079645591606));
#26823=CARTESIAN_POINT('Ctrl Pts',(-0.748091554181101,-1.,2.05713023030263));
#26824=CARTESIAN_POINT('Ctrl Pts',(-0.748091554181101,1.,2.05713023030263));
#26825=CARTESIAN_POINT('Ctrl Pts',(-0.747103932785504,-1.,2.06220058927162));
#26826=CARTESIAN_POINT('Ctrl Pts',(-0.747103932785504,1.,2.06220058927162));
#26827=CARTESIAN_POINT('Ctrl Pts',(-0.746345871542696,-1.,2.06600523016401));
#26828=CARTESIAN_POINT('Ctrl Pts',(-0.746345871542696,1.,2.06600523016401));
#26829=CARTESIAN_POINT('Ctrl Pts',(-0.74583279137781,-1.,2.06854248895575));
#26830=CARTESIAN_POINT('Ctrl Pts',(-0.74583279137781,1.,2.06854248895575));
#26831=CARTESIAN_POINT('Ctrl Pts',(-0.745574324794401,-1.,2.0698113262342));
#26832=CARTESIAN_POINT('Ctrl Pts',(-0.745574324794401,1.,2.0698113262342));
#26833=CARTESIAN_POINT('',(-0.693717979106306,1.,1.60662857109684));
#26834=CARTESIAN_POINT('Ctrl Pts',(-0.693717979106306,1.,1.60662857109684));
#26835=CARTESIAN_POINT('Ctrl Pts',(-0.695712097881194,1.,1.61106790958151));
#26836=CARTESIAN_POINT('Ctrl Pts',(-0.699605146405088,1.,1.61974673472612));
#26837=CARTESIAN_POINT('Ctrl Pts',(-0.705159151988319,1.,1.63216541664676));
#26838=CARTESIAN_POINT('Ctrl Pts',(-0.711993139355394,1.,1.64752408832016));
#26839=CARTESIAN_POINT('Ctrl Pts',(-0.719585433804282,1.,1.6647288055568));
#26840=CARTESIAN_POINT('Ctrl Pts',(-0.726235967997433,1.,1.67996158455503));
#26841=CARTESIAN_POINT('Ctrl Pts',(-0.731963238697195,1.,1.69326921975743));
#26842=CARTESIAN_POINT('Ctrl Pts',(-0.736799665724771,1.,1.70473309006121));
#26843=CARTESIAN_POINT('Ctrl Pts',(-0.740795162032088,1.,1.71447789751927));
#26844=CARTESIAN_POINT('Ctrl Pts',(-0.744021445433764,1.,1.7226822991693));
#26845=CARTESIAN_POINT('Ctrl Pts',(-0.746574710096436,1.,1.72958533647399));
#26846=CARTESIAN_POINT('Ctrl Pts',(-0.748582462954855,1.,1.73550351679848));
#26847=CARTESIAN_POINT('Ctrl Pts',(-0.75019343597954,1.,1.74080458266705));
#26848=CARTESIAN_POINT('Ctrl Pts',(-0.751555614163629,1.,1.74585086852298));
#26849=CARTESIAN_POINT('Ctrl Pts',(-0.752797683531377,1.,1.75095139468809));
#26850=CARTESIAN_POINT('Ctrl Pts',(-0.75400925402848,1.,1.75631083600175));
#26851=CARTESIAN_POINT('Ctrl Pts',(-0.755220979975262,1.,1.7619781724032));
#26852=CARTESIAN_POINT('Ctrl Pts',(-0.756421896028403,1.,1.76789396003141));
#26853=CARTESIAN_POINT('Ctrl Pts',(-0.757578264077238,1.,1.77394167108342));
#26854=CARTESIAN_POINT('Ctrl Pts',(-0.75865062667738,1.,1.77999411220912));
#26855=CARTESIAN_POINT('Ctrl Pts',(-0.759614401109868,1.,1.78596964884526));
#26856=CARTESIAN_POINT('Ctrl Pts',(-0.760469555880425,1.,1.79185815610802));
#26857=CARTESIAN_POINT('Ctrl Pts',(-0.761229695230359,1.,1.79768986997735));
#26858=CARTESIAN_POINT('Ctrl Pts',(-0.761915336443516,1.,1.80351583877334));
#26859=CARTESIAN_POINT('Ctrl Pts',(-0.762546129464036,1.,1.80938551463989));
#26860=CARTESIAN_POINT('Ctrl Pts',(-0.763132003836783,1.,1.81532118405566));
#26861=CARTESIAN_POINT('Ctrl Pts',(-0.763673465462854,1.,1.82131873145297));
#26862=CARTESIAN_POINT('Ctrl Pts',(-0.764165902606055,1.,1.8273599120008));
#26863=CARTESIAN_POINT('Ctrl Pts',(-0.764602549687845,1.,1.8334207722714));
#26864=CARTESIAN_POINT('Ctrl Pts',(-0.764978057881687,1.,1.83948181064823));
#26865=CARTESIAN_POINT('Ctrl Pts',(-0.765291664861971,1.,1.8455369887591));
#26866=CARTESIAN_POINT('Ctrl Pts',(-0.765545710619023,1.,1.85158945130054));
#26867=CARTESIAN_POINT('Ctrl Pts',(-0.765744212909305,1.,1.85764741390391));
#26868=CARTESIAN_POINT('Ctrl Pts',(-0.765891519092557,1.,1.86372027063314));
#26869=CARTESIAN_POINT('Ctrl Pts',(-0.765990708546111,1.,1.86981398314345));
#26870=CARTESIAN_POINT('Ctrl Pts',(-0.766042837036759,1.,1.87592888967886));
#26871=CARTESIAN_POINT('Ctrl Pts',(-0.766047794851869,1.,1.88206215302561));
#26872=CARTESIAN_POINT('Ctrl Pts',(-0.76600483706209,1.,1.88820926433409));
#26873=CARTESIAN_POINT('Ctrl Pts',(-0.765913193856979,1.,1.89436577771389));
#26874=CARTESIAN_POINT('Ctrl Pts',(-0.765772772593395,1.,1.90052930393599));
#26875=CARTESIAN_POINT('Ctrl Pts',(-0.765584196937936,1.,1.90669961402362));
#26876=CARTESIAN_POINT('Ctrl Pts',(-0.765348465884739,1.,1.91287765805174));
#26877=CARTESIAN_POINT('Ctrl Pts',(-0.765066729667095,1.,1.91906491634197));
#26878=CARTESIAN_POINT('Ctrl Pts',(-0.764740025488189,1.,1.92526263537041));
#26879=CARTESIAN_POINT('Ctrl Pts',(-0.764369010673889,1.,1.93147105496367));
#26880=CARTESIAN_POINT('Ctrl Pts',(-0.763954049121393,1.,1.93768964875867));
#26881=CARTESIAN_POINT('Ctrl Pts',(-0.76349533353858,1.,1.94391746617626));
#26882=CARTESIAN_POINT('Ctrl Pts',(-0.762992990878774,1.,1.95015342590025));
#26883=CARTESIAN_POINT('Ctrl Pts',(-0.762447203806263,1.,1.95639665309893));
#26884=CARTESIAN_POINT('Ctrl Pts',(-0.761858300014575,1.,1.96264672744229));
#26885=CARTESIAN_POINT('Ctrl Pts',(-0.761226690483986,1.,1.96890351582545));
#26886=CARTESIAN_POINT('Ctrl Pts',(-0.760552825409855,1.,1.97516705321521));
#26887=CARTESIAN_POINT('Ctrl Pts',(-0.759837147452135,1.,1.98143741418156));
#26888=CARTESIAN_POINT('Ctrl Pts',(-0.759080037802243,1.,1.98771456680806));
#26889=CARTESIAN_POINT('Ctrl Pts',(-0.758281796766377,1.,1.9939983109871));
#26890=CARTESIAN_POINT('Ctrl Pts',(-0.757442676862341,1.,2.00028834739072));
#26891=CARTESIAN_POINT('Ctrl Pts',(-0.756562904646496,1.,2.00658431587682));
#26892=CARTESIAN_POINT('Ctrl Pts',(-0.7556427049581,1.,2.01288584328149));
#26893=CARTESIAN_POINT('Ctrl Pts',(-0.75468233072352,1.,2.01919259406003));
#26894=CARTESIAN_POINT('Ctrl Pts',(-0.753682061113766,1.,2.02550428623587));
#26895=CARTESIAN_POINT('Ctrl Pts',(-0.752642180488104,1.,2.03182068456467));
#26896=CARTESIAN_POINT('Ctrl Pts',(-0.751562963361384,1.,2.03814160092173));
#26897=CARTESIAN_POINT('Ctrl Pts',(-0.750444657874758,1.,2.04446689147754));
#26898=CARTESIAN_POINT('Ctrl Pts',(-0.749287468663053,1.,2.05079645591606));
#26899=CARTESIAN_POINT('Ctrl Pts',(-0.748091554181101,1.,2.05713023030263));
#26900=CARTESIAN_POINT('Ctrl Pts',(-0.747103932785504,1.,2.06220058927162));
#26901=CARTESIAN_POINT('Ctrl Pts',(-0.746345871542696,1.,2.06600523016401));
#26902=CARTESIAN_POINT('Ctrl Pts',(-0.74583279137781,1.,2.06854248895575));
#26903=CARTESIAN_POINT('Ctrl Pts',(-0.745574324794401,1.,2.0698113262342));
#26904=CARTESIAN_POINT('',(-0.693717979106306,0.,1.60662857109684));
#26905=CARTESIAN_POINT('Origin',(0.,0.,0.));
#26906=CARTESIAN_POINT('',(-0.892032620296855,1.,1.5055822144029));
#26907=CARTESIAN_POINT('Origin',(0.,1.,0.));
#26908=CARTESIAN_POINT('',(-0.892032620296855,0.,1.5055822144029));
#26909=CARTESIAN_POINT('Ctrl Pts',(-1.23627494547115,-1.,1.81978687191668));
#26910=CARTESIAN_POINT('Ctrl Pts',(-1.23627494547115,1.,1.81978687191668));
#26911=CARTESIAN_POINT('Ctrl Pts',(-1.23509651170476,-1.,1.81925017193666));
#26912=CARTESIAN_POINT('Ctrl Pts',(-1.23509651170476,1.,1.81925017193666));
#26913=CARTESIAN_POINT('Ctrl Pts',(-1.2327422452705,-1.,1.81817389921279));
#26914=CARTESIAN_POINT('Ctrl Pts',(-1.2327422452705,1.,1.81817389921279));
#26915=CARTESIAN_POINT('Ctrl Pts',(-1.2292186489137,-1.,1.8165508718364));
#26916=CARTESIAN_POINT('Ctrl Pts',(-1.2292186489137,1.,1.8165508718364));
#26917=CARTESIAN_POINT('Ctrl Pts',(-1.2245361330495,-1.,1.81436959210434));
#26918=CARTESIAN_POINT('Ctrl Pts',(-1.2245361330495,1.,1.81436959210434));
#26919=CARTESIAN_POINT('Ctrl Pts',(-1.21870906103557,-1.,1.81161420806656));
#26920=CARTESIAN_POINT('Ctrl Pts',(-1.21870906103557,1.,1.81161420806656));
#26921=CARTESIAN_POINT('Ctrl Pts',(-1.21290815708314,-1.,1.80882996917129));
#26922=CARTESIAN_POINT('Ctrl Pts',(-1.21290815708314,1.,1.80882996917129));
#26923=CARTESIAN_POINT('Ctrl Pts',(-1.20713356605475,-1.,1.80601678480707));
#26924=CARTESIAN_POINT('Ctrl Pts',(-1.20713356605475,1.,1.80601678480707));
#26925=CARTESIAN_POINT('Ctrl Pts',(-1.20138548938974,-1.,1.80317454838603));
#26926=CARTESIAN_POINT('Ctrl Pts',(-1.20138548938974,1.,1.80317454838603));
#26927=CARTESIAN_POINT('Ctrl Pts',(-1.19566418930242,-1.,1.80030314369879));
#26928=CARTESIAN_POINT('Ctrl Pts',(-1.19566418930242,1.,1.80030314369879));
#26929=CARTESIAN_POINT('Ctrl Pts',(-1.18996997934445,-1.,1.79740245923478));
#26930=CARTESIAN_POINT('Ctrl Pts',(-1.18996997934445,1.,1.79740245923478));
#26931=CARTESIAN_POINT('Ctrl Pts',(-1.18430321697432,-1.,1.79447240321515));
#26932=CARTESIAN_POINT('Ctrl Pts',(-1.18430321697432,1.,1.79447240321515));
#26933=CARTESIAN_POINT('Ctrl Pts',(-1.17866429440809,-1.,1.79151291552689));
#26934=CARTESIAN_POINT('Ctrl Pts',(-1.17866429440809,1.,1.79151291552689));
#26935=CARTESIAN_POINT('Ctrl Pts',(-1.17305363177328,-1.,1.78852398877616));
#26936=CARTESIAN_POINT('Ctrl Pts',(-1.17305363177328,1.,1.78852398877616));
#26937=CARTESIAN_POINT('Ctrl Pts',(-1.16747166312303,-1.,1.78550566040443));
#26938=CARTESIAN_POINT('Ctrl Pts',(-1.16747166312303,1.,1.78550566040443));
#26939=CARTESIAN_POINT('Ctrl Pts',(-1.16191881298499,-1.,1.78245795881009));
#26940=CARTESIAN_POINT('Ctrl Pts',(-1.16191881298499,1.,1.78245795881009));
#26941=CARTESIAN_POINT('Ctrl Pts',(-1.15639547194698,-1.,1.77938085564275));
#26942=CARTESIAN_POINT('Ctrl Pts',(-1.15639547194698,1.,1.77938085564275));
#26943=CARTESIAN_POINT('Ctrl Pts',(-1.15090197841515,-1.,1.7762742255701));
#26944=CARTESIAN_POINT('Ctrl Pts',(-1.15090197841515,1.,1.7762742255701));
#26945=CARTESIAN_POINT('Ctrl Pts',(-1.1454385822692,-1.,1.77313777896194));
#26946=CARTESIAN_POINT('Ctrl Pts',(-1.1454385822692,1.,1.77313777896194));
#26947=CARTESIAN_POINT('Ctrl Pts',(-1.14000548336975,-1.,1.76997111386769));
#26948=CARTESIAN_POINT('Ctrl Pts',(-1.14000548336975,1.,1.76997111386769));
#26949=CARTESIAN_POINT('Ctrl Pts',(-1.1346029180462,-1.,1.76677384551862));
#26950=CARTESIAN_POINT('Ctrl Pts',(-1.1346029180462,1.,1.76677384551862));
#26951=CARTESIAN_POINT('Ctrl Pts',(-1.12923123555075,-1.,1.7635457196617));
#26952=CARTESIAN_POINT('Ctrl Pts',(-1.12923123555075,1.,1.7635457196617));
#26953=CARTESIAN_POINT('Ctrl Pts',(-1.12389096855086,-1.,1.76028671825096));
#26954=CARTESIAN_POINT('Ctrl Pts',(-1.12389096855086,1.,1.76028671825096));
#26955=CARTESIAN_POINT('Ctrl Pts',(-1.11858293216763,-1.,1.75699720772105));
#26956=CARTESIAN_POINT('Ctrl Pts',(-1.11858293216763,1.,1.75699720772105));
#26957=CARTESIAN_POINT('Ctrl Pts',(-1.11330807582551,-1.,1.7536777209463));
#26958=CARTESIAN_POINT('Ctrl Pts',(-1.11330807582551,1.,1.7536777209463));
#26959=CARTESIAN_POINT('Ctrl Pts',(-1.10806728183007,-1.,1.7503286607592));
#26960=CARTESIAN_POINT('Ctrl Pts',(-1.10806728183007,1.,1.7503286607592));
#26961=CARTESIAN_POINT('Ctrl Pts',(-1.10286118991143,-1.,1.74695004214923));
#26962=CARTESIAN_POINT('Ctrl Pts',(-1.10286118991143,1.,1.74695004214923));
#26963=CARTESIAN_POINT('Ctrl Pts',(-1.09768999241225,-1.,1.74354119236208));
#26964=CARTESIAN_POINT('Ctrl Pts',(-1.09768999241225,1.,1.74354119236208));
#26965=CARTESIAN_POINT('Ctrl Pts',(-1.09255329056493,-1.,1.74010053962247));
#26966=CARTESIAN_POINT('Ctrl Pts',(-1.09255329056493,1.,1.74010053962247));
#26967=CARTESIAN_POINT('Ctrl Pts',(-1.08745056285427,-1.,1.73662628326091));
#26968=CARTESIAN_POINT('Ctrl Pts',(-1.08745056285427,1.,1.73662628326091));
#26969=CARTESIAN_POINT('Ctrl Pts',(-1.08238162784749,-1.,1.73311705663407));
#26970=CARTESIAN_POINT('Ctrl Pts',(-1.08238162784749,1.,1.73311705663407));
#26971=CARTESIAN_POINT('Ctrl Pts',(-1.0773470373727,-1.,1.72957248977424));
#26972=CARTESIAN_POINT('Ctrl Pts',(-1.0773470373727,1.,1.72957248977424));
#26973=CARTESIAN_POINT('Ctrl Pts',(-1.07234866990252,-1.,1.72599406198488));
#26974=CARTESIAN_POINT('Ctrl Pts',(-1.07234866990252,1.,1.72599406198488));
#26975=CARTESIAN_POINT('Ctrl Pts',(-1.06738966975462,-1.,1.72238500928453));
#26976=CARTESIAN_POINT('Ctrl Pts',(-1.06738966975462,1.,1.72238500928453));
#26977=CARTESIAN_POINT('Ctrl Pts',(-1.06247324680647,-1.,1.71874858456904));
#26978=CARTESIAN_POINT('Ctrl Pts',(-1.06247324680647,1.,1.71874858456904));
#26979=CARTESIAN_POINT('Ctrl Pts',(-1.05760163192479,-1.,1.7150865442702));
#26980=CARTESIAN_POINT('Ctrl Pts',(-1.05760163192479,1.,1.7150865442702));
#26981=CARTESIAN_POINT('Ctrl Pts',(-1.05277517202855,-1.,1.71139783543989));
#26982=CARTESIAN_POINT('Ctrl Pts',(-1.05277517202855,1.,1.71139783543989));
#26983=CARTESIAN_POINT('Ctrl Pts',(-1.04799085404995,-1.,1.70767646263649));
#26984=CARTESIAN_POINT('Ctrl Pts',(-1.04799085404995,1.,1.70767646263649));
#26985=CARTESIAN_POINT('Ctrl Pts',(-1.04324363334554,-1.,1.70391338707982));
#26986=CARTESIAN_POINT('Ctrl Pts',(-1.04324363334554,1.,1.70391338707982));
#26987=CARTESIAN_POINT('Ctrl Pts',(-1.03852922490789,-1.,1.70010052930962));
#26988=CARTESIAN_POINT('Ctrl Pts',(-1.03852922490789,1.,1.70010052930962));
#26989=CARTESIAN_POINT('Ctrl Pts',(-1.03384646003588,-1.,1.69623414782771));
#26990=CARTESIAN_POINT('Ctrl Pts',(-1.03384646003588,1.,1.69623414782771));
#26991=CARTESIAN_POINT('Ctrl Pts',(-1.02919977579147,-1.,1.69231840863458));
#26992=CARTESIAN_POINT('Ctrl Pts',(-1.02919977579147,1.,1.69231840863458));
#26993=CARTESIAN_POINT('Ctrl Pts',(-1.02460180535255,-1.,1.68836910178447));
#26994=CARTESIAN_POINT('Ctrl Pts',(-1.02460180535255,1.,1.68836910178447));
#26995=CARTESIAN_POINT('Ctrl Pts',(-1.02006795074201,-1.,1.68440578021706));
#26996=CARTESIAN_POINT('Ctrl Pts',(-1.02006795074201,1.,1.68440578021706));
#26997=CARTESIAN_POINT('Ctrl Pts',(-1.01561026162773,-1.,1.68044289894798));
#26998=CARTESIAN_POINT('Ctrl Pts',(-1.01561026162773,1.,1.68044289894798));
#26999=CARTESIAN_POINT('Ctrl Pts',(-1.01123236493511,-1.,1.67648246776464));
#27000=CARTESIAN_POINT('Ctrl Pts',(-1.01123236493511,1.,1.67648246776464));
#27001=CARTESIAN_POINT('Ctrl Pts',(-1.00692206696414,-1.,1.67250335383293));
#27002=CARTESIAN_POINT('Ctrl Pts',(-1.00692206696414,1.,1.67250335383293));
#27003=CARTESIAN_POINT('Ctrl Pts',(-1.00265091003727,-1.,1.66846059277303));
#27004=CARTESIAN_POINT('Ctrl Pts',(-1.00265091003727,1.,1.66846059277303));
#27005=CARTESIAN_POINT('Ctrl Pts',(-0.998389654952758,-1.,1.66430758030376));
#27006=CARTESIAN_POINT('Ctrl Pts',(-0.998389654952758,1.,1.66430758030376));
#27007=CARTESIAN_POINT('Ctrl Pts',(-0.994121836661306,-1.,1.66001553809947));
#27008=CARTESIAN_POINT('Ctrl Pts',(-0.994121836661306,1.,1.66001553809947));
#27009=CARTESIAN_POINT('Ctrl Pts',(-0.989855627854165,-1.,1.65559044289699));
#27010=CARTESIAN_POINT('Ctrl Pts',(-0.989855627854165,1.,1.65559044289699));
#27011=CARTESIAN_POINT('Ctrl Pts',(-0.985642622920821,-1.,1.65110016612638));
#27012=CARTESIAN_POINT('Ctrl Pts',(-0.985642622920821,1.,1.65110016612638));
#27013=CARTESIAN_POINT('Ctrl Pts',(-0.981562530939489,-1.,1.64665139190656));
#27014=CARTESIAN_POINT('Ctrl Pts',(-0.981562530939489,1.,1.64665139190656));
#27015=CARTESIAN_POINT('Ctrl Pts',(-0.977689794119416,-1.,1.64233990826687));
#27016=CARTESIAN_POINT('Ctrl Pts',(-0.977689794119416,1.,1.64233990826687));
#27017=CARTESIAN_POINT('Ctrl Pts',(-0.974066058287418,-1.,1.63820952658144));
#27018=CARTESIAN_POINT('Ctrl Pts',(-0.974066058287418,1.,1.63820952658144));
#27019=CARTESIAN_POINT('Ctrl Pts',(-0.970669715997509,-1.,1.63420665729798));
#27020=CARTESIAN_POINT('Ctrl Pts',(-0.970669715997509,1.,1.63420665729798));
#27021=CARTESIAN_POINT('Ctrl Pts',(-0.967387853230345,-1.,1.63013849959461));
#27022=CARTESIAN_POINT('Ctrl Pts',(-0.967387853230345,1.,1.63013849959461));
#27023=CARTESIAN_POINT('Ctrl Pts',(-0.964046107040536,-1.,1.62571930670187));
#27024=CARTESIAN_POINT('Ctrl Pts',(-0.964046107040536,1.,1.62571930670187));
#27025=CARTESIAN_POINT('Ctrl Pts',(-0.960438326101729,-1.,1.62061638140221));
#27026=CARTESIAN_POINT('Ctrl Pts',(-0.960438326101729,1.,1.62061638140221));
#27027=CARTESIAN_POINT('Ctrl Pts',(-0.956354422920671,-1.,1.61449324337085));
#27028=CARTESIAN_POINT('Ctrl Pts',(-0.956354422920671,1.,1.61449324337085));
#27029=CARTESIAN_POINT('Ctrl Pts',(-0.951613284356035,-1.,1.60706069896936));
#27030=CARTESIAN_POINT('Ctrl Pts',(-0.951613284356035,1.,1.60706069896936));
#27031=CARTESIAN_POINT('Ctrl Pts',(-0.946078063315257,-1.,1.59810042043673));
#27032=CARTESIAN_POINT('Ctrl Pts',(-0.946078063315257,1.,1.59810042043673));
#27033=CARTESIAN_POINT('Ctrl Pts',(-0.939646377893399,-1.,1.58744937487176));
#27034=CARTESIAN_POINT('Ctrl Pts',(-0.939646377893399,1.,1.58744937487176));
#27035=CARTESIAN_POINT('Ctrl Pts',(-0.932246680108685,-1.,1.57499388382243));
#27036=CARTESIAN_POINT('Ctrl Pts',(-0.932246680108685,1.,1.57499388382243));
#27037=CARTESIAN_POINT('Ctrl Pts',(-0.923832188944341,-1.,1.56065988578893));
#27038=CARTESIAN_POINT('Ctrl Pts',(-0.923832188944341,1.,1.56065988578893));
#27039=CARTESIAN_POINT('Ctrl Pts',(-0.914375919026456,-1.,1.54440491149498));
#27040=CARTESIAN_POINT('Ctrl Pts',(-0.914375919026456,1.,1.54440491149498));
#27041=CARTESIAN_POINT('Ctrl Pts',(-0.905967409625651,-1.,1.52984849887993));
#27042=CARTESIAN_POINT('Ctrl Pts',(-0.905967409625651,1.,1.52984849887993));
#27043=CARTESIAN_POINT('Ctrl Pts',(-0.899185047483511,-1.,1.51805569590094));
#27044=CARTESIAN_POINT('Ctrl Pts',(-0.899185047483511,1.,1.51805569590094));
#27045=CARTESIAN_POINT('Ctrl Pts',(-0.894452006964543,-1.,1.50980486806688));
#27046=CARTESIAN_POINT('Ctrl Pts',(-0.894452006964543,1.,1.50980486806688));
#27047=CARTESIAN_POINT('Ctrl Pts',(-0.892032620296855,-1.,1.5055822144029));
#27048=CARTESIAN_POINT('Ctrl Pts',(-0.892032620296855,1.,1.5055822144029));
#27049=CARTESIAN_POINT('',(-1.23627494547115,1.,1.81978687191668));
#27050=CARTESIAN_POINT('Ctrl Pts',(-1.23627494547115,1.,1.81978687191668));
#27051=CARTESIAN_POINT('Ctrl Pts',(-1.23509651170476,1.,1.81925017193666));
#27052=CARTESIAN_POINT('Ctrl Pts',(-1.2327422452705,1.,1.81817389921279));
#27053=CARTESIAN_POINT('Ctrl Pts',(-1.2292186489137,1.,1.8165508718364));
#27054=CARTESIAN_POINT('Ctrl Pts',(-1.2245361330495,1.,1.81436959210434));
#27055=CARTESIAN_POINT('Ctrl Pts',(-1.21870906103557,1.,1.81161420806656));
#27056=CARTESIAN_POINT('Ctrl Pts',(-1.21290815708314,1.,1.80882996917129));
#27057=CARTESIAN_POINT('Ctrl Pts',(-1.20713356605475,1.,1.80601678480707));
#27058=CARTESIAN_POINT('Ctrl Pts',(-1.20138548938974,1.,1.80317454838603));
#27059=CARTESIAN_POINT('Ctrl Pts',(-1.19566418930242,1.,1.80030314369879));
#27060=CARTESIAN_POINT('Ctrl Pts',(-1.18996997934445,1.,1.79740245923478));
#27061=CARTESIAN_POINT('Ctrl Pts',(-1.18430321697432,1.,1.79447240321515));
#27062=CARTESIAN_POINT('Ctrl Pts',(-1.17866429440809,1.,1.79151291552689));
#27063=CARTESIAN_POINT('Ctrl Pts',(-1.17305363177328,1.,1.78852398877616));
#27064=CARTESIAN_POINT('Ctrl Pts',(-1.16747166312303,1.,1.78550566040443));
#27065=CARTESIAN_POINT('Ctrl Pts',(-1.16191881298499,1.,1.78245795881009));
#27066=CARTESIAN_POINT('Ctrl Pts',(-1.15639547194698,1.,1.77938085564275));
#27067=CARTESIAN_POINT('Ctrl Pts',(-1.15090197841515,1.,1.7762742255701));
#27068=CARTESIAN_POINT('Ctrl Pts',(-1.1454385822692,1.,1.77313777896194));
#27069=CARTESIAN_POINT('Ctrl Pts',(-1.14000548336975,1.,1.76997111386769));
#27070=CARTESIAN_POINT('Ctrl Pts',(-1.1346029180462,1.,1.76677384551862));
#27071=CARTESIAN_POINT('Ctrl Pts',(-1.12923123555075,1.,1.7635457196617));
#27072=CARTESIAN_POINT('Ctrl Pts',(-1.12389096855086,1.,1.76028671825096));
#27073=CARTESIAN_POINT('Ctrl Pts',(-1.11858293216763,1.,1.75699720772105));
#27074=CARTESIAN_POINT('Ctrl Pts',(-1.11330807582551,1.,1.7536777209463));
#27075=CARTESIAN_POINT('Ctrl Pts',(-1.10806728183007,1.,1.7503286607592));
#27076=CARTESIAN_POINT('Ctrl Pts',(-1.10286118991143,1.,1.74695004214923));
#27077=CARTESIAN_POINT('Ctrl Pts',(-1.09768999241225,1.,1.74354119236208));
#27078=CARTESIAN_POINT('Ctrl Pts',(-1.09255329056493,1.,1.74010053962247));
#27079=CARTESIAN_POINT('Ctrl Pts',(-1.08745056285427,1.,1.73662628326091));
#27080=CARTESIAN_POINT('Ctrl Pts',(-1.08238162784749,1.,1.73311705663407));
#27081=CARTESIAN_POINT('Ctrl Pts',(-1.0773470373727,1.,1.72957248977424));
#27082=CARTESIAN_POINT('Ctrl Pts',(-1.07234866990252,1.,1.72599406198488));
#27083=CARTESIAN_POINT('Ctrl Pts',(-1.06738966975462,1.,1.72238500928453));
#27084=CARTESIAN_POINT('Ctrl Pts',(-1.06247324680647,1.,1.71874858456904));
#27085=CARTESIAN_POINT('Ctrl Pts',(-1.05760163192479,1.,1.7150865442702));
#27086=CARTESIAN_POINT('Ctrl Pts',(-1.05277517202855,1.,1.71139783543989));
#27087=CARTESIAN_POINT('Ctrl Pts',(-1.04799085404995,1.,1.70767646263649));
#27088=CARTESIAN_POINT('Ctrl Pts',(-1.04324363334554,1.,1.70391338707982));
#27089=CARTESIAN_POINT('Ctrl Pts',(-1.03852922490789,1.,1.70010052930962));
#27090=CARTESIAN_POINT('Ctrl Pts',(-1.03384646003588,1.,1.69623414782771));
#27091=CARTESIAN_POINT('Ctrl Pts',(-1.02919977579147,1.,1.69231840863458));
#27092=CARTESIAN_POINT('Ctrl Pts',(-1.02460180535255,1.,1.68836910178447));
#27093=CARTESIAN_POINT('Ctrl Pts',(-1.02006795074201,1.,1.68440578021706));
#27094=CARTESIAN_POINT('Ctrl Pts',(-1.01561026162773,1.,1.68044289894798));
#27095=CARTESIAN_POINT('Ctrl Pts',(-1.01123236493511,1.,1.67648246776464));
#27096=CARTESIAN_POINT('Ctrl Pts',(-1.00692206696414,1.,1.67250335383293));
#27097=CARTESIAN_POINT('Ctrl Pts',(-1.00265091003727,1.,1.66846059277303));
#27098=CARTESIAN_POINT('Ctrl Pts',(-0.998389654952758,1.,1.66430758030376));
#27099=CARTESIAN_POINT('Ctrl Pts',(-0.994121836661306,1.,1.66001553809947));
#27100=CARTESIAN_POINT('Ctrl Pts',(-0.989855627854165,1.,1.65559044289699));
#27101=CARTESIAN_POINT('Ctrl Pts',(-0.985642622920821,1.,1.65110016612638));
#27102=CARTESIAN_POINT('Ctrl Pts',(-0.981562530939489,1.,1.64665139190656));
#27103=CARTESIAN_POINT('Ctrl Pts',(-0.977689794119416,1.,1.64233990826687));
#27104=CARTESIAN_POINT('Ctrl Pts',(-0.974066058287418,1.,1.63820952658144));
#27105=CARTESIAN_POINT('Ctrl Pts',(-0.970669715997509,1.,1.63420665729798));
#27106=CARTESIAN_POINT('Ctrl Pts',(-0.967387853230345,1.,1.63013849959461));
#27107=CARTESIAN_POINT('Ctrl Pts',(-0.964046107040536,1.,1.62571930670187));
#27108=CARTESIAN_POINT('Ctrl Pts',(-0.960438326101729,1.,1.62061638140221));
#27109=CARTESIAN_POINT('Ctrl Pts',(-0.956354422920671,1.,1.61449324337085));
#27110=CARTESIAN_POINT('Ctrl Pts',(-0.951613284356035,1.,1.60706069896936));
#27111=CARTESIAN_POINT('Ctrl Pts',(-0.946078063315257,1.,1.59810042043673));
#27112=CARTESIAN_POINT('Ctrl Pts',(-0.939646377893399,1.,1.58744937487176));
#27113=CARTESIAN_POINT('Ctrl Pts',(-0.932246680108685,1.,1.57499388382243));
#27114=CARTESIAN_POINT('Ctrl Pts',(-0.923832188944341,1.,1.56065988578893));
#27115=CARTESIAN_POINT('Ctrl Pts',(-0.914375919026456,1.,1.54440491149498));
#27116=CARTESIAN_POINT('Ctrl Pts',(-0.905967409625651,1.,1.52984849887993));
#27117=CARTESIAN_POINT('Ctrl Pts',(-0.899185047483511,1.,1.51805569590094));
#27118=CARTESIAN_POINT('Ctrl Pts',(-0.894452006964543,1.,1.50980486806688));
#27119=CARTESIAN_POINT('Ctrl Pts',(-0.892032620296855,1.,1.5055822144029));
#27120=CARTESIAN_POINT('',(-1.23627494547115,0.,1.81978687191668));
#27121=CARTESIAN_POINT('Origin',(-1.34869019493419,0.,1.73811241238545));
#27122=CARTESIAN_POINT('',(-1.34869019493419,1.,1.73811241238545));
#27123=CARTESIAN_POINT('',(-1.23627494547115,1.,1.81978687191668));
#27124=CARTESIAN_POINT('',(-1.34869019493419,0.,1.73811241238545));
#27125=CARTESIAN_POINT('Ctrl Pts',(-1.15624053661742,-1.,1.31362392696032));
#27126=CARTESIAN_POINT('Ctrl Pts',(-1.15624053661742,1.,1.31362392696032));
#27127=CARTESIAN_POINT('Ctrl Pts',(-1.15950888730809,-1.,1.31722977216397));
#27128=CARTESIAN_POINT('Ctrl Pts',(-1.15950888730809,1.,1.31722977216397));
#27129=CARTESIAN_POINT('Ctrl Pts',(-1.16589330093588,-1.,1.32428080721772));
#27130=CARTESIAN_POINT('Ctrl Pts',(-1.16589330093588,1.,1.32428080721772));
#27131=CARTESIAN_POINT('Ctrl Pts',(-1.17501305789857,-1.,1.33437539347008));
#27132=CARTESIAN_POINT('Ctrl Pts',(-1.17501305789857,1.,1.33437539347008));
#27133=CARTESIAN_POINT('Ctrl Pts',(-1.18625865667441,-1.,1.34687054001093));
#27134=CARTESIAN_POINT('Ctrl Pts',(-1.18625865667441,1.,1.34687054001093));
#27135=CARTESIAN_POINT('Ctrl Pts',(-1.1987959077932,-1.,1.36088705043885));
#27136=CARTESIAN_POINT('Ctrl Pts',(-1.1987959077932,1.,1.36088705043885));
#27137=CARTESIAN_POINT('Ctrl Pts',(-1.20982812925645,-1.,1.37331915607905));
#27138=CARTESIAN_POINT('Ctrl Pts',(-1.20982812925645,1.,1.37331915607905));
#27139=CARTESIAN_POINT('Ctrl Pts',(-1.21938737280852,-1.,1.38420564527715));
#27140=CARTESIAN_POINT('Ctrl Pts',(-1.21938737280852,1.,1.38420564527715));
#27141=CARTESIAN_POINT('Ctrl Pts',(-1.22752961899387,-1.,1.39361389568796));
#27142=CARTESIAN_POINT('Ctrl Pts',(-1.22752961899387,1.,1.39361389568796));
#27143=CARTESIAN_POINT('Ctrl Pts',(-1.23434087290423,-1.,1.40164708206106));
#27144=CARTESIAN_POINT('Ctrl Pts',(-1.23434087290423,1.,1.40164708206106));
#27145=CARTESIAN_POINT('Ctrl Pts',(-1.23994455029534,-1.,1.40845295531283));
#27146=CARTESIAN_POINT('Ctrl Pts',(-1.23994455029534,1.,1.40845295531283));
#27147=CARTESIAN_POINT('Ctrl Pts',(-1.24450600513056,-1.,1.41422913175179));
#27148=CARTESIAN_POINT('Ctrl Pts',(-1.24450600513056,1.,1.41422913175179));
#27149=CARTESIAN_POINT('Ctrl Pts',(-1.24824430986571,-1.,1.41923722596025));
#27150=CARTESIAN_POINT('Ctrl Pts',(-1.24824430986571,1.,1.41923722596025));
#27151=CARTESIAN_POINT('Ctrl Pts',(-1.2514145557001,-1.,1.42378102115575));
#27152=CARTESIAN_POINT('Ctrl Pts',(-1.2514145557001,1.,1.42378102115575));
#27153=CARTESIAN_POINT('Ctrl Pts',(-1.25426945222639,-1.,1.42815938799387));
#27154=CARTESIAN_POINT('Ctrl Pts',(-1.25426945222639,1.,1.42815938799387));
#27155=CARTESIAN_POINT('Ctrl Pts',(-1.25702687965755,-1.,1.43262645609691));
#27156=CARTESIAN_POINT('Ctrl Pts',(-1.25702687965755,1.,1.43262645609691));
#27157=CARTESIAN_POINT('Ctrl Pts',(-1.25983531012005,-1.,1.43734919180848));
#27158=CARTESIAN_POINT('Ctrl Pts',(-1.25983531012005,1.,1.43734919180848));
#27159=CARTESIAN_POINT('Ctrl Pts',(-1.26273903323859,-1.,1.44236470511303));
#27160=CARTESIAN_POINT('Ctrl Pts',(-1.26273903323859,1.,1.44236470511303));
#27161=CARTESIAN_POINT('Ctrl Pts',(-1.26570925118868,-1.,1.44761985001662));
#27162=CARTESIAN_POINT('Ctrl Pts',(-1.26570925118868,1.,1.44761985001662));
#27163=CARTESIAN_POINT('Ctrl Pts',(-1.2686778680489,-1.,1.45301422764247));
#27164=CARTESIAN_POINT('Ctrl Pts',(-1.2686778680489,1.,1.45301422764247));
#27165=CARTESIAN_POINT('Ctrl Pts',(-1.27156805265289,-1.,1.45843906294697));
#27166=CARTESIAN_POINT('Ctrl Pts',(-1.27156805265289,1.,1.45843906294697));
#27167=CARTESIAN_POINT('Ctrl Pts',(-1.27433119897822,-1.,1.46382431332476));
#27168=CARTESIAN_POINT('Ctrl Pts',(-1.27433119897822,1.,1.46382431332476));
#27169=CARTESIAN_POINT('Ctrl Pts',(-1.27696414831089,-1.,1.46916035917133));
#27170=CARTESIAN_POINT('Ctrl Pts',(-1.27696414831089,1.,1.46916035917133));
#27171=CARTESIAN_POINT('Ctrl Pts',(-1.2794891824849,-1.,1.4744717526707));
#27172=CARTESIAN_POINT('Ctrl Pts',(-1.2794891824849,1.,1.4744717526707));
#27173=CARTESIAN_POINT('Ctrl Pts',(-1.28194158939517,-1.,1.47980070347095));
#27174=CARTESIAN_POINT('Ctrl Pts',(-1.28194158939517,1.,1.47980070347095));
#27175=CARTESIAN_POINT('Ctrl Pts',(-1.28435533880201,-1.,1.4851881711891));
#27176=CARTESIAN_POINT('Ctrl Pts',(-1.28435533880201,1.,1.4851881711891));
#27177=CARTESIAN_POINT('Ctrl Pts',(-1.2867467611644,-1.,1.4906522831278));
#27178=CARTESIAN_POINT('Ctrl Pts',(-1.2867467611644,1.,1.4906522831278));
#27179=CARTESIAN_POINT('Ctrl Pts',(-1.28911506584254,-1.,1.49618896881754));
#27180=CARTESIAN_POINT('Ctrl Pts',(-1.28911506584254,1.,1.49618896881754));
#27181=CARTESIAN_POINT('Ctrl Pts',(-1.29145022885181,-1.,1.50178230149776));
#27182=CARTESIAN_POINT('Ctrl Pts',(-1.29145022885181,1.,1.50178230149776));
#27183=CARTESIAN_POINT('Ctrl Pts',(-1.29373841372842,-1.,1.50741159078365));
#27184=CARTESIAN_POINT('Ctrl Pts',(-1.29373841372842,1.,1.50741159078365));
#27185=CARTESIAN_POINT('Ctrl Pts',(-1.29596850710509,-1.,1.51305994241402));
#27186=CARTESIAN_POINT('Ctrl Pts',(-1.29596850710509,1.,1.51305994241402));
#27187=CARTESIAN_POINT('Ctrl Pts',(-1.29813791800747,-1.,1.51872184912724));
#27188=CARTESIAN_POINT('Ctrl Pts',(-1.29813791800747,1.,1.51872184912724));
#27189=CARTESIAN_POINT('Ctrl Pts',(-1.30024984366328,-1.,1.52439957861062));
#27190=CARTESIAN_POINT('Ctrl Pts',(-1.30024984366328,1.,1.52439957861062));
#27191=CARTESIAN_POINT('Ctrl Pts',(-1.30231064395568,-1.,1.53009970283891));
#27192=CARTESIAN_POINT('Ctrl Pts',(-1.30231064395568,1.,1.53009970283891));
#27193=CARTESIAN_POINT('Ctrl Pts',(-1.30432735639489,-1.,1.53582981268977));
#27194=CARTESIAN_POINT('Ctrl Pts',(-1.30432735639489,1.,1.53582981268977));
#27195=CARTESIAN_POINT('Ctrl Pts',(-1.30630475189556,-1.,1.54159462645432));
#27196=CARTESIAN_POINT('Ctrl Pts',(-1.30630475189556,1.,1.54159462645432));
#27197=CARTESIAN_POINT('Ctrl Pts',(-1.30824393907473,-1.,1.54739413957185));
#27198=CARTESIAN_POINT('Ctrl Pts',(-1.30824393907473,1.,1.54739413957185));
#27199=CARTESIAN_POINT('Ctrl Pts',(-1.31014393684222,-1.,1.55322568759481));
#27200=CARTESIAN_POINT('Ctrl Pts',(-1.31014393684222,1.,1.55322568759481));
#27201=CARTESIAN_POINT('Ctrl Pts',(-1.31200264341696,-1.,1.55908521254821));
#27202=CARTESIAN_POINT('Ctrl Pts',(-1.31200264341696,1.,1.55908521254821));
#27203=CARTESIAN_POINT('Ctrl Pts',(-1.31381795281002,-1.,1.56496872402353));
#27204=CARTESIAN_POINT('Ctrl Pts',(-1.31381795281002,1.,1.56496872402353));
#27205=CARTESIAN_POINT('Ctrl Pts',(-1.31558903860016,-1.,1.57087397835723));
#27206=CARTESIAN_POINT('Ctrl Pts',(-1.31558903860016,1.,1.57087397835723));
#27207=CARTESIAN_POINT('Ctrl Pts',(-1.31731642317187,-1.,1.5768005650559));
#27208=CARTESIAN_POINT('Ctrl Pts',(-1.31731642317187,1.,1.5768005650559));
#27209=CARTESIAN_POINT('Ctrl Pts',(-1.31900135021432,-1.,1.58274907898834));
#27210=CARTESIAN_POINT('Ctrl Pts',(-1.31900135021432,1.,1.58274907898834));
#27211=CARTESIAN_POINT('Ctrl Pts',(-1.32064537110892,-1.,1.58872057258245));
#27212=CARTESIAN_POINT('Ctrl Pts',(-1.32064537110892,1.,1.58872057258245));
#27213=CARTESIAN_POINT('Ctrl Pts',(-1.32224985747682,-1.,1.59471591079403));
#27214=CARTESIAN_POINT('Ctrl Pts',(-1.32224985747682,1.,1.59471591079403));
#27215=CARTESIAN_POINT('Ctrl Pts',(-1.32381550858256,-1.,1.60073511858687));
#27216=CARTESIAN_POINT('Ctrl Pts',(-1.32381550858256,1.,1.60073511858687));
#27217=CARTESIAN_POINT('Ctrl Pts',(-1.32534250785782,-1.,1.60677758290954));
#27218=CARTESIAN_POINT('Ctrl Pts',(-1.32534250785782,1.,1.60677758290954));
#27219=CARTESIAN_POINT('Ctrl Pts',(-1.32683074483356,-1.,1.6128423401575));
#27220=CARTESIAN_POINT('Ctrl Pts',(-1.32683074483356,1.,1.6128423401575));
#27221=CARTESIAN_POINT('Ctrl Pts',(-1.32828000610449,-1.,1.61892832270724));
#27222=CARTESIAN_POINT('Ctrl Pts',(-1.32828000610449,1.,1.61892832270724));
#27223=CARTESIAN_POINT('Ctrl Pts',(-1.3296901950568,-1.,1.62503464209797));
#27224=CARTESIAN_POINT('Ctrl Pts',(-1.3296901950568,1.,1.62503464209797));
#27225=CARTESIAN_POINT('Ctrl Pts',(-1.33106149345645,-1.,1.63116079730923));
#27226=CARTESIAN_POINT('Ctrl Pts',(-1.33106149345645,1.,1.63116079730923));
#27227=CARTESIAN_POINT('Ctrl Pts',(-1.33239425103724,-1.,1.63730653475089));
#27228=CARTESIAN_POINT('Ctrl Pts',(-1.33239425103724,1.,1.63730653475089));
#27229=CARTESIAN_POINT('Ctrl Pts',(-1.33368890676572,-1.,1.6434717485603));
#27230=CARTESIAN_POINT('Ctrl Pts',(-1.33368890676572,1.,1.6434717485603));
#27231=CARTESIAN_POINT('Ctrl Pts',(-1.33494590467993,-1.,1.6496563728683));
#27232=CARTESIAN_POINT('Ctrl Pts',(-1.33494590467993,1.,1.6496563728683));
#27233=CARTESIAN_POINT('Ctrl Pts',(-1.33616559745172,-1.,1.65586025952593));
#27234=CARTESIAN_POINT('Ctrl Pts',(-1.33616559745172,1.,1.65586025952593));
#27235=CARTESIAN_POINT('Ctrl Pts',(-1.33734820885262,-1.,1.66208312541983));
#27236=CARTESIAN_POINT('Ctrl Pts',(-1.33734820885262,1.,1.66208312541983));
#27237=CARTESIAN_POINT('Ctrl Pts',(-1.33849388654388,-1.,1.66832460783989));
#27238=CARTESIAN_POINT('Ctrl Pts',(-1.33849388654388,1.,1.66832460783989));
#27239=CARTESIAN_POINT('Ctrl Pts',(-1.3396027347034,-1.,1.67458429426086));
#27240=CARTESIAN_POINT('Ctrl Pts',(-1.3396027347034,1.,1.67458429426086));
#27241=CARTESIAN_POINT('Ctrl Pts',(-1.34067485185203,-1.,1.68086176030362));
#27242=CARTESIAN_POINT('Ctrl Pts',(-1.34067485185203,1.,1.68086176030362));
#27243=CARTESIAN_POINT('Ctrl Pts',(-1.341710374848,-1.,1.68715660868764));
#27244=CARTESIAN_POINT('Ctrl Pts',(-1.341710374848,1.,1.68715660868764));
#27245=CARTESIAN_POINT('Ctrl Pts',(-1.34270948206319,-1.,1.6934684849687));
#27246=CARTESIAN_POINT('Ctrl Pts',(-1.34270948206319,1.,1.6934684849687));
#27247=CARTESIAN_POINT('Ctrl Pts',(-1.34367237124483,-1.,1.69979707754427));
#27248=CARTESIAN_POINT('Ctrl Pts',(-1.34367237124483,1.,1.69979707754427));
#27249=CARTESIAN_POINT('Ctrl Pts',(-1.34459924533831,-1.,1.70614212266738));
#27250=CARTESIAN_POINT('Ctrl Pts',(-1.34459924533831,1.,1.70614212266738));
#27251=CARTESIAN_POINT('Ctrl Pts',(-1.34549029589416,-1.,1.71250340686822));
#27252=CARTESIAN_POINT('Ctrl Pts',(-1.34549029589416,1.,1.71250340686822));
#27253=CARTESIAN_POINT('Ctrl Pts',(-1.34634568653227,-1.,1.7188807715049));
#27254=CARTESIAN_POINT('Ctrl Pts',(-1.34634568653227,1.,1.7188807715049));
#27255=CARTESIAN_POINT('Ctrl Pts',(-1.34716554819527,-1.,1.72527410680674));
#27256=CARTESIAN_POINT('Ctrl Pts',(-1.34716554819527,1.,1.72527410680674));
#27257=CARTESIAN_POINT('Ctrl Pts',(-1.34779309152035,-1.,1.7304014965394));
#27258=CARTESIAN_POINT('Ctrl Pts',(-1.34779309152035,1.,1.7304014965394));
#27259=CARTESIAN_POINT('Ctrl Pts',(-1.34824783112887,-1.,1.73425417885907));
#27260=CARTESIAN_POINT('Ctrl Pts',(-1.34824783112887,1.,1.73425417885907));
#27261=CARTESIAN_POINT('Ctrl Pts',(-1.34854391898045,-1.,1.73682580585691));
#27262=CARTESIAN_POINT('Ctrl Pts',(-1.34854391898045,1.,1.73682580585691));
#27263=CARTESIAN_POINT('Ctrl Pts',(-1.34869019493419,-1.,1.73811241238545));
#27264=CARTESIAN_POINT('Ctrl Pts',(-1.34869019493419,1.,1.73811241238545));
#27265=CARTESIAN_POINT('',(-1.15624053661742,1.,1.31362392696032));
#27266=CARTESIAN_POINT('Ctrl Pts',(-1.15624053661742,1.,1.31362392696032));
#27267=CARTESIAN_POINT('Ctrl Pts',(-1.15950888730809,1.,1.31722977216397));
#27268=CARTESIAN_POINT('Ctrl Pts',(-1.16589330093588,1.,1.32428080721772));
#27269=CARTESIAN_POINT('Ctrl Pts',(-1.17501305789857,1.,1.33437539347008));
#27270=CARTESIAN_POINT('Ctrl Pts',(-1.18625865667441,1.,1.34687054001093));
#27271=CARTESIAN_POINT('Ctrl Pts',(-1.1987959077932,1.,1.36088705043885));
#27272=CARTESIAN_POINT('Ctrl Pts',(-1.20982812925645,1.,1.37331915607905));
#27273=CARTESIAN_POINT('Ctrl Pts',(-1.21938737280852,1.,1.38420564527715));
#27274=CARTESIAN_POINT('Ctrl Pts',(-1.22752961899387,1.,1.39361389568796));
#27275=CARTESIAN_POINT('Ctrl Pts',(-1.23434087290423,1.,1.40164708206106));
#27276=CARTESIAN_POINT('Ctrl Pts',(-1.23994455029534,1.,1.40845295531283));
#27277=CARTESIAN_POINT('Ctrl Pts',(-1.24450600513056,1.,1.41422913175179));
#27278=CARTESIAN_POINT('Ctrl Pts',(-1.24824430986571,1.,1.41923722596025));
#27279=CARTESIAN_POINT('Ctrl Pts',(-1.2514145557001,1.,1.42378102115575));
#27280=CARTESIAN_POINT('Ctrl Pts',(-1.25426945222639,1.,1.42815938799387));
#27281=CARTESIAN_POINT('Ctrl Pts',(-1.25702687965755,1.,1.43262645609691));
#27282=CARTESIAN_POINT('Ctrl Pts',(-1.25983531012005,1.,1.43734919180848));
#27283=CARTESIAN_POINT('Ctrl Pts',(-1.26273903323859,1.,1.44236470511303));
#27284=CARTESIAN_POINT('Ctrl Pts',(-1.26570925118868,1.,1.44761985001662));
#27285=CARTESIAN_POINT('Ctrl Pts',(-1.2686778680489,1.,1.45301422764247));
#27286=CARTESIAN_POINT('Ctrl Pts',(-1.27156805265289,1.,1.45843906294697));
#27287=CARTESIAN_POINT('Ctrl Pts',(-1.27433119897822,1.,1.46382431332476));
#27288=CARTESIAN_POINT('Ctrl Pts',(-1.27696414831089,1.,1.46916035917133));
#27289=CARTESIAN_POINT('Ctrl Pts',(-1.2794891824849,1.,1.4744717526707));
#27290=CARTESIAN_POINT('Ctrl Pts',(-1.28194158939517,1.,1.47980070347095));
#27291=CARTESIAN_POINT('Ctrl Pts',(-1.28435533880201,1.,1.4851881711891));
#27292=CARTESIAN_POINT('Ctrl Pts',(-1.2867467611644,1.,1.4906522831278));
#27293=CARTESIAN_POINT('Ctrl Pts',(-1.28911506584254,1.,1.49618896881754));
#27294=CARTESIAN_POINT('Ctrl Pts',(-1.29145022885181,1.,1.50178230149776));
#27295=CARTESIAN_POINT('Ctrl Pts',(-1.29373841372842,1.,1.50741159078365));
#27296=CARTESIAN_POINT('Ctrl Pts',(-1.29596850710509,1.,1.51305994241402));
#27297=CARTESIAN_POINT('Ctrl Pts',(-1.29813791800747,1.,1.51872184912724));
#27298=CARTESIAN_POINT('Ctrl Pts',(-1.30024984366328,1.,1.52439957861062));
#27299=CARTESIAN_POINT('Ctrl Pts',(-1.30231064395568,1.,1.53009970283891));
#27300=CARTESIAN_POINT('Ctrl Pts',(-1.30432735639489,1.,1.53582981268977));
#27301=CARTESIAN_POINT('Ctrl Pts',(-1.30630475189556,1.,1.54159462645432));
#27302=CARTESIAN_POINT('Ctrl Pts',(-1.30824393907473,1.,1.54739413957185));
#27303=CARTESIAN_POINT('Ctrl Pts',(-1.31014393684222,1.,1.55322568759481));
#27304=CARTESIAN_POINT('Ctrl Pts',(-1.31200264341696,1.,1.55908521254821));
#27305=CARTESIAN_POINT('Ctrl Pts',(-1.31381795281002,1.,1.56496872402353));
#27306=CARTESIAN_POINT('Ctrl Pts',(-1.31558903860016,1.,1.57087397835723));
#27307=CARTESIAN_POINT('Ctrl Pts',(-1.31731642317187,1.,1.5768005650559));
#27308=CARTESIAN_POINT('Ctrl Pts',(-1.31900135021432,1.,1.58274907898834));
#27309=CARTESIAN_POINT('Ctrl Pts',(-1.32064537110892,1.,1.58872057258245));
#27310=CARTESIAN_POINT('Ctrl Pts',(-1.32224985747682,1.,1.59471591079403));
#27311=CARTESIAN_POINT('Ctrl Pts',(-1.32381550858256,1.,1.60073511858687));
#27312=CARTESIAN_POINT('Ctrl Pts',(-1.32534250785782,1.,1.60677758290954));
#27313=CARTESIAN_POINT('Ctrl Pts',(-1.32683074483356,1.,1.6128423401575));
#27314=CARTESIAN_POINT('Ctrl Pts',(-1.32828000610449,1.,1.61892832270724));
#27315=CARTESIAN_POINT('Ctrl Pts',(-1.3296901950568,1.,1.62503464209797));
#27316=CARTESIAN_POINT('Ctrl Pts',(-1.33106149345645,1.,1.63116079730923));
#27317=CARTESIAN_POINT('Ctrl Pts',(-1.33239425103724,1.,1.63730653475089));
#27318=CARTESIAN_POINT('Ctrl Pts',(-1.33368890676572,1.,1.6434717485603));
#27319=CARTESIAN_POINT('Ctrl Pts',(-1.33494590467993,1.,1.6496563728683));
#27320=CARTESIAN_POINT('Ctrl Pts',(-1.33616559745172,1.,1.65586025952593));
#27321=CARTESIAN_POINT('Ctrl Pts',(-1.33734820885262,1.,1.66208312541983));
#27322=CARTESIAN_POINT('Ctrl Pts',(-1.33849388654388,1.,1.66832460783989));
#27323=CARTESIAN_POINT('Ctrl Pts',(-1.3396027347034,1.,1.67458429426086));
#27324=CARTESIAN_POINT('Ctrl Pts',(-1.34067485185203,1.,1.68086176030362));
#27325=CARTESIAN_POINT('Ctrl Pts',(-1.341710374848,1.,1.68715660868764));
#27326=CARTESIAN_POINT('Ctrl Pts',(-1.34270948206319,1.,1.6934684849687));
#27327=CARTESIAN_POINT('Ctrl Pts',(-1.34367237124483,1.,1.69979707754427));
#27328=CARTESIAN_POINT('Ctrl Pts',(-1.34459924533831,1.,1.70614212266738));
#27329=CARTESIAN_POINT('Ctrl Pts',(-1.34549029589416,1.,1.71250340686822));
#27330=CARTESIAN_POINT('Ctrl Pts',(-1.34634568653227,1.,1.7188807715049));
#27331=CARTESIAN_POINT('Ctrl Pts',(-1.34716554819527,1.,1.72527410680674));
#27332=CARTESIAN_POINT('Ctrl Pts',(-1.34779309152035,1.,1.7304014965394));
#27333=CARTESIAN_POINT('Ctrl Pts',(-1.34824783112887,1.,1.73425417885907));
#27334=CARTESIAN_POINT('Ctrl Pts',(-1.34854391898045,1.,1.73682580585691));
#27335=CARTESIAN_POINT('Ctrl Pts',(-1.34869019493419,1.,1.73811241238545));
#27336=CARTESIAN_POINT('',(-1.15624053661742,0.,1.31362392696032));
#27337=CARTESIAN_POINT('Origin',(0.,0.,0.));
#27338=CARTESIAN_POINT('',(-1.31362392696033,1.,1.15624053661742));
#27339=CARTESIAN_POINT('Origin',(0.,1.,0.));
#27340=CARTESIAN_POINT('',(-1.31362392696033,0.,1.15624053661742));
#27341=CARTESIAN_POINT('Ctrl Pts',(-1.73811241238545,-1.,1.34869019493419));
#27342=CARTESIAN_POINT('Ctrl Pts',(-1.73811241238545,1.,1.34869019493419));
#27343=CARTESIAN_POINT('Ctrl Pts',(-1.73682580585819,-1.,1.34854391898145));
#27344=CARTESIAN_POINT('Ctrl Pts',(-1.73682580585819,1.,1.34854391898145));
#27345=CARTESIAN_POINT('Ctrl Pts',(-1.73425417886255,-1.,1.34824783113158));
#27346=CARTESIAN_POINT('Ctrl Pts',(-1.73425417886255,1.,1.34824783113158));
#27347=CARTESIAN_POINT('Ctrl Pts',(-1.73040149654497,-1.,1.3477930915247));
#27348=CARTESIAN_POINT('Ctrl Pts',(-1.73040149654497,1.,1.3477930915247));
#27349=CARTESIAN_POINT('Ctrl Pts',(-1.72527410681298,-1.,1.34716554820013));
#27350=CARTESIAN_POINT('Ctrl Pts',(-1.72527410681298,1.,1.34716554820013));
#27351=CARTESIAN_POINT('Ctrl Pts',(-1.7188807715095,-1.,1.34634568653586));
#27352=CARTESIAN_POINT('Ctrl Pts',(-1.7188807715095,1.,1.34634568653586));
#27353=CARTESIAN_POINT('Ctrl Pts',(-1.71250340687011,-1.,1.34549029589563));
#27354=CARTESIAN_POINT('Ctrl Pts',(-1.71250340687011,1.,1.34549029589563));
#27355=CARTESIAN_POINT('Ctrl Pts',(-1.70614212266676,-1.,1.34459924533783));
#27356=CARTESIAN_POINT('Ctrl Pts',(-1.70614212266676,1.,1.34459924533783));
#27357=CARTESIAN_POINT('Ctrl Pts',(-1.69979707754221,-1.,1.34367237124322));
#27358=CARTESIAN_POINT('Ctrl Pts',(-1.69979707754221,1.,1.34367237124322));
#27359=CARTESIAN_POINT('Ctrl Pts',(-1.6934684849664,-1.,1.34270948206139));
#27360=CARTESIAN_POINT('Ctrl Pts',(-1.6934684849664,1.,1.34270948206139));
#27361=CARTESIAN_POINT('Ctrl Pts',(-1.68715660868602,-1.,1.34171037484673));
#27362=CARTESIAN_POINT('Ctrl Pts',(-1.68715660868602,1.,1.34171037484673));
#27363=CARTESIAN_POINT('Ctrl Pts',(-1.68086176030308,-1.,1.3406748518516));
#27364=CARTESIAN_POINT('Ctrl Pts',(-1.68086176030308,1.,1.3406748518516));
#27365=CARTESIAN_POINT('Ctrl Pts',(-1.67458429426126,-1.,1.33960273470372));
#27366=CARTESIAN_POINT('Ctrl Pts',(-1.67458429426126,1.,1.33960273470372));
#27367=CARTESIAN_POINT('Ctrl Pts',(-1.66832460784078,-1.,1.33849388654458));
#27368=CARTESIAN_POINT('Ctrl Pts',(-1.66832460784078,1.,1.33849388654458));
#27369=CARTESIAN_POINT('Ctrl Pts',(-1.66208312542073,-1.,1.33734820885331));
#27370=CARTESIAN_POINT('Ctrl Pts',(-1.66208312542073,1.,1.33734820885331));
#27371=CARTESIAN_POINT('Ctrl Pts',(-1.65586025952651,-1.,1.33616559745217));
#27372=CARTESIAN_POINT('Ctrl Pts',(-1.65586025952651,1.,1.33616559745217));
#27373=CARTESIAN_POINT('Ctrl Pts',(-1.64965637286843,-1.,1.33494590468003));
#27374=CARTESIAN_POINT('Ctrl Pts',(-1.64965637286843,1.,1.33494590468003));
#27375=CARTESIAN_POINT('Ctrl Pts',(-1.64347174856007,-1.,1.33368890676554));
#27376=CARTESIAN_POINT('Ctrl Pts',(-1.64347174856007,1.,1.33368890676554));
#27377=CARTESIAN_POINT('Ctrl Pts',(-1.6373065347505,-1.,1.33239425103694));
#27378=CARTESIAN_POINT('Ctrl Pts',(-1.6373065347505,1.,1.33239425103694));
#27379=CARTESIAN_POINT('Ctrl Pts',(-1.63116079730887,-1.,1.33106149345618));
#27380=CARTESIAN_POINT('Ctrl Pts',(-1.63116079730887,1.,1.33106149345618));
#27381=CARTESIAN_POINT('Ctrl Pts',(-1.62503464209777,-1.,1.32969019505665));
#27382=CARTESIAN_POINT('Ctrl Pts',(-1.62503464209777,1.,1.32969019505665));
#27383=CARTESIAN_POINT('Ctrl Pts',(-1.61892832270723,-1.,1.32828000610448));
#27384=CARTESIAN_POINT('Ctrl Pts',(-1.61892832270723,1.,1.32828000610448));
#27385=CARTESIAN_POINT('Ctrl Pts',(-1.61284234015762,-1.,1.32683074483365));
#27386=CARTESIAN_POINT('Ctrl Pts',(-1.61284234015762,1.,1.32683074483365));
#27387=CARTESIAN_POINT('Ctrl Pts',(-1.6067775829097,-1.,1.32534250785794));
#27388=CARTESIAN_POINT('Ctrl Pts',(-1.6067775829097,1.,1.32534250785794));
#27389=CARTESIAN_POINT('Ctrl Pts',(-1.600735118587,-1.,1.32381550858266));
#27390=CARTESIAN_POINT('Ctrl Pts',(-1.600735118587,1.,1.32381550858266));
#27391=CARTESIAN_POINT('Ctrl Pts',(-1.59471591079408,-1.,1.32224985747686));
#27392=CARTESIAN_POINT('Ctrl Pts',(-1.59471591079408,1.,1.32224985747686));
#27393=CARTESIAN_POINT('Ctrl Pts',(-1.58872057258244,-1.,1.32064537110891));
#27394=CARTESIAN_POINT('Ctrl Pts',(-1.58872057258244,1.,1.32064537110891));
#27395=CARTESIAN_POINT('Ctrl Pts',(-1.58274907898829,-1.,1.31900135021428));
#27396=CARTESIAN_POINT('Ctrl Pts',(-1.58274907898829,1.,1.31900135021428));
#27397=CARTESIAN_POINT('Ctrl Pts',(-1.57680056505585,-1.,1.31731642317183));
#27398=CARTESIAN_POINT('Ctrl Pts',(-1.57680056505585,1.,1.31731642317183));
#27399=CARTESIAN_POINT('Ctrl Pts',(-1.57087397835721,-1.,1.31558903860015));
#27400=CARTESIAN_POINT('Ctrl Pts',(-1.57087397835721,1.,1.31558903860015));
#27401=CARTESIAN_POINT('Ctrl Pts',(-1.56496872402352,-1.,1.31381795281002));
#27402=CARTESIAN_POINT('Ctrl Pts',(-1.56496872402352,1.,1.31381795281002));
#27403=CARTESIAN_POINT('Ctrl Pts',(-1.55908521254822,-1.,1.31200264341696));
#27404=CARTESIAN_POINT('Ctrl Pts',(-1.55908521254822,1.,1.31200264341696));
#27405=CARTESIAN_POINT('Ctrl Pts',(-1.55322568759481,-1.,1.31014393684221));
#27406=CARTESIAN_POINT('Ctrl Pts',(-1.55322568759481,1.,1.31014393684221));
#27407=CARTESIAN_POINT('Ctrl Pts',(-1.54739413957183,-1.,1.30824393907471));
#27408=CARTESIAN_POINT('Ctrl Pts',(-1.54739413957183,1.,1.30824393907471));
#27409=CARTESIAN_POINT('Ctrl Pts',(-1.54159462645428,-1.,1.30630475189553));
#27410=CARTESIAN_POINT('Ctrl Pts',(-1.54159462645428,1.,1.30630475189553));
#27411=CARTESIAN_POINT('Ctrl Pts',(-1.53582981268976,-1.,1.30432735639487));
#27412=CARTESIAN_POINT('Ctrl Pts',(-1.53582981268976,1.,1.30432735639487));
#27413=CARTESIAN_POINT('Ctrl Pts',(-1.53009970283893,-1.,1.3023106439557));
#27414=CARTESIAN_POINT('Ctrl Pts',(-1.53009970283893,1.,1.3023106439557));
#27415=CARTESIAN_POINT('Ctrl Pts',(-1.5243995786107,-1.,1.30024984366334));
#27416=CARTESIAN_POINT('Ctrl Pts',(-1.5243995786107,1.,1.30024984366334));
#27417=CARTESIAN_POINT('Ctrl Pts',(-1.51872184912735,-1.,1.29813791800757));
#27418=CARTESIAN_POINT('Ctrl Pts',(-1.51872184912735,1.,1.29813791800757));
#27419=CARTESIAN_POINT('Ctrl Pts',(-1.51305994241412,-1.,1.29596850710518));
#27420=CARTESIAN_POINT('Ctrl Pts',(-1.51305994241412,1.,1.29596850710518));
#27421=CARTESIAN_POINT('Ctrl Pts',(-1.50741159078367,-1.,1.29373841372843));
#27422=CARTESIAN_POINT('Ctrl Pts',(-1.50741159078367,1.,1.29373841372843));
#27423=CARTESIAN_POINT('Ctrl Pts',(-1.50178230149764,-1.,1.29145022885171));
#27424=CARTESIAN_POINT('Ctrl Pts',(-1.50178230149764,1.,1.29145022885171));
#27425=CARTESIAN_POINT('Ctrl Pts',(-1.49618896881729,-1.,1.28911506584232));
#27426=CARTESIAN_POINT('Ctrl Pts',(-1.49618896881729,1.,1.28911506584232));
#27427=CARTESIAN_POINT('Ctrl Pts',(-1.4906522831275,-1.,1.28674676116415));
#27428=CARTESIAN_POINT('Ctrl Pts',(-1.4906522831275,1.,1.28674676116415));
#27429=CARTESIAN_POINT('Ctrl Pts',(-1.48518817118891,-1.,1.28435533880184));
#27430=CARTESIAN_POINT('Ctrl Pts',(-1.48518817118891,1.,1.28435533880184));
#27431=CARTESIAN_POINT('Ctrl Pts',(-1.47980070347102,-1.,1.28194158939522));
#27432=CARTESIAN_POINT('Ctrl Pts',(-1.47980070347102,1.,1.28194158939522));
#27433=CARTESIAN_POINT('Ctrl Pts',(-1.4744717526711,-1.,1.27948918248524));
#27434=CARTESIAN_POINT('Ctrl Pts',(-1.4744717526711,1.,1.27948918248524));
#27435=CARTESIAN_POINT('Ctrl Pts',(-1.46916035917197,-1.,1.27696414831144));
#27436=CARTESIAN_POINT('Ctrl Pts',(-1.46916035917197,1.,1.27696414831144));
#27437=CARTESIAN_POINT('Ctrl Pts',(-1.4638243133254,-1.,1.27433119897877));
#27438=CARTESIAN_POINT('Ctrl Pts',(-1.4638243133254,1.,1.27433119897877));
#27439=CARTESIAN_POINT('Ctrl Pts',(-1.45843906294725,-1.,1.27156805265312));
#27440=CARTESIAN_POINT('Ctrl Pts',(-1.45843906294725,1.,1.27156805265312));
#27441=CARTESIAN_POINT('Ctrl Pts',(-1.45301422764205,-1.,1.26867786804854));
#27442=CARTESIAN_POINT('Ctrl Pts',(-1.45301422764205,1.,1.26867786804854));
#27443=CARTESIAN_POINT('Ctrl Pts',(-1.44761985001544,-1.,1.26570925118767));
#27444=CARTESIAN_POINT('Ctrl Pts',(-1.44761985001544,1.,1.26570925118767));
#27445=CARTESIAN_POINT('Ctrl Pts',(-1.44236470511145,-1.,1.26273903323723));
#27446=CARTESIAN_POINT('Ctrl Pts',(-1.44236470511145,1.,1.26273903323723));
#27447=CARTESIAN_POINT('Ctrl Pts',(-1.43734919180719,-1.,1.25983531011894));
#27448=CARTESIAN_POINT('Ctrl Pts',(-1.43734919180719,1.,1.25983531011894));
#27449=CARTESIAN_POINT('Ctrl Pts',(-1.43262645609679,-1.,1.25702687965744));
#27450=CARTESIAN_POINT('Ctrl Pts',(-1.43262645609679,1.,1.25702687965744));
#27451=CARTESIAN_POINT('Ctrl Pts',(-1.42815938799555,-1.,1.25426945222783));
#27452=CARTESIAN_POINT('Ctrl Pts',(-1.42815938799555,1.,1.25426945222783));
#27453=CARTESIAN_POINT('Ctrl Pts',(-1.42378102115911,-1.,1.25141455570299));
#27454=CARTESIAN_POINT('Ctrl Pts',(-1.42378102115911,1.,1.25141455570299));
#27455=CARTESIAN_POINT('Ctrl Pts',(-1.41923722596421,-1.,1.24824430986911));
#27456=CARTESIAN_POINT('Ctrl Pts',(-1.41923722596421,1.,1.24824430986911));
#27457=CARTESIAN_POINT('Ctrl Pts',(-1.41422913175437,-1.,1.24450600513278));
#27458=CARTESIAN_POINT('Ctrl Pts',(-1.41422913175437,1.,1.24450600513278));
#27459=CARTESIAN_POINT('Ctrl Pts',(-1.40845295531151,-1.,1.23994455029421));
#27460=CARTESIAN_POINT('Ctrl Pts',(-1.40845295531151,1.,1.23994455029421));
#27461=CARTESIAN_POINT('Ctrl Pts',(-1.40164708205345,-1.,1.23434087289768));
#27462=CARTESIAN_POINT('Ctrl Pts',(-1.40164708205345,1.,1.23434087289768));
#27463=CARTESIAN_POINT('Ctrl Pts',(-1.39361389567257,-1.,1.22752961898063));
#27464=CARTESIAN_POINT('Ctrl Pts',(-1.39361389567257,1.,1.22752961898063));
#27465=CARTESIAN_POINT('Ctrl Pts',(-1.38420564525391,-1.,1.21938737278853));
#27466=CARTESIAN_POINT('Ctrl Pts',(-1.38420564525391,1.,1.21938737278853));
#27467=CARTESIAN_POINT('Ctrl Pts',(-1.37331915604962,-1.,1.20982812923113));
#27468=CARTESIAN_POINT('Ctrl Pts',(-1.37331915604962,1.,1.20982812923113));
#27469=CARTESIAN_POINT('Ctrl Pts',(-1.36088705040677,-1.,1.1987959077656));
#27470=CARTESIAN_POINT('Ctrl Pts',(-1.36088705040677,1.,1.1987959077656));
#27471=CARTESIAN_POINT('Ctrl Pts',(-1.34687053998157,-1.,1.18625865664915));
#27472=CARTESIAN_POINT('Ctrl Pts',(-1.34687053998157,1.,1.18625865664915));
#27473=CARTESIAN_POINT('Ctrl Pts',(-1.33437539344842,-1.,1.17501305787994));
#27474=CARTESIAN_POINT('Ctrl Pts',(-1.33437539344842,1.,1.17501305787994));
#27475=CARTESIAN_POINT('Ctrl Pts',(-1.32428080720544,-1.,1.16589330092532));
#27476=CARTESIAN_POINT('Ctrl Pts',(-1.32428080720544,1.,1.16589330092532));
#27477=CARTESIAN_POINT('Ctrl Pts',(-1.3172297721596,-1.,1.15950888730433));
#27478=CARTESIAN_POINT('Ctrl Pts',(-1.3172297721596,1.,1.15950888730433));
#27479=CARTESIAN_POINT('Ctrl Pts',(-1.31362392696033,-1.,1.15624053661742));
#27480=CARTESIAN_POINT('Ctrl Pts',(-1.31362392696033,1.,1.15624053661742));
#27481=CARTESIAN_POINT('',(-1.73811241238545,1.,1.34869019493419));
#27482=CARTESIAN_POINT('Ctrl Pts',(-1.73811241238545,1.,1.34869019493419));
#27483=CARTESIAN_POINT('Ctrl Pts',(-1.73682580585819,1.,1.34854391898145));
#27484=CARTESIAN_POINT('Ctrl Pts',(-1.73425417886255,1.,1.34824783113158));
#27485=CARTESIAN_POINT('Ctrl Pts',(-1.73040149654497,1.,1.3477930915247));
#27486=CARTESIAN_POINT('Ctrl Pts',(-1.72527410681298,1.,1.34716554820013));
#27487=CARTESIAN_POINT('Ctrl Pts',(-1.7188807715095,1.,1.34634568653586));
#27488=CARTESIAN_POINT('Ctrl Pts',(-1.71250340687011,1.,1.34549029589563));
#27489=CARTESIAN_POINT('Ctrl Pts',(-1.70614212266676,1.,1.34459924533783));
#27490=CARTESIAN_POINT('Ctrl Pts',(-1.69979707754221,1.,1.34367237124322));
#27491=CARTESIAN_POINT('Ctrl Pts',(-1.6934684849664,1.,1.34270948206139));
#27492=CARTESIAN_POINT('Ctrl Pts',(-1.68715660868602,1.,1.34171037484673));
#27493=CARTESIAN_POINT('Ctrl Pts',(-1.68086176030308,1.,1.3406748518516));
#27494=CARTESIAN_POINT('Ctrl Pts',(-1.67458429426126,1.,1.33960273470372));
#27495=CARTESIAN_POINT('Ctrl Pts',(-1.66832460784078,1.,1.33849388654458));
#27496=CARTESIAN_POINT('Ctrl Pts',(-1.66208312542073,1.,1.33734820885331));
#27497=CARTESIAN_POINT('Ctrl Pts',(-1.65586025952651,1.,1.33616559745217));
#27498=CARTESIAN_POINT('Ctrl Pts',(-1.64965637286843,1.,1.33494590468003));
#27499=CARTESIAN_POINT('Ctrl Pts',(-1.64347174856007,1.,1.33368890676554));
#27500=CARTESIAN_POINT('Ctrl Pts',(-1.6373065347505,1.,1.33239425103694));
#27501=CARTESIAN_POINT('Ctrl Pts',(-1.63116079730887,1.,1.33106149345618));
#27502=CARTESIAN_POINT('Ctrl Pts',(-1.62503464209777,1.,1.32969019505665));
#27503=CARTESIAN_POINT('Ctrl Pts',(-1.61892832270723,1.,1.32828000610448));
#27504=CARTESIAN_POINT('Ctrl Pts',(-1.61284234015762,1.,1.32683074483365));
#27505=CARTESIAN_POINT('Ctrl Pts',(-1.6067775829097,1.,1.32534250785794));
#27506=CARTESIAN_POINT('Ctrl Pts',(-1.600735118587,1.,1.32381550858266));
#27507=CARTESIAN_POINT('Ctrl Pts',(-1.59471591079408,1.,1.32224985747686));
#27508=CARTESIAN_POINT('Ctrl Pts',(-1.58872057258244,1.,1.32064537110891));
#27509=CARTESIAN_POINT('Ctrl Pts',(-1.58274907898829,1.,1.31900135021428));
#27510=CARTESIAN_POINT('Ctrl Pts',(-1.57680056505585,1.,1.31731642317183));
#27511=CARTESIAN_POINT('Ctrl Pts',(-1.57087397835721,1.,1.31558903860015));
#27512=CARTESIAN_POINT('Ctrl Pts',(-1.56496872402352,1.,1.31381795281002));
#27513=CARTESIAN_POINT('Ctrl Pts',(-1.55908521254822,1.,1.31200264341696));
#27514=CARTESIAN_POINT('Ctrl Pts',(-1.55322568759481,1.,1.31014393684221));
#27515=CARTESIAN_POINT('Ctrl Pts',(-1.54739413957183,1.,1.30824393907471));
#27516=CARTESIAN_POINT('Ctrl Pts',(-1.54159462645428,1.,1.30630475189553));
#27517=CARTESIAN_POINT('Ctrl Pts',(-1.53582981268976,1.,1.30432735639487));
#27518=CARTESIAN_POINT('Ctrl Pts',(-1.53009970283893,1.,1.3023106439557));
#27519=CARTESIAN_POINT('Ctrl Pts',(-1.5243995786107,1.,1.30024984366334));
#27520=CARTESIAN_POINT('Ctrl Pts',(-1.51872184912735,1.,1.29813791800757));
#27521=CARTESIAN_POINT('Ctrl Pts',(-1.51305994241412,1.,1.29596850710518));
#27522=CARTESIAN_POINT('Ctrl Pts',(-1.50741159078367,1.,1.29373841372843));
#27523=CARTESIAN_POINT('Ctrl Pts',(-1.50178230149764,1.,1.29145022885171));
#27524=CARTESIAN_POINT('Ctrl Pts',(-1.49618896881729,1.,1.28911506584232));
#27525=CARTESIAN_POINT('Ctrl Pts',(-1.4906522831275,1.,1.28674676116415));
#27526=CARTESIAN_POINT('Ctrl Pts',(-1.48518817118891,1.,1.28435533880184));
#27527=CARTESIAN_POINT('Ctrl Pts',(-1.47980070347102,1.,1.28194158939522));
#27528=CARTESIAN_POINT('Ctrl Pts',(-1.4744717526711,1.,1.27948918248524));
#27529=CARTESIAN_POINT('Ctrl Pts',(-1.46916035917197,1.,1.27696414831144));
#27530=CARTESIAN_POINT('Ctrl Pts',(-1.4638243133254,1.,1.27433119897877));
#27531=CARTESIAN_POINT('Ctrl Pts',(-1.45843906294725,1.,1.27156805265312));
#27532=CARTESIAN_POINT('Ctrl Pts',(-1.45301422764205,1.,1.26867786804854));
#27533=CARTESIAN_POINT('Ctrl Pts',(-1.44761985001544,1.,1.26570925118767));
#27534=CARTESIAN_POINT('Ctrl Pts',(-1.44236470511145,1.,1.26273903323723));
#27535=CARTESIAN_POINT('Ctrl Pts',(-1.43734919180719,1.,1.25983531011894));
#27536=CARTESIAN_POINT('Ctrl Pts',(-1.43262645609679,1.,1.25702687965744));
#27537=CARTESIAN_POINT('Ctrl Pts',(-1.42815938799555,1.,1.25426945222783));
#27538=CARTESIAN_POINT('Ctrl Pts',(-1.42378102115911,1.,1.25141455570299));
#27539=CARTESIAN_POINT('Ctrl Pts',(-1.41923722596421,1.,1.24824430986911));
#27540=CARTESIAN_POINT('Ctrl Pts',(-1.41422913175437,1.,1.24450600513278));
#27541=CARTESIAN_POINT('Ctrl Pts',(-1.40845295531151,1.,1.23994455029421));
#27542=CARTESIAN_POINT('Ctrl Pts',(-1.40164708205345,1.,1.23434087289768));
#27543=CARTESIAN_POINT('Ctrl Pts',(-1.39361389567257,1.,1.22752961898063));
#27544=CARTESIAN_POINT('Ctrl Pts',(-1.38420564525391,1.,1.21938737278853));
#27545=CARTESIAN_POINT('Ctrl Pts',(-1.37331915604962,1.,1.20982812923113));
#27546=CARTESIAN_POINT('Ctrl Pts',(-1.36088705040677,1.,1.1987959077656));
#27547=CARTESIAN_POINT('Ctrl Pts',(-1.34687053998157,1.,1.18625865664915));
#27548=CARTESIAN_POINT('Ctrl Pts',(-1.33437539344842,1.,1.17501305787994));
#27549=CARTESIAN_POINT('Ctrl Pts',(-1.32428080720544,1.,1.16589330092532));
#27550=CARTESIAN_POINT('Ctrl Pts',(-1.3172297721596,1.,1.15950888730433));
#27551=CARTESIAN_POINT('Ctrl Pts',(-1.31362392696033,1.,1.15624053661742));
#27552=CARTESIAN_POINT('',(-1.73811241238545,0.,1.34869019493419));
#27553=CARTESIAN_POINT('Origin',(-1.81978687191668,0.,1.23627494547115));
#27554=CARTESIAN_POINT('',(-1.81978687191668,1.,1.23627494547115));
#27555=CARTESIAN_POINT('',(-1.73811241238545,1.,1.34869019493419));
#27556=CARTESIAN_POINT('',(-1.81978687191668,0.,1.23627494547115));
#27557=CARTESIAN_POINT('Ctrl Pts',(-1.5055822144029,-1.,0.892032620296855));
#27558=CARTESIAN_POINT('Ctrl Pts',(-1.5055822144029,1.,0.892032620296855));
#27559=CARTESIAN_POINT('Ctrl Pts',(-1.50980486807181,-1.,0.894452006967538));
#27560=CARTESIAN_POINT('Ctrl Pts',(-1.50980486807181,1.,0.894452006967538));
#27561=CARTESIAN_POINT('Ctrl Pts',(-1.51805569591479,-1.,0.89918504749193));
#27562=CARTESIAN_POINT('Ctrl Pts',(-1.51805569591479,1.,0.89918504749193));
#27563=CARTESIAN_POINT('Ctrl Pts',(-1.52984849890434,-1.,0.905967409640499));
#27564=CARTESIAN_POINT('Ctrl Pts',(-1.52984849890434,1.,0.905967409640499));
#27565=CARTESIAN_POINT('Ctrl Pts',(-1.54440491152808,-1.,0.91437591904658));
#27566=CARTESIAN_POINT('Ctrl Pts',(-1.54440491152808,1.,0.91437591904658));
#27567=CARTESIAN_POINT('Ctrl Pts',(-1.56065988582509,-1.,0.923832188966322));
#27568=CARTESIAN_POINT('Ctrl Pts',(-1.56065988582509,1.,0.923832188966322));
#27569=CARTESIAN_POINT('Ctrl Pts',(-1.57499388385561,-1.,0.932246680128849));
#27570=CARTESIAN_POINT('Ctrl Pts',(-1.57499388385561,1.,0.932246680128849));
#27571=CARTESIAN_POINT('Ctrl Pts',(-1.58744937489796,-1.,0.939646377909319));
#27572=CARTESIAN_POINT('Ctrl Pts',(-1.58744937489796,1.,0.939646377909319));
#27573=CARTESIAN_POINT('Ctrl Pts',(-1.59810042045408,-1.,0.946078063325796));
#27574=CARTESIAN_POINT('Ctrl Pts',(-1.59810042045408,1.,0.946078063325796));
#27575=CARTESIAN_POINT('Ctrl Pts',(-1.60706069897794,-1.,0.951613284361248));
#27576=CARTESIAN_POINT('Ctrl Pts',(-1.60706069897794,1.,0.951613284361248));
#27577=CARTESIAN_POINT('Ctrl Pts',(-1.61449324337233,-1.,0.956354422921573));
#27578=CARTESIAN_POINT('Ctrl Pts',(-1.61449324337233,1.,0.956354422921573));
#27579=CARTESIAN_POINT('Ctrl Pts',(-1.62061638139929,-1.,0.960438326099958));
#27580=CARTESIAN_POINT('Ctrl Pts',(-1.62061638139929,1.,0.960438326099958));
#27581=CARTESIAN_POINT('Ctrl Pts',(-1.6257193066974,-1.,0.964046107037821));
#27582=CARTESIAN_POINT('Ctrl Pts',(-1.6257193066974,1.,0.964046107037821));
#27583=CARTESIAN_POINT('Ctrl Pts',(-1.63013849959083,-1.,0.967387853228041));
#27584=CARTESIAN_POINT('Ctrl Pts',(-1.63013849959083,1.,0.967387853228041));
#27585=CARTESIAN_POINT('Ctrl Pts',(-1.63420665729609,-1.,0.970669715996356));
#27586=CARTESIAN_POINT('Ctrl Pts',(-1.63420665729609,1.,0.970669715996356));
#27587=CARTESIAN_POINT('Ctrl Pts',(-1.63820952658157,-1.,0.974066058287501));
#27588=CARTESIAN_POINT('Ctrl Pts',(-1.63820952658157,1.,0.974066058287501));
#27589=CARTESIAN_POINT('Ctrl Pts',(-1.64233990826831,-1.,0.977689794120297));
#27590=CARTESIAN_POINT('Ctrl Pts',(-1.64233990826831,1.,0.977689794120297));
#27591=CARTESIAN_POINT('Ctrl Pts',(-1.64665139190834,-1.,0.981562530940574));
#27592=CARTESIAN_POINT('Ctrl Pts',(-1.64665139190834,1.,0.981562530940574));
#27593=CARTESIAN_POINT('Ctrl Pts',(-1.6511001661277,-1.,0.985642622921626));
#27594=CARTESIAN_POINT('Ctrl Pts',(-1.6511001661277,1.,0.985642622921626));
#27595=CARTESIAN_POINT('Ctrl Pts',(-1.65559044289746,-1.,0.98985562785445));
#27596=CARTESIAN_POINT('Ctrl Pts',(-1.65559044289746,1.,0.98985562785445));
#27597=CARTESIAN_POINT('Ctrl Pts',(-1.66001553809916,-1.,0.994121836661116));
#27598=CARTESIAN_POINT('Ctrl Pts',(-1.66001553809916,1.,0.994121836661116));
#27599=CARTESIAN_POINT('Ctrl Pts',(-1.66430758030304,-1.,0.998389654952317));
#27600=CARTESIAN_POINT('Ctrl Pts',(-1.66430758030304,1.,0.998389654952317));
#27601=CARTESIAN_POINT('Ctrl Pts',(-1.66846059277231,-1.,1.00265091003682));
#27602=CARTESIAN_POINT('Ctrl Pts',(-1.66846059277231,1.,1.00265091003682));
#27603=CARTESIAN_POINT('Ctrl Pts',(-1.67250335383248,-1.,1.00692206696387));
#27604=CARTESIAN_POINT('Ctrl Pts',(-1.67250335383248,1.,1.00692206696387));
#27605=CARTESIAN_POINT('Ctrl Pts',(-1.67648246776457,-1.,1.01123236493507));
#27606=CARTESIAN_POINT('Ctrl Pts',(-1.67648246776457,1.,1.01123236493507));
#27607=CARTESIAN_POINT('Ctrl Pts',(-1.6804428989482,-1.,1.01561026162787));
#27608=CARTESIAN_POINT('Ctrl Pts',(-1.6804428989482,1.,1.01561026162787));
#27609=CARTESIAN_POINT('Ctrl Pts',(-1.68440578021739,-1.,1.02006795074222));
#27610=CARTESIAN_POINT('Ctrl Pts',(-1.68440578021739,1.,1.02006795074222));
#27611=CARTESIAN_POINT('Ctrl Pts',(-1.68836910178475,-1.,1.02460180535272));
#27612=CARTESIAN_POINT('Ctrl Pts',(-1.68836910178475,1.,1.02460180535272));
#27613=CARTESIAN_POINT('Ctrl Pts',(-1.69231840863471,-1.,1.02919977579155));
#27614=CARTESIAN_POINT('Ctrl Pts',(-1.69231840863471,1.,1.02919977579155));
#27615=CARTESIAN_POINT('Ctrl Pts',(-1.69623414782769,-1.,1.03384646003587));
#27616=CARTESIAN_POINT('Ctrl Pts',(-1.69623414782769,1.,1.03384646003587));
#27617=CARTESIAN_POINT('Ctrl Pts',(-1.70010052930951,-1.,1.03852922490782));
#27618=CARTESIAN_POINT('Ctrl Pts',(-1.70010052930951,1.,1.03852922490782));
#27619=CARTESIAN_POINT('Ctrl Pts',(-1.70391338707969,-1.,1.04324363334546));
#27620=CARTESIAN_POINT('Ctrl Pts',(-1.70391338707969,1.,1.04324363334546));
#27621=CARTESIAN_POINT('Ctrl Pts',(-1.70767646263641,-1.,1.0479908540499));
#27622=CARTESIAN_POINT('Ctrl Pts',(-1.70767646263641,1.,1.0479908540499));
#27623=CARTESIAN_POINT('Ctrl Pts',(-1.71139783543986,-1.,1.05277517202854));
#27624=CARTESIAN_POINT('Ctrl Pts',(-1.71139783543986,1.,1.05277517202854));
#27625=CARTESIAN_POINT('Ctrl Pts',(-1.71508654427022,-1.,1.05760163192481));
#27626=CARTESIAN_POINT('Ctrl Pts',(-1.71508654427022,1.,1.05760163192481));
#27627=CARTESIAN_POINT('Ctrl Pts',(-1.71874858456908,-1.,1.0624732468065));
#27628=CARTESIAN_POINT('Ctrl Pts',(-1.71874858456908,1.,1.0624732468065));
#27629=CARTESIAN_POINT('Ctrl Pts',(-1.72238500928456,-1.,1.06738966975463));
#27630=CARTESIAN_POINT('Ctrl Pts',(-1.72238500928456,1.,1.06738966975463));
#27631=CARTESIAN_POINT('Ctrl Pts',(-1.72599406198489,-1.,1.07234866990252));
#27632=CARTESIAN_POINT('Ctrl Pts',(-1.72599406198489,1.,1.07234866990252));
#27633=CARTESIAN_POINT('Ctrl Pts',(-1.72957248977424,-1.,1.0773470373727));
#27634=CARTESIAN_POINT('Ctrl Pts',(-1.72957248977424,1.,1.0773470373727));
#27635=CARTESIAN_POINT('Ctrl Pts',(-1.73311705663407,-1.,1.08238162784749));
#27636=CARTESIAN_POINT('Ctrl Pts',(-1.73311705663407,1.,1.08238162784749));
#27637=CARTESIAN_POINT('Ctrl Pts',(-1.73662628326093,-1.,1.08745056285429));
#27638=CARTESIAN_POINT('Ctrl Pts',(-1.73662628326093,1.,1.08745056285429));
#27639=CARTESIAN_POINT('Ctrl Pts',(-1.74010053962252,-1.,1.09255329056496));
#27640=CARTESIAN_POINT('Ctrl Pts',(-1.74010053962252,1.,1.09255329056496));
#27641=CARTESIAN_POINT('Ctrl Pts',(-1.74354119236212,-1.,1.09768999241229));
#27642=CARTESIAN_POINT('Ctrl Pts',(-1.74354119236212,1.,1.09768999241229));
#27643=CARTESIAN_POINT('Ctrl Pts',(-1.74695004214924,-1.,1.10286118991144));
#27644=CARTESIAN_POINT('Ctrl Pts',(-1.74695004214924,1.,1.10286118991144));
#27645=CARTESIAN_POINT('Ctrl Pts',(-1.75032866075914,-1.,1.10806728183003));
#27646=CARTESIAN_POINT('Ctrl Pts',(-1.75032866075914,1.,1.10806728183003));
#27647=CARTESIAN_POINT('Ctrl Pts',(-1.75367772094617,-1.,1.11330807582542));
#27648=CARTESIAN_POINT('Ctrl Pts',(-1.75367772094617,1.,1.11330807582542));
#27649=CARTESIAN_POINT('Ctrl Pts',(-1.75699720772089,-1.,1.11858293216752));
#27650=CARTESIAN_POINT('Ctrl Pts',(-1.75699720772089,1.,1.11858293216752));
#27651=CARTESIAN_POINT('Ctrl Pts',(-1.76028671825084,-1.,1.12389096855078));
#27652=CARTESIAN_POINT('Ctrl Pts',(-1.76028671825084,1.,1.12389096855078));
#27653=CARTESIAN_POINT('Ctrl Pts',(-1.76354571966171,-1.,1.12923123555076));
#27654=CARTESIAN_POINT('Ctrl Pts',(-1.76354571966171,1.,1.12923123555076));
#27655=CARTESIAN_POINT('Ctrl Pts',(-1.76677384551883,-1.,1.13460291804635));
#27656=CARTESIAN_POINT('Ctrl Pts',(-1.76677384551883,1.,1.13460291804635));
#27657=CARTESIAN_POINT('Ctrl Pts',(-1.76997111386806,-1.,1.14000548337));
#27658=CARTESIAN_POINT('Ctrl Pts',(-1.76997111386806,1.,1.14000548337));
#27659=CARTESIAN_POINT('Ctrl Pts',(-1.77313777896234,-1.,1.14543858226948));
#27660=CARTESIAN_POINT('Ctrl Pts',(-1.77313777896234,1.,1.14543858226948));
#27661=CARTESIAN_POINT('Ctrl Pts',(-1.77627422557034,-1.,1.15090197841531));
#27662=CARTESIAN_POINT('Ctrl Pts',(-1.77627422557034,1.,1.15090197841531));
#27663=CARTESIAN_POINT('Ctrl Pts',(-1.77938085564261,-1.,1.15639547194689));
#27664=CARTESIAN_POINT('Ctrl Pts',(-1.77938085564261,1.,1.15639547194689));
#27665=CARTESIAN_POINT('Ctrl Pts',(-1.78245795880949,-1.,1.16191881298458));
#27666=CARTESIAN_POINT('Ctrl Pts',(-1.78245795880949,1.,1.16191881298458));
#27667=CARTESIAN_POINT('Ctrl Pts',(-1.78550566040349,-1.,1.16747166312239));
#27668=CARTESIAN_POINT('Ctrl Pts',(-1.78550566040349,1.,1.16747166312239));
#27669=CARTESIAN_POINT('Ctrl Pts',(-1.78852398877523,-1.,1.17305363177265));
#27670=CARTESIAN_POINT('Ctrl Pts',(-1.78852398877523,1.,1.17305363177265));
#27671=CARTESIAN_POINT('Ctrl Pts',(-1.79151291552646,-1.,1.17866429440781));
#27672=CARTESIAN_POINT('Ctrl Pts',(-1.79151291552646,1.,1.17866429440781));
#27673=CARTESIAN_POINT('Ctrl Pts',(-1.79447240321572,-1.,1.18430321697471));
#27674=CARTESIAN_POINT('Ctrl Pts',(-1.79447240321572,1.,1.18430321697471));
#27675=CARTESIAN_POINT('Ctrl Pts',(-1.79740245923649,-1.,1.1899699793456));
#27676=CARTESIAN_POINT('Ctrl Pts',(-1.79740245923649,1.,1.1899699793456));
#27677=CARTESIAN_POINT('Ctrl Pts',(-1.80030314370121,-1.,1.19566418930405));
#27678=CARTESIAN_POINT('Ctrl Pts',(-1.80030314370121,1.,1.19566418930405));
#27679=CARTESIAN_POINT('Ctrl Pts',(-1.8031745483882,-1.,1.2013854893912));
#27680=CARTESIAN_POINT('Ctrl Pts',(-1.8031745483882,1.,1.2013854893912));
#27681=CARTESIAN_POINT('Ctrl Pts',(-1.80601678480772,-1.,1.20713356605519));
#27682=CARTESIAN_POINT('Ctrl Pts',(-1.80601678480772,1.,1.20713356605519));
#27683=CARTESIAN_POINT('Ctrl Pts',(-1.80882996916931,-1.,1.2129081570818));
#27684=CARTESIAN_POINT('Ctrl Pts',(-1.80882996916931,1.,1.2129081570818));
#27685=CARTESIAN_POINT('Ctrl Pts',(-1.81161420806172,-1.,1.2187090610323));
#27686=CARTESIAN_POINT('Ctrl Pts',(-1.81161420806172,1.,1.2187090610323));
#27687=CARTESIAN_POINT('Ctrl Pts',(-1.81436959209778,-1.,1.22453613304507));
#27688=CARTESIAN_POINT('Ctrl Pts',(-1.81436959209778,1.,1.22453613304507));
#27689=CARTESIAN_POINT('Ctrl Pts',(-1.81655087183054,-1.,1.22921864890975));
#27690=CARTESIAN_POINT('Ctrl Pts',(-1.81655087183054,1.,1.22921864890975));
#27691=CARTESIAN_POINT('Ctrl Pts',(-1.81817389920914,-1.,1.23274224526804));
#27692=CARTESIAN_POINT('Ctrl Pts',(-1.81817389920914,1.,1.23274224526804));
#27693=CARTESIAN_POINT('Ctrl Pts',(-1.81925017193531,-1.,1.23509651170384));
#27694=CARTESIAN_POINT('Ctrl Pts',(-1.81925017193531,1.,1.23509651170384));
#27695=CARTESIAN_POINT('Ctrl Pts',(-1.81978687191668,-1.,1.23627494547115));
#27696=CARTESIAN_POINT('Ctrl Pts',(-1.81978687191668,1.,1.23627494547115));
#27697=CARTESIAN_POINT('',(-1.5055822144029,1.,0.892032620296855));
#27698=CARTESIAN_POINT('Ctrl Pts',(-1.5055822144029,1.,0.892032620296855));
#27699=CARTESIAN_POINT('Ctrl Pts',(-1.50980486807181,1.,0.894452006967538));
#27700=CARTESIAN_POINT('Ctrl Pts',(-1.51805569591479,1.,0.89918504749193));
#27701=CARTESIAN_POINT('Ctrl Pts',(-1.52984849890434,1.,0.905967409640499));
#27702=CARTESIAN_POINT('Ctrl Pts',(-1.54440491152808,1.,0.91437591904658));
#27703=CARTESIAN_POINT('Ctrl Pts',(-1.56065988582509,1.,0.923832188966322));
#27704=CARTESIAN_POINT('Ctrl Pts',(-1.57499388385561,1.,0.932246680128849));
#27705=CARTESIAN_POINT('Ctrl Pts',(-1.58744937489796,1.,0.939646377909319));
#27706=CARTESIAN_POINT('Ctrl Pts',(-1.59810042045408,1.,0.946078063325796));
#27707=CARTESIAN_POINT('Ctrl Pts',(-1.60706069897794,1.,0.951613284361248));
#27708=CARTESIAN_POINT('Ctrl Pts',(-1.61449324337233,1.,0.956354422921573));
#27709=CARTESIAN_POINT('Ctrl Pts',(-1.62061638139929,1.,0.960438326099958));
#27710=CARTESIAN_POINT('Ctrl Pts',(-1.6257193066974,1.,0.964046107037821));
#27711=CARTESIAN_POINT('Ctrl Pts',(-1.63013849959083,1.,0.967387853228041));
#27712=CARTESIAN_POINT('Ctrl Pts',(-1.63420665729609,1.,0.970669715996356));
#27713=CARTESIAN_POINT('Ctrl Pts',(-1.63820952658157,1.,0.974066058287501));
#27714=CARTESIAN_POINT('Ctrl Pts',(-1.64233990826831,1.,0.977689794120297));
#27715=CARTESIAN_POINT('Ctrl Pts',(-1.64665139190834,1.,0.981562530940574));
#27716=CARTESIAN_POINT('Ctrl Pts',(-1.6511001661277,1.,0.985642622921626));
#27717=CARTESIAN_POINT('Ctrl Pts',(-1.65559044289746,1.,0.98985562785445));
#27718=CARTESIAN_POINT('Ctrl Pts',(-1.66001553809916,1.,0.994121836661116));
#27719=CARTESIAN_POINT('Ctrl Pts',(-1.66430758030304,1.,0.998389654952317));
#27720=CARTESIAN_POINT('Ctrl Pts',(-1.66846059277231,1.,1.00265091003682));
#27721=CARTESIAN_POINT('Ctrl Pts',(-1.67250335383248,1.,1.00692206696387));
#27722=CARTESIAN_POINT('Ctrl Pts',(-1.67648246776457,1.,1.01123236493507));
#27723=CARTESIAN_POINT('Ctrl Pts',(-1.6804428989482,1.,1.01561026162787));
#27724=CARTESIAN_POINT('Ctrl Pts',(-1.68440578021739,1.,1.02006795074222));
#27725=CARTESIAN_POINT('Ctrl Pts',(-1.68836910178475,1.,1.02460180535272));
#27726=CARTESIAN_POINT('Ctrl Pts',(-1.69231840863471,1.,1.02919977579155));
#27727=CARTESIAN_POINT('Ctrl Pts',(-1.69623414782769,1.,1.03384646003587));
#27728=CARTESIAN_POINT('Ctrl Pts',(-1.70010052930951,1.,1.03852922490782));
#27729=CARTESIAN_POINT('Ctrl Pts',(-1.70391338707969,1.,1.04324363334546));
#27730=CARTESIAN_POINT('Ctrl Pts',(-1.70767646263641,1.,1.0479908540499));
#27731=CARTESIAN_POINT('Ctrl Pts',(-1.71139783543986,1.,1.05277517202854));
#27732=CARTESIAN_POINT('Ctrl Pts',(-1.71508654427022,1.,1.05760163192481));
#27733=CARTESIAN_POINT('Ctrl Pts',(-1.71874858456908,1.,1.0624732468065));
#27734=CARTESIAN_POINT('Ctrl Pts',(-1.72238500928456,1.,1.06738966975463));
#27735=CARTESIAN_POINT('Ctrl Pts',(-1.72599406198489,1.,1.07234866990252));
#27736=CARTESIAN_POINT('Ctrl Pts',(-1.72957248977424,1.,1.0773470373727));
#27737=CARTESIAN_POINT('Ctrl Pts',(-1.73311705663407,1.,1.08238162784749));
#27738=CARTESIAN_POINT('Ctrl Pts',(-1.73662628326093,1.,1.08745056285429));
#27739=CARTESIAN_POINT('Ctrl Pts',(-1.74010053962252,1.,1.09255329056496));
#27740=CARTESIAN_POINT('Ctrl Pts',(-1.74354119236212,1.,1.09768999241229));
#27741=CARTESIAN_POINT('Ctrl Pts',(-1.74695004214924,1.,1.10286118991144));
#27742=CARTESIAN_POINT('Ctrl Pts',(-1.75032866075914,1.,1.10806728183003));
#27743=CARTESIAN_POINT('Ctrl Pts',(-1.75367772094617,1.,1.11330807582542));
#27744=CARTESIAN_POINT('Ctrl Pts',(-1.75699720772089,1.,1.11858293216752));
#27745=CARTESIAN_POINT('Ctrl Pts',(-1.76028671825084,1.,1.12389096855078));
#27746=CARTESIAN_POINT('Ctrl Pts',(-1.76354571966171,1.,1.12923123555076));
#27747=CARTESIAN_POINT('Ctrl Pts',(-1.76677384551883,1.,1.13460291804635));
#27748=CARTESIAN_POINT('Ctrl Pts',(-1.76997111386806,1.,1.14000548337));
#27749=CARTESIAN_POINT('Ctrl Pts',(-1.77313777896234,1.,1.14543858226948));
#27750=CARTESIAN_POINT('Ctrl Pts',(-1.77627422557034,1.,1.15090197841531));
#27751=CARTESIAN_POINT('Ctrl Pts',(-1.77938085564261,1.,1.15639547194689));
#27752=CARTESIAN_POINT('Ctrl Pts',(-1.78245795880949,1.,1.16191881298458));
#27753=CARTESIAN_POINT('Ctrl Pts',(-1.78550566040349,1.,1.16747166312239));
#27754=CARTESIAN_POINT('Ctrl Pts',(-1.78852398877523,1.,1.17305363177265));
#27755=CARTESIAN_POINT('Ctrl Pts',(-1.79151291552646,1.,1.17866429440781));
#27756=CARTESIAN_POINT('Ctrl Pts',(-1.79447240321572,1.,1.18430321697471));
#27757=CARTESIAN_POINT('Ctrl Pts',(-1.79740245923649,1.,1.1899699793456));
#27758=CARTESIAN_POINT('Ctrl Pts',(-1.80030314370121,1.,1.19566418930405));
#27759=CARTESIAN_POINT('Ctrl Pts',(-1.8031745483882,1.,1.2013854893912));
#27760=CARTESIAN_POINT('Ctrl Pts',(-1.80601678480772,1.,1.20713356605519));
#27761=CARTESIAN_POINT('Ctrl Pts',(-1.80882996916931,1.,1.2129081570818));
#27762=CARTESIAN_POINT('Ctrl Pts',(-1.81161420806172,1.,1.2187090610323));
#27763=CARTESIAN_POINT('Ctrl Pts',(-1.81436959209778,1.,1.22453613304507));
#27764=CARTESIAN_POINT('Ctrl Pts',(-1.81655087183054,1.,1.22921864890975));
#27765=CARTESIAN_POINT('Ctrl Pts',(-1.81817389920914,1.,1.23274224526804));
#27766=CARTESIAN_POINT('Ctrl Pts',(-1.81925017193531,1.,1.23509651170384));
#27767=CARTESIAN_POINT('Ctrl Pts',(-1.81978687191668,1.,1.23627494547115));
#27768=CARTESIAN_POINT('',(-1.5055822144029,0.,0.892032620296856));
#27769=CARTESIAN_POINT('Origin',(0.,0.,0.));
#27770=CARTESIAN_POINT('',(-1.60662857109684,1.,0.693717979106305));
#27771=CARTESIAN_POINT('Origin',(0.,1.,0.));
#27772=CARTESIAN_POINT('',(-1.60662857109684,0.,0.693717979106306));
#27773=CARTESIAN_POINT('Ctrl Pts',(-2.0698113262342,-1.,0.7455743247944));
#27774=CARTESIAN_POINT('Ctrl Pts',(-2.0698113262342,1.,0.7455743247944));
#27775=CARTESIAN_POINT('Ctrl Pts',(-2.06854248895728,-1.,0.745832791378367));
#27776=CARTESIAN_POINT('Ctrl Pts',(-2.06854248895728,1.,0.745832791378367));
#27777=CARTESIAN_POINT('Ctrl Pts',(-2.06600523016815,-1.,0.7463458715442));
#27778=CARTESIAN_POINT('Ctrl Pts',(-2.06600523016815,1.,0.7463458715442));
#27779=CARTESIAN_POINT('Ctrl Pts',(-2.06220058927826,-1.,0.747103932787919));
#27780=CARTESIAN_POINT('Ctrl Pts',(-2.06220058927826,1.,0.747103932787919));
#27781=CARTESIAN_POINT('Ctrl Pts',(-2.05713023031006,-1.,0.748091554183802));
#27782=CARTESIAN_POINT('Ctrl Pts',(-2.05713023031006,1.,0.748091554183802));
#27783=CARTESIAN_POINT('Ctrl Pts',(-2.05079645592154,-1.,0.749287468665046));
#27784=CARTESIAN_POINT('Ctrl Pts',(-2.05079645592154,1.,0.749287468665046));
#27785=CARTESIAN_POINT('Ctrl Pts',(-2.04446689147979,-1.,0.750444657875576));
#27786=CARTESIAN_POINT('Ctrl Pts',(-2.04446689147979,1.,0.750444657875576));
#27787=CARTESIAN_POINT('Ctrl Pts',(-2.03814160092099,-1.,0.751562963361115));
#27788=CARTESIAN_POINT('Ctrl Pts',(-2.03814160092099,1.,0.751562963361115));
#27789=CARTESIAN_POINT('Ctrl Pts',(-2.03182068456221,-1.,0.752642180487211));
#27790=CARTESIAN_POINT('Ctrl Pts',(-2.03182068456221,1.,0.752642180487211));
#27791=CARTESIAN_POINT('Ctrl Pts',(-2.02550428623313,-1.,0.753682061112768));
#27792=CARTESIAN_POINT('Ctrl Pts',(-2.02550428623313,1.,0.753682061112768));
#27793=CARTESIAN_POINT('Ctrl Pts',(-2.01919259405809,-1.,0.754682330722816));
#27794=CARTESIAN_POINT('Ctrl Pts',(-2.01919259405809,1.,0.754682330722816));
#27795=CARTESIAN_POINT('Ctrl Pts',(-2.01288584328084,-1.,0.755642704957865));
#27796=CARTESIAN_POINT('Ctrl Pts',(-2.01288584328084,1.,0.755642704957865));
#27797=CARTESIAN_POINT('Ctrl Pts',(-2.0065843158773,-1.,0.75656290464667));
#27798=CARTESIAN_POINT('Ctrl Pts',(-2.0065843158773,1.,0.75656290464667));
#27799=CARTESIAN_POINT('Ctrl Pts',(-2.00028834739178,-1.,0.757442676862724));
#27800=CARTESIAN_POINT('Ctrl Pts',(-2.00028834739178,1.,0.757442676862724));
#27801=CARTESIAN_POINT('Ctrl Pts',(-1.99399831098817,-1.,0.758281796766761));
#27802=CARTESIAN_POINT('Ctrl Pts',(-1.99399831098817,1.,0.758281796766761));
#27803=CARTESIAN_POINT('Ctrl Pts',(-1.98771456680874,-1.,0.759080037802488));
#27804=CARTESIAN_POINT('Ctrl Pts',(-1.98771456680874,1.,0.759080037802488));
#27805=CARTESIAN_POINT('Ctrl Pts',(-1.98143741418172,-1.,0.75983714745219));
#27806=CARTESIAN_POINT('Ctrl Pts',(-1.98143741418172,1.,0.75983714745219));
#27807=CARTESIAN_POINT('Ctrl Pts',(-1.97516705321494,-1.,0.760552825409757));
#27808=CARTESIAN_POINT('Ctrl Pts',(-1.97516705321494,1.,0.760552825409757));
#27809=CARTESIAN_POINT('Ctrl Pts',(-1.96890351582499,-1.,0.76122669048382));
#27810=CARTESIAN_POINT('Ctrl Pts',(-1.96890351582499,1.,0.76122669048382));
#27811=CARTESIAN_POINT('Ctrl Pts',(-1.96264672744186,-1.,0.761858300014423));
#27812=CARTESIAN_POINT('Ctrl Pts',(-1.96264672744186,1.,0.761858300014423));
#27813=CARTESIAN_POINT('Ctrl Pts',(-1.95639665309869,-1.,0.762447203806179));
#27814=CARTESIAN_POINT('Ctrl Pts',(-1.95639665309869,1.,0.762447203806179));
#27815=CARTESIAN_POINT('Ctrl Pts',(-1.95015342590024,-1.,0.762992990878769));
#27816=CARTESIAN_POINT('Ctrl Pts',(-1.95015342590024,1.,0.762992990878769));
#27817=CARTESIAN_POINT('Ctrl Pts',(-1.9439174661764,-1.,0.763495333538629));
#27818=CARTESIAN_POINT('Ctrl Pts',(-1.9439174661764,1.,0.763495333538629));
#27819=CARTESIAN_POINT('Ctrl Pts',(-1.93768964875886,-1.,0.763954049121458));
#27820=CARTESIAN_POINT('Ctrl Pts',(-1.93768964875886,1.,0.763954049121458));
#27821=CARTESIAN_POINT('Ctrl Pts',(-1.93147105496382,-1.,0.76436901067394));
#27822=CARTESIAN_POINT('Ctrl Pts',(-1.93147105496382,1.,0.76436901067394));
#27823=CARTESIAN_POINT('Ctrl Pts',(-1.92526263537048,-1.,0.764740025488211));
#27824=CARTESIAN_POINT('Ctrl Pts',(-1.92526263537048,1.,0.764740025488211));
#27825=CARTESIAN_POINT('Ctrl Pts',(-1.91906491634196,-1.,0.765066729667088));
#27826=CARTESIAN_POINT('Ctrl Pts',(-1.91906491634196,1.,0.765066729667088));
#27827=CARTESIAN_POINT('Ctrl Pts',(-1.91287765805169,-1.,0.765348465884722));
#27828=CARTESIAN_POINT('Ctrl Pts',(-1.91287765805169,1.,0.765348465884722));
#27829=CARTESIAN_POINT('Ctrl Pts',(-1.90669961402356,-1.,0.765584196937919));
#27830=CARTESIAN_POINT('Ctrl Pts',(-1.90669961402356,1.,0.765584196937919));
#27831=CARTESIAN_POINT('Ctrl Pts',(-1.90052930393596,-1.,0.765772772593386));
#27832=CARTESIAN_POINT('Ctrl Pts',(-1.90052930393596,1.,0.765772772593386));
#27833=CARTESIAN_POINT('Ctrl Pts',(-1.89436577771388,-1.,0.765913193856978));
#27834=CARTESIAN_POINT('Ctrl Pts',(-1.89436577771388,1.,0.765913193856978));
#27835=CARTESIAN_POINT('Ctrl Pts',(-1.88820926433409,-1.,0.766004837062091));
#27836=CARTESIAN_POINT('Ctrl Pts',(-1.88820926433409,1.,0.766004837062091));
#27837=CARTESIAN_POINT('Ctrl Pts',(-1.88206215302561,-1.,0.766047794851864));
#27838=CARTESIAN_POINT('Ctrl Pts',(-1.88206215302561,1.,0.766047794851864));
#27839=CARTESIAN_POINT('Ctrl Pts',(-1.87592888967883,-1.,0.766042837036744));
#27840=CARTESIAN_POINT('Ctrl Pts',(-1.87592888967883,1.,0.766042837036744));
#27841=CARTESIAN_POINT('Ctrl Pts',(-1.86981398314341,-1.,0.765990708546091));
#27842=CARTESIAN_POINT('Ctrl Pts',(-1.86981398314341,1.,0.765990708546091));
#27843=CARTESIAN_POINT('Ctrl Pts',(-1.86372027063312,-1.,0.765891519092547));
#27844=CARTESIAN_POINT('Ctrl Pts',(-1.86372027063312,1.,0.765891519092547));
#27845=CARTESIAN_POINT('Ctrl Pts',(-1.85764741390394,-1.,0.765744212909318));
#27846=CARTESIAN_POINT('Ctrl Pts',(-1.85764741390394,1.,0.765744212909318));
#27847=CARTESIAN_POINT('Ctrl Pts',(-1.85158945130063,-1.,0.765545710619062));
#27848=CARTESIAN_POINT('Ctrl Pts',(-1.85158945130063,1.,0.765545710619062));
#27849=CARTESIAN_POINT('Ctrl Pts',(-1.84553698875924,-1.,0.765291664862029));
#27850=CARTESIAN_POINT('Ctrl Pts',(-1.84553698875924,1.,0.765291664862029));
#27851=CARTESIAN_POINT('Ctrl Pts',(-1.83948181064835,-1.,0.764978057881737));
#27852=CARTESIAN_POINT('Ctrl Pts',(-1.83948181064835,1.,0.764978057881737));
#27853=CARTESIAN_POINT('Ctrl Pts',(-1.83342077227142,-1.,0.764602549687853));
#27854=CARTESIAN_POINT('Ctrl Pts',(-1.83342077227142,1.,0.764602549687853));
#27855=CARTESIAN_POINT('Ctrl Pts',(-1.82735991200065,-1.,0.764165902605995));
#27856=CARTESIAN_POINT('Ctrl Pts',(-1.82735991200065,1.,0.764165902605995));
#27857=CARTESIAN_POINT('Ctrl Pts',(-1.82131873145266,-1.,0.763673465462726));
#27858=CARTESIAN_POINT('Ctrl Pts',(-1.82131873145266,1.,0.763673465462726));
#27859=CARTESIAN_POINT('Ctrl Pts',(-1.8153211840553,-1.,0.763132003836634));
#27860=CARTESIAN_POINT('Ctrl Pts',(-1.8153211840553,1.,0.763132003836634));
#27861=CARTESIAN_POINT('Ctrl Pts',(-1.80938551463965,-1.,0.762546129463938));
#27862=CARTESIAN_POINT('Ctrl Pts',(-1.80938551463965,1.,0.762546129463938));
#27863=CARTESIAN_POINT('Ctrl Pts',(-1.80351583877342,-1.,0.761915336443547));
#27864=CARTESIAN_POINT('Ctrl Pts',(-1.80351583877342,1.,0.761915336443547));
#27865=CARTESIAN_POINT('Ctrl Pts',(-1.79768986997783,-1.,0.761229695230558));
#27866=CARTESIAN_POINT('Ctrl Pts',(-1.79768986997783,1.,0.761229695230558));
#27867=CARTESIAN_POINT('Ctrl Pts',(-1.7918581561088,-1.,0.760469555880749));
#27868=CARTESIAN_POINT('Ctrl Pts',(-1.7918581561088,1.,0.760469555880749));
#27869=CARTESIAN_POINT('Ctrl Pts',(-1.78596964884604,-1.,0.759614401110189));
#27870=CARTESIAN_POINT('Ctrl Pts',(-1.78596964884604,1.,0.759614401110189));
#27871=CARTESIAN_POINT('Ctrl Pts',(-1.77999411220945,-1.,0.758650626677518));
#27872=CARTESIAN_POINT('Ctrl Pts',(-1.77999411220945,1.,0.758650626677518));
#27873=CARTESIAN_POINT('Ctrl Pts',(-1.77394167108292,-1.,0.757578264077029));
#27874=CARTESIAN_POINT('Ctrl Pts',(-1.77394167108292,1.,0.757578264077029));
#27875=CARTESIAN_POINT('Ctrl Pts',(-1.76789396002998,-1.,0.75642189602781));
#27876=CARTESIAN_POINT('Ctrl Pts',(-1.76789396002998,1.,0.75642189602781));
#27877=CARTESIAN_POINT('Ctrl Pts',(-1.76197817240128,-1.,0.755220979974461));
#27878=CARTESIAN_POINT('Ctrl Pts',(-1.76197817240128,1.,0.755220979974461));
#27879=CARTESIAN_POINT('Ctrl Pts',(-1.75631083600019,-1.,0.754009254027829));
#27880=CARTESIAN_POINT('Ctrl Pts',(-1.75631083600019,1.,0.754009254027829));
#27881=CARTESIAN_POINT('Ctrl Pts',(-1.75095139468794,-1.,0.752797683531314));
#27882=CARTESIAN_POINT('Ctrl Pts',(-1.75095139468794,1.,0.752797683531314));
#27883=CARTESIAN_POINT('Ctrl Pts',(-1.74585086852502,-1.,0.751555614164482));
#27884=CARTESIAN_POINT('Ctrl Pts',(-1.74585086852502,1.,0.751555614164482));
#27885=CARTESIAN_POINT('Ctrl Pts',(-1.74080458267114,-1.,0.750193435981249));
#27886=CARTESIAN_POINT('Ctrl Pts',(-1.74080458267114,1.,0.750193435981249));
#27887=CARTESIAN_POINT('Ctrl Pts',(-1.7355035168033,-1.,0.74858246295687));
#27888=CARTESIAN_POINT('Ctrl Pts',(-1.7355035168033,1.,0.74858246295687));
#27889=CARTESIAN_POINT('Ctrl Pts',(-1.72958533647714,-1.,0.746574710097752));
#27890=CARTESIAN_POINT('Ctrl Pts',(-1.72958533647714,1.,0.746574710097752));
#27891=CARTESIAN_POINT('Ctrl Pts',(-1.72268229916769,-1.,0.744021445433093));
#27892=CARTESIAN_POINT('Ctrl Pts',(-1.72268229916769,1.,0.744021445433093));
#27893=CARTESIAN_POINT('Ctrl Pts',(-1.71447789751001,-1.,0.74079516202821));
#27894=CARTESIAN_POINT('Ctrl Pts',(-1.71447789751001,1.,0.74079516202821));
#27895=CARTESIAN_POINT('Ctrl Pts',(-1.70473309004249,-1.,0.736799665716932));
#27896=CARTESIAN_POINT('Ctrl Pts',(-1.70473309004249,1.,0.736799665716932));
#27897=CARTESIAN_POINT('Ctrl Pts',(-1.69326921972915,-1.,0.731963238685357));
#27898=CARTESIAN_POINT('Ctrl Pts',(-1.69326921972915,1.,0.731963238685357));
#27899=CARTESIAN_POINT('Ctrl Pts',(-1.67996158451922,-1.,0.726235967982445));
#27900=CARTESIAN_POINT('Ctrl Pts',(-1.67996158451922,1.,0.726235967982445));
#27901=CARTESIAN_POINT('Ctrl Pts',(-1.66472880551777,-1.,0.71958543378795));
#27902=CARTESIAN_POINT('Ctrl Pts',(-1.66472880551777,1.,0.71958543378795));
#27903=CARTESIAN_POINT('Ctrl Pts',(-1.64752408828442,-1.,0.711993139340447));
#27904=CARTESIAN_POINT('Ctrl Pts',(-1.64752408828442,1.,0.711993139340447));
#27905=CARTESIAN_POINT('Ctrl Pts',(-1.6321654166204,-1.,0.705159151977294));
#27906=CARTESIAN_POINT('Ctrl Pts',(-1.6321654166204,1.,0.705159151977294));
#27907=CARTESIAN_POINT('Ctrl Pts',(-1.61974673471117,-1.,0.699605146398837));
#27908=CARTESIAN_POINT('Ctrl Pts',(-1.61974673471117,1.,0.699605146398837));
#27909=CARTESIAN_POINT('Ctrl Pts',(-1.61106790957619,-1.,0.69571209787897));
#27910=CARTESIAN_POINT('Ctrl Pts',(-1.61106790957619,1.,0.69571209787897));
#27911=CARTESIAN_POINT('Ctrl Pts',(-1.60662857109684,-1.,0.693717979106305));
#27912=CARTESIAN_POINT('Ctrl Pts',(-1.60662857109684,1.,0.693717979106305));
#27913=CARTESIAN_POINT('',(-2.0698113262342,1.,0.7455743247944));
#27914=CARTESIAN_POINT('Ctrl Pts',(-2.0698113262342,1.,0.7455743247944));
#27915=CARTESIAN_POINT('Ctrl Pts',(-2.06854248895728,1.,0.745832791378367));
#27916=CARTESIAN_POINT('Ctrl Pts',(-2.06600523016815,1.,0.7463458715442));
#27917=CARTESIAN_POINT('Ctrl Pts',(-2.06220058927826,1.,0.747103932787919));
#27918=CARTESIAN_POINT('Ctrl Pts',(-2.05713023031006,1.,0.748091554183802));
#27919=CARTESIAN_POINT('Ctrl Pts',(-2.05079645592154,1.,0.749287468665046));
#27920=CARTESIAN_POINT('Ctrl Pts',(-2.04446689147979,1.,0.750444657875576));
#27921=CARTESIAN_POINT('Ctrl Pts',(-2.03814160092099,1.,0.751562963361115));
#27922=CARTESIAN_POINT('Ctrl Pts',(-2.03182068456221,1.,0.752642180487211));
#27923=CARTESIAN_POINT('Ctrl Pts',(-2.02550428623313,1.,0.753682061112768));
#27924=CARTESIAN_POINT('Ctrl Pts',(-2.01919259405809,1.,0.754682330722816));
#27925=CARTESIAN_POINT('Ctrl Pts',(-2.01288584328084,1.,0.755642704957865));
#27926=CARTESIAN_POINT('Ctrl Pts',(-2.0065843158773,1.,0.75656290464667));
#27927=CARTESIAN_POINT('Ctrl Pts',(-2.00028834739178,1.,0.757442676862724));
#27928=CARTESIAN_POINT('Ctrl Pts',(-1.99399831098817,1.,0.758281796766761));
#27929=CARTESIAN_POINT('Ctrl Pts',(-1.98771456680874,1.,0.759080037802488));
#27930=CARTESIAN_POINT('Ctrl Pts',(-1.98143741418172,1.,0.75983714745219));
#27931=CARTESIAN_POINT('Ctrl Pts',(-1.97516705321494,1.,0.760552825409757));
#27932=CARTESIAN_POINT('Ctrl Pts',(-1.96890351582499,1.,0.76122669048382));
#27933=CARTESIAN_POINT('Ctrl Pts',(-1.96264672744186,1.,0.761858300014423));
#27934=CARTESIAN_POINT('Ctrl Pts',(-1.95639665309869,1.,0.762447203806179));
#27935=CARTESIAN_POINT('Ctrl Pts',(-1.95015342590024,1.,0.762992990878769));
#27936=CARTESIAN_POINT('Ctrl Pts',(-1.9439174661764,1.,0.763495333538629));
#27937=CARTESIAN_POINT('Ctrl Pts',(-1.93768964875886,1.,0.763954049121458));
#27938=CARTESIAN_POINT('Ctrl Pts',(-1.93147105496382,1.,0.76436901067394));
#27939=CARTESIAN_POINT('Ctrl Pts',(-1.92526263537048,1.,0.764740025488211));
#27940=CARTESIAN_POINT('Ctrl Pts',(-1.91906491634196,1.,0.765066729667088));
#27941=CARTESIAN_POINT('Ctrl Pts',(-1.91287765805169,1.,0.765348465884722));
#27942=CARTESIAN_POINT('Ctrl Pts',(-1.90669961402356,1.,0.765584196937919));
#27943=CARTESIAN_POINT('Ctrl Pts',(-1.90052930393596,1.,0.765772772593386));
#27944=CARTESIAN_POINT('Ctrl Pts',(-1.89436577771388,1.,0.765913193856978));
#27945=CARTESIAN_POINT('Ctrl Pts',(-1.88820926433409,1.,0.766004837062091));
#27946=CARTESIAN_POINT('Ctrl Pts',(-1.88206215302561,1.,0.766047794851864));
#27947=CARTESIAN_POINT('Ctrl Pts',(-1.87592888967883,1.,0.766042837036744));
#27948=CARTESIAN_POINT('Ctrl Pts',(-1.86981398314341,1.,0.765990708546091));
#27949=CARTESIAN_POINT('Ctrl Pts',(-1.86372027063312,1.,0.765891519092547));
#27950=CARTESIAN_POINT('Ctrl Pts',(-1.85764741390394,1.,0.765744212909318));
#27951=CARTESIAN_POINT('Ctrl Pts',(-1.85158945130063,1.,0.765545710619062));
#27952=CARTESIAN_POINT('Ctrl Pts',(-1.84553698875924,1.,0.765291664862029));
#27953=CARTESIAN_POINT('Ctrl Pts',(-1.83948181064835,1.,0.764978057881737));
#27954=CARTESIAN_POINT('Ctrl Pts',(-1.83342077227142,1.,0.764602549687853));
#27955=CARTESIAN_POINT('Ctrl Pts',(-1.82735991200065,1.,0.764165902605995));
#27956=CARTESIAN_POINT('Ctrl Pts',(-1.82131873145266,1.,0.763673465462726));
#27957=CARTESIAN_POINT('Ctrl Pts',(-1.8153211840553,1.,0.763132003836634));
#27958=CARTESIAN_POINT('Ctrl Pts',(-1.80938551463965,1.,0.762546129463938));
#27959=CARTESIAN_POINT('Ctrl Pts',(-1.80351583877342,1.,0.761915336443547));
#27960=CARTESIAN_POINT('Ctrl Pts',(-1.79768986997783,1.,0.761229695230558));
#27961=CARTESIAN_POINT('Ctrl Pts',(-1.7918581561088,1.,0.760469555880749));
#27962=CARTESIAN_POINT('Ctrl Pts',(-1.78596964884604,1.,0.759614401110189));
#27963=CARTESIAN_POINT('Ctrl Pts',(-1.77999411220945,1.,0.758650626677518));
#27964=CARTESIAN_POINT('Ctrl Pts',(-1.77394167108292,1.,0.757578264077029));
#27965=CARTESIAN_POINT('Ctrl Pts',(-1.76789396002998,1.,0.75642189602781));
#27966=CARTESIAN_POINT('Ctrl Pts',(-1.76197817240128,1.,0.755220979974461));
#27967=CARTESIAN_POINT('Ctrl Pts',(-1.75631083600019,1.,0.754009254027829));
#27968=CARTESIAN_POINT('Ctrl Pts',(-1.75095139468794,1.,0.752797683531314));
#27969=CARTESIAN_POINT('Ctrl Pts',(-1.74585086852502,1.,0.751555614164482));
#27970=CARTESIAN_POINT('Ctrl Pts',(-1.74080458267114,1.,0.750193435981249));
#27971=CARTESIAN_POINT('Ctrl Pts',(-1.7355035168033,1.,0.74858246295687));
#27972=CARTESIAN_POINT('Ctrl Pts',(-1.72958533647714,1.,0.746574710097752));
#27973=CARTESIAN_POINT('Ctrl Pts',(-1.72268229916769,1.,0.744021445433093));
#27974=CARTESIAN_POINT('Ctrl Pts',(-1.71447789751001,1.,0.74079516202821));
#27975=CARTESIAN_POINT('Ctrl Pts',(-1.70473309004249,1.,0.736799665716932));
#27976=CARTESIAN_POINT('Ctrl Pts',(-1.69326921972915,1.,0.731963238685357));
#27977=CARTESIAN_POINT('Ctrl Pts',(-1.67996158451922,1.,0.726235967982445));
#27978=CARTESIAN_POINT('Ctrl Pts',(-1.66472880551777,1.,0.71958543378795));
#27979=CARTESIAN_POINT('Ctrl Pts',(-1.64752408828442,1.,0.711993139340447));
#27980=CARTESIAN_POINT('Ctrl Pts',(-1.6321654166204,1.,0.705159151977294));
#27981=CARTESIAN_POINT('Ctrl Pts',(-1.61974673471117,1.,0.699605146398837));
#27982=CARTESIAN_POINT('Ctrl Pts',(-1.61106790957619,1.,0.69571209787897));
#27983=CARTESIAN_POINT('Ctrl Pts',(-1.60662857109684,1.,0.693717979106305));
#27984=CARTESIAN_POINT('',(-2.0698113262342,0.,0.7455743247944));
#27985=CARTESIAN_POINT('Origin',(-2.11275013067528,0.,0.61342227326009));
#27986=CARTESIAN_POINT('',(-2.11275013067528,1.,0.61342227326009));
#27987=CARTESIAN_POINT('',(-2.0698113262342,1.,0.7455743247944));
#27988=CARTESIAN_POINT('',(-2.11275013067528,0.,0.61342227326009));
#27989=CARTESIAN_POINT('Ctrl Pts',(-1.7075470150345,-1.,0.383122945602004));
#27990=CARTESIAN_POINT('Ctrl Pts',(-1.7075470150345,1.,0.383122945602004));
#27991=CARTESIAN_POINT('Ctrl Pts',(-1.71231062891958,-1.,0.384119047315542));
#27992=CARTESIAN_POINT('Ctrl Pts',(-1.71231062891958,1.,0.384119047315542));
#27993=CARTESIAN_POINT('Ctrl Pts',(-1.72162022246158,-1.,0.38607079032701));
#27994=CARTESIAN_POINT('Ctrl Pts',(-1.72162022246158,1.,0.38607079032701));
#27995=CARTESIAN_POINT('Ctrl Pts',(-1.7349317097561,-1.,0.388877023509191));
#27996=CARTESIAN_POINT('Ctrl Pts',(-1.7349317097561,1.,0.388877023509191));
#27997=CARTESIAN_POINT('Ctrl Pts',(-1.75137405313962,-1.,0.392375812294307));
#27998=CARTESIAN_POINT('Ctrl Pts',(-1.75137405313962,1.,0.392375812294307));
#27999=CARTESIAN_POINT('Ctrl Pts',(-1.7697556004756,-1.,0.39634619612042));
#28000=CARTESIAN_POINT('Ctrl Pts',(-1.7697556004756,1.,0.39634619612042));
#28001=CARTESIAN_POINT('Ctrl Pts',(-1.78598826347533,-1.,0.39991940378308));
#28002=CARTESIAN_POINT('Ctrl Pts',(-1.78598826347533,1.,0.39991940378308));
#28003=CARTESIAN_POINT('Ctrl Pts',(-1.80012077176221,-1.,0.403107976170441));
#28004=CARTESIAN_POINT('Ctrl Pts',(-1.80012077176221,1.,0.403107976170441));
#28005=CARTESIAN_POINT('Ctrl Pts',(-1.81223801813988,-1.,0.405933518411838));
#28006=CARTESIAN_POINT('Ctrl Pts',(-1.81223801813988,1.,0.405933518411838));
#28007=CARTESIAN_POINT('Ctrl Pts',(-1.8224702267854,-1.,0.408428948108533));
#28008=CARTESIAN_POINT('Ctrl Pts',(-1.8224702267854,1.,0.408428948108533));
#28009=CARTESIAN_POINT('Ctrl Pts',(-1.83100408895216,-1.,0.410641256301675));
#28010=CARTESIAN_POINT('Ctrl Pts',(-1.83100408895216,1.,0.410641256301675));
#28011=CARTESIAN_POINT('Ctrl Pts',(-1.83808953475839,-1.,0.412633125322161));
#28012=CARTESIAN_POINT('Ctrl Pts',(-1.83808953475839,1.,0.412633125322161));
#28013=CARTESIAN_POINT('Ctrl Pts',(-1.8440575707371,-1.,0.41448743825434));
#28014=CARTESIAN_POINT('Ctrl Pts',(-1.8440575707371,1.,0.41448743825434));
#28015=CARTESIAN_POINT('Ctrl Pts',(-1.84929312929882,-1.,0.416300022038864));
#28016=CARTESIAN_POINT('Ctrl Pts',(-1.84929312929882,1.,0.416300022038864));
#28017=CARTESIAN_POINT('Ctrl Pts',(-1.85417632856234,-1.,0.418164129143534));
#28018=CARTESIAN_POINT('Ctrl Pts',(-1.85417632856234,1.,0.418164129143534));
#28019=CARTESIAN_POINT('Ctrl Pts',(-1.85903281096686,-1.,0.420157287975619));
#28020=CARTESIAN_POINT('Ctrl Pts',(-1.85903281096686,1.,0.420157287975619));
#28021=CARTESIAN_POINT('Ctrl Pts',(-1.86408083334028,-1.,0.422327307418275));
#28022=CARTESIAN_POINT('Ctrl Pts',(-1.86408083334028,1.,0.422327307418275));
#28023=CARTESIAN_POINT('Ctrl Pts',(-1.86937803944323,-1.,0.424678177291359));
#28024=CARTESIAN_POINT('Ctrl Pts',(-1.86937803944323,1.,0.424678177291359));
#28025=CARTESIAN_POINT('Ctrl Pts',(-1.87486989291484,-1.,0.427183828519102));
#28026=CARTESIAN_POINT('Ctrl Pts',(-1.87486989291484,1.,0.427183828519102));
#28027=CARTESIAN_POINT('Ctrl Pts',(-1.88044229001832,-1.,0.429803062482344));
#28028=CARTESIAN_POINT('Ctrl Pts',(-1.88044229001832,1.,0.429803062482344));
#28029=CARTESIAN_POINT('Ctrl Pts',(-1.88596913666793,-1.,0.432493038548748));
#28030=CARTESIAN_POINT('Ctrl Pts',(-1.88596913666793,1.,0.432493038548748));
#28031=CARTESIAN_POINT('Ctrl Pts',(-1.89136993975504,-1.,0.435225660963383));
#28032=CARTESIAN_POINT('Ctrl Pts',(-1.89136993975504,1.,0.435225660963383));
#28033=CARTESIAN_POINT('Ctrl Pts',(-1.89663648956466,-1.,0.437995003948244));
#28034=CARTESIAN_POINT('Ctrl Pts',(-1.89663648956466,1.,0.437995003948244));
#28035=CARTESIAN_POINT('Ctrl Pts',(-1.90180124389086,-1.,0.440807833704038));
#28036=CARTESIAN_POINT('Ctrl Pts',(-1.90180124389086,1.,0.440807833704038));
#28037=CARTESIAN_POINT('Ctrl Pts',(-1.90691756144898,-1.,0.44367755684915));
#28038=CARTESIAN_POINT('Ctrl Pts',(-1.90691756144898,1.,0.44367755684915));
#28039=CARTESIAN_POINT('Ctrl Pts',(-1.9120369998112,-1.,0.446617343485711));
#28040=CARTESIAN_POINT('Ctrl Pts',(-1.9120369998112,1.,0.446617343485711));
#28041=CARTESIAN_POINT('Ctrl Pts',(-1.91718342555755,-1.,0.449632260106662));
#28042=CARTESIAN_POINT('Ctrl Pts',(-1.91718342555755,1.,0.449632260106662));
#28043=CARTESIAN_POINT('Ctrl Pts',(-1.92235380648502,-1.,0.452719478359432));
#28044=CARTESIAN_POINT('Ctrl Pts',(-1.92235380648502,1.,0.452719478359432));
#28045=CARTESIAN_POINT('Ctrl Pts',(-1.92753067150476,-1.,0.455872005174371));
#28046=CARTESIAN_POINT('Ctrl Pts',(-1.92753067150476,1.,0.455872005174371));
#28047=CARTESIAN_POINT('Ctrl Pts',(-1.93269066517934,-1.,0.459081234547926));
#28048=CARTESIAN_POINT('Ctrl Pts',(-1.93269066517934,1.,0.459081234547926));
#28049=CARTESIAN_POINT('Ctrl Pts',(-1.93781486640821,-1.,0.462340031009056));
#28050=CARTESIAN_POINT('Ctrl Pts',(-1.93781486640821,1.,0.462340031009056));
#28051=CARTESIAN_POINT('Ctrl Pts',(-1.9428979419619,-1.,0.46564546202603));
#28052=CARTESIAN_POINT('Ctrl Pts',(-1.9428979419619,1.,0.46564546202603));
#28053=CARTESIAN_POINT('Ctrl Pts',(-1.94794381136514,-1.,0.468997482913135));
#28054=CARTESIAN_POINT('Ctrl Pts',(-1.94794381136514,1.,0.468997482913135));
#28055=CARTESIAN_POINT('Ctrl Pts',(-1.95296148278133,-1.,0.472397672264072));
#28056=CARTESIAN_POINT('Ctrl Pts',(-1.95296148278133,1.,0.472397672264072));
#28057=CARTESIAN_POINT('Ctrl Pts',(-1.95796111148177,-1.,0.475848034683176));
#28058=CARTESIAN_POINT('Ctrl Pts',(-1.95796111148177,1.,0.475848034683176));
#28059=CARTESIAN_POINT('Ctrl Pts',(-1.96294933055943,-1.,0.479349583074855));
#28060=CARTESIAN_POINT('Ctrl Pts',(-1.96294933055943,1.,0.479349583074855));
#28061=CARTESIAN_POINT('Ctrl Pts',(-1.96792703422362,-1.,0.48290166212069));
#28062=CARTESIAN_POINT('Ctrl Pts',(-1.96792703422362,1.,0.48290166212069));
#28063=CARTESIAN_POINT('Ctrl Pts',(-1.97289186263272,-1.,0.486502692907659));
#28064=CARTESIAN_POINT('Ctrl Pts',(-1.97289186263272,1.,0.486502692907659));
#28065=CARTESIAN_POINT('Ctrl Pts',(-1.97783973019229,-1.,0.490150627860952));
#28066=CARTESIAN_POINT('Ctrl Pts',(-1.97783973019229,1.,0.490150627860952));
#28067=CARTESIAN_POINT('Ctrl Pts',(-1.98276658761821,-1.,0.493843476541494));
#28068=CARTESIAN_POINT('Ctrl Pts',(-1.98276658761821,1.,0.493843476541494));
#28069=CARTESIAN_POINT('Ctrl Pts',(-1.98767044752932,-1.,0.497579909545574));
#28070=CARTESIAN_POINT('Ctrl Pts',(-1.98767044752932,1.,0.497579909545574));
#28071=CARTESIAN_POINT('Ctrl Pts',(-1.99255149126155,-1.,0.501359287727146));
#28072=CARTESIAN_POINT('Ctrl Pts',(-1.99255149126155,1.,0.501359287727146));
#28073=CARTESIAN_POINT('Ctrl Pts',(-1.99741107463572,-1.,0.505181361323026));
#28074=CARTESIAN_POINT('Ctrl Pts',(-1.99741107463572,1.,0.505181361323026));
#28075=CARTESIAN_POINT('Ctrl Pts',(-2.00225107134734,-1.,0.509046069886157));
#28076=CARTESIAN_POINT('Ctrl Pts',(-2.00225107134734,1.,0.509046069886157));
#28077=CARTESIAN_POINT('Ctrl Pts',(-2.00707309946949,-1.,0.512953306961792));
#28078=CARTESIAN_POINT('Ctrl Pts',(-2.00707309946949,1.,0.512953306961792));
#28079=CARTESIAN_POINT('Ctrl Pts',(-2.01187773939242,-1.,0.516902681728687));
#28080=CARTESIAN_POINT('Ctrl Pts',(-2.01187773939242,1.,0.516902681728687));
#28081=CARTESIAN_POINT('Ctrl Pts',(-2.01666477917286,-1.,0.52089359039937));
#28082=CARTESIAN_POINT('Ctrl Pts',(-2.01666477917286,1.,0.52089359039937));
#28083=CARTESIAN_POINT('Ctrl Pts',(-2.02143356304698,-1.,0.524925318333476));
#28084=CARTESIAN_POINT('Ctrl Pts',(-2.02143356304698,1.,0.524925318333476));
#28085=CARTESIAN_POINT('Ctrl Pts',(-2.0261832908329,-1.,0.528997127241914));
#28086=CARTESIAN_POINT('Ctrl Pts',(-2.0261832908329,1.,0.528997127241914));
#28087=CARTESIAN_POINT('Ctrl Pts',(-2.03091336214426,-1.,0.533108355132976));
#28088=CARTESIAN_POINT('Ctrl Pts',(-2.03091336214426,1.,0.533108355132976));
#28089=CARTESIAN_POINT('Ctrl Pts',(-2.03562362954037,-1.,0.537258489833262));
#28090=CARTESIAN_POINT('Ctrl Pts',(-2.03562362954037,1.,0.537258489833262));
#28091=CARTESIAN_POINT('Ctrl Pts',(-2.04031422690527,-1.,0.541447120615659));
#28092=CARTESIAN_POINT('Ctrl Pts',(-2.04031422690527,1.,0.541447120615659));
#28093=CARTESIAN_POINT('Ctrl Pts',(-2.04498544714588,-1.,0.54567390381743));
#28094=CARTESIAN_POINT('Ctrl Pts',(-2.04498544714588,1.,0.54567390381743));
#28095=CARTESIAN_POINT('Ctrl Pts',(-2.04963761077958,-1.,0.549938525150295));
#28096=CARTESIAN_POINT('Ctrl Pts',(-2.04963761077958,1.,0.549938525150295));
#28097=CARTESIAN_POINT('Ctrl Pts',(-2.05427091604413,-1.,0.554240657463906));
#28098=CARTESIAN_POINT('Ctrl Pts',(-2.05427091604413,1.,0.554240657463906));
#28099=CARTESIAN_POINT('Ctrl Pts',(-2.05888537756462,-1.,0.558579940185151));
#28100=CARTESIAN_POINT('Ctrl Pts',(-2.05888537756462,1.,0.558579940185151));
#28101=CARTESIAN_POINT('Ctrl Pts',(-2.06348090160589,-1.,0.562955993082261));
#28102=CARTESIAN_POINT('Ctrl Pts',(-2.06348090160589,1.,0.562955993082261));
#28103=CARTESIAN_POINT('Ctrl Pts',(-2.06805732997334,-1.,0.567368421181087));
#28104=CARTESIAN_POINT('Ctrl Pts',(-2.06805732997334,1.,0.567368421181087));
#28105=CARTESIAN_POINT('Ctrl Pts',(-2.07261449292824,-1.,0.571816823242603));
#28106=CARTESIAN_POINT('Ctrl Pts',(-2.07261449292824,1.,0.571816823242603));
#28107=CARTESIAN_POINT('Ctrl Pts',(-2.07715226767559,-1.,0.576300797416844));
#28108=CARTESIAN_POINT('Ctrl Pts',(-2.07715226767559,1.,0.576300797416844));
#28109=CARTESIAN_POINT('Ctrl Pts',(-2.08167059018418,-1.,0.580819952108063));
#28110=CARTESIAN_POINT('Ctrl Pts',(-2.08167059018418,1.,0.580819952108063));
#28111=CARTESIAN_POINT('Ctrl Pts',(-2.08616943727951,-1.,0.585373918991617));
#28112=CARTESIAN_POINT('Ctrl Pts',(-2.08616943727951,1.,0.585373918991617));
#28113=CARTESIAN_POINT('Ctrl Pts',(-2.09064881812129,-1.,0.589962365403406));
#28114=CARTESIAN_POINT('Ctrl Pts',(-2.09064881812129,1.,0.589962365403406));
#28115=CARTESIAN_POINT('Ctrl Pts',(-2.0951087622027,-1.,0.594585006052162));
#28116=CARTESIAN_POINT('Ctrl Pts',(-2.0951087622027,1.,0.594585006052162));
#28117=CARTESIAN_POINT('Ctrl Pts',(-2.0995493086477,-1.,0.599241616420533));
#28118=CARTESIAN_POINT('Ctrl Pts',(-2.0995493086477,1.,0.599241616420533));
#28119=CARTESIAN_POINT('Ctrl Pts',(-2.10397049886949,-1.,0.60393203073603));
#28120=CARTESIAN_POINT('Ctrl Pts',(-2.10397049886949,1.,0.60393203073603));
#28121=CARTESIAN_POINT('Ctrl Pts',(-2.1074919961518,-1.,0.607711315454876));
#28122=CARTESIAN_POINT('Ctrl Pts',(-2.1074919961518,1.,0.607711315454876));
#28123=CARTESIAN_POINT('Ctrl Pts',(-2.11012443807238,-1.,0.610560911689899));
#28124=CARTESIAN_POINT('Ctrl Pts',(-2.11012443807238,1.,0.610560911689899));
#28125=CARTESIAN_POINT('Ctrl Pts',(-2.11187554259986,-1.,0.6124673655618));
#28126=CARTESIAN_POINT('Ctrl Pts',(-2.11187554259986,1.,0.6124673655618));
#28127=CARTESIAN_POINT('Ctrl Pts',(-2.11275013067528,-1.,0.61342227326009));
#28128=CARTESIAN_POINT('Ctrl Pts',(-2.11275013067528,1.,0.61342227326009));
#28129=CARTESIAN_POINT('',(-1.7075470150345,1.,0.383122945602004));
#28130=CARTESIAN_POINT('Ctrl Pts',(-1.7075470150345,1.,0.383122945602004));
#28131=CARTESIAN_POINT('Ctrl Pts',(-1.71231062891958,1.,0.384119047315542));
#28132=CARTESIAN_POINT('Ctrl Pts',(-1.72162022246158,1.,0.38607079032701));
#28133=CARTESIAN_POINT('Ctrl Pts',(-1.7349317097561,1.,0.388877023509191));
#28134=CARTESIAN_POINT('Ctrl Pts',(-1.75137405313962,1.,0.392375812294307));
#28135=CARTESIAN_POINT('Ctrl Pts',(-1.7697556004756,1.,0.39634619612042));
#28136=CARTESIAN_POINT('Ctrl Pts',(-1.78598826347533,1.,0.39991940378308));
#28137=CARTESIAN_POINT('Ctrl Pts',(-1.80012077176221,1.,0.403107976170441));
#28138=CARTESIAN_POINT('Ctrl Pts',(-1.81223801813988,1.,0.405933518411838));
#28139=CARTESIAN_POINT('Ctrl Pts',(-1.8224702267854,1.,0.408428948108533));
#28140=CARTESIAN_POINT('Ctrl Pts',(-1.83100408895216,1.,0.410641256301675));
#28141=CARTESIAN_POINT('Ctrl Pts',(-1.83808953475839,1.,0.412633125322161));
#28142=CARTESIAN_POINT('Ctrl Pts',(-1.8440575707371,1.,0.41448743825434));
#28143=CARTESIAN_POINT('Ctrl Pts',(-1.84929312929882,1.,0.416300022038864));
#28144=CARTESIAN_POINT('Ctrl Pts',(-1.85417632856234,1.,0.418164129143534));
#28145=CARTESIAN_POINT('Ctrl Pts',(-1.85903281096686,1.,0.420157287975619));
#28146=CARTESIAN_POINT('Ctrl Pts',(-1.86408083334028,1.,0.422327307418275));
#28147=CARTESIAN_POINT('Ctrl Pts',(-1.86937803944323,1.,0.424678177291359));
#28148=CARTESIAN_POINT('Ctrl Pts',(-1.87486989291484,1.,0.427183828519102));
#28149=CARTESIAN_POINT('Ctrl Pts',(-1.88044229001832,1.,0.429803062482344));
#28150=CARTESIAN_POINT('Ctrl Pts',(-1.88596913666793,1.,0.432493038548748));
#28151=CARTESIAN_POINT('Ctrl Pts',(-1.89136993975504,1.,0.435225660963383));
#28152=CARTESIAN_POINT('Ctrl Pts',(-1.89663648956466,1.,0.437995003948244));
#28153=CARTESIAN_POINT('Ctrl Pts',(-1.90180124389086,1.,0.440807833704038));
#28154=CARTESIAN_POINT('Ctrl Pts',(-1.90691756144898,1.,0.44367755684915));
#28155=CARTESIAN_POINT('Ctrl Pts',(-1.9120369998112,1.,0.446617343485711));
#28156=CARTESIAN_POINT('Ctrl Pts',(-1.91718342555755,1.,0.449632260106662));
#28157=CARTESIAN_POINT('Ctrl Pts',(-1.92235380648502,1.,0.452719478359432));
#28158=CARTESIAN_POINT('Ctrl Pts',(-1.92753067150476,1.,0.455872005174371));
#28159=CARTESIAN_POINT('Ctrl Pts',(-1.93269066517934,1.,0.459081234547926));
#28160=CARTESIAN_POINT('Ctrl Pts',(-1.93781486640821,1.,0.462340031009056));
#28161=CARTESIAN_POINT('Ctrl Pts',(-1.9428979419619,1.,0.46564546202603));
#28162=CARTESIAN_POINT('Ctrl Pts',(-1.94794381136514,1.,0.468997482913135));
#28163=CARTESIAN_POINT('Ctrl Pts',(-1.95296148278133,1.,0.472397672264072));
#28164=CARTESIAN_POINT('Ctrl Pts',(-1.95796111148177,1.,0.475848034683176));
#28165=CARTESIAN_POINT('Ctrl Pts',(-1.96294933055943,1.,0.479349583074855));
#28166=CARTESIAN_POINT('Ctrl Pts',(-1.96792703422362,1.,0.48290166212069));
#28167=CARTESIAN_POINT('Ctrl Pts',(-1.97289186263272,1.,0.486502692907659));
#28168=CARTESIAN_POINT('Ctrl Pts',(-1.97783973019229,1.,0.490150627860952));
#28169=CARTESIAN_POINT('Ctrl Pts',(-1.98276658761821,1.,0.493843476541494));
#28170=CARTESIAN_POINT('Ctrl Pts',(-1.98767044752932,1.,0.497579909545574));
#28171=CARTESIAN_POINT('Ctrl Pts',(-1.99255149126155,1.,0.501359287727146));
#28172=CARTESIAN_POINT('Ctrl Pts',(-1.99741107463572,1.,0.505181361323026));
#28173=CARTESIAN_POINT('Ctrl Pts',(-2.00225107134734,1.,0.509046069886157));
#28174=CARTESIAN_POINT('Ctrl Pts',(-2.00707309946949,1.,0.512953306961792));
#28175=CARTESIAN_POINT('Ctrl Pts',(-2.01187773939242,1.,0.516902681728687));
#28176=CARTESIAN_POINT('Ctrl Pts',(-2.01666477917286,1.,0.52089359039937));
#28177=CARTESIAN_POINT('Ctrl Pts',(-2.02143356304698,1.,0.524925318333476));
#28178=CARTESIAN_POINT('Ctrl Pts',(-2.0261832908329,1.,0.528997127241914));
#28179=CARTESIAN_POINT('Ctrl Pts',(-2.03091336214426,1.,0.533108355132976));
#28180=CARTESIAN_POINT('Ctrl Pts',(-2.03562362954037,1.,0.537258489833262));
#28181=CARTESIAN_POINT('Ctrl Pts',(-2.04031422690527,1.,0.541447120615659));
#28182=CARTESIAN_POINT('Ctrl Pts',(-2.04498544714588,1.,0.54567390381743));
#28183=CARTESIAN_POINT('Ctrl Pts',(-2.04963761077958,1.,0.549938525150295));
#28184=CARTESIAN_POINT('Ctrl Pts',(-2.05427091604413,1.,0.554240657463906));
#28185=CARTESIAN_POINT('Ctrl Pts',(-2.05888537756462,1.,0.558579940185151));
#28186=CARTESIAN_POINT('Ctrl Pts',(-2.06348090160589,1.,0.562955993082261));
#28187=CARTESIAN_POINT('Ctrl Pts',(-2.06805732997334,1.,0.567368421181087));
#28188=CARTESIAN_POINT('Ctrl Pts',(-2.07261449292824,1.,0.571816823242603));
#28189=CARTESIAN_POINT('Ctrl Pts',(-2.07715226767559,1.,0.576300797416844));
#28190=CARTESIAN_POINT('Ctrl Pts',(-2.08167059018418,1.,0.580819952108063));
#28191=CARTESIAN_POINT('Ctrl Pts',(-2.08616943727951,1.,0.585373918991617));
#28192=CARTESIAN_POINT('Ctrl Pts',(-2.09064881812129,1.,0.589962365403406));
#28193=CARTESIAN_POINT('Ctrl Pts',(-2.0951087622027,1.,0.594585006052162));
#28194=CARTESIAN_POINT('Ctrl Pts',(-2.0995493086477,1.,0.599241616420533));
#28195=CARTESIAN_POINT('Ctrl Pts',(-2.10397049886949,1.,0.60393203073603));
#28196=CARTESIAN_POINT('Ctrl Pts',(-2.1074919961518,1.,0.607711315454876));
#28197=CARTESIAN_POINT('Ctrl Pts',(-2.11012443807238,1.,0.610560911689899));
#28198=CARTESIAN_POINT('Ctrl Pts',(-2.11187554259986,1.,0.6124673655618));
#28199=CARTESIAN_POINT('Ctrl Pts',(-2.11275013067528,1.,0.61342227326009));
#28200=CARTESIAN_POINT('',(-1.7075470150345,0.,0.383122945602003));
#28201=CARTESIAN_POINT('Origin',(0.,0.,0.));
#28202=CARTESIAN_POINT('',(-1.74236521665491,1.,0.163289472382896));
#28203=CARTESIAN_POINT('Origin',(0.,1.,0.));
#28204=CARTESIAN_POINT('',(-1.74236521665491,0.,0.163289472382896));
#28205=CARTESIAN_POINT('Ctrl Pts',(-2.19890268624765,-1.,0.069476445021958));
#28206=CARTESIAN_POINT('Ctrl Pts',(-2.19890268624765,1.,0.069476445021958));
#28207=CARTESIAN_POINT('Ctrl Pts',(-2.19777582085423,-1.,0.0701143536325489));
#28208=CARTESIAN_POINT('Ctrl Pts',(-2.19777582085423,1.,0.0701143536325489));
#28209=CARTESIAN_POINT('Ctrl Pts',(-2.19552129484002,-1.,0.0713863779526153));
#28210=CARTESIAN_POINT('Ctrl Pts',(-2.19552129484002,1.,0.0713863779526153));
#28211=CARTESIAN_POINT('Ctrl Pts',(-2.19213712013662,-1.,0.0732830357306724));
#28212=CARTESIAN_POINT('Ctrl Pts',(-2.19213712013662,1.,0.0732830357306724));
#28213=CARTESIAN_POINT('Ctrl Pts',(-2.1876201139953,-1.,0.0757891465836146));
#28214=CARTESIAN_POINT('Ctrl Pts',(-2.1876201139953,1.,0.0757891465836146));
#28215=CARTESIAN_POINT('Ctrl Pts',(-2.18196589448887,-1.,0.0788837727685241));
#28216=CARTESIAN_POINT('Ctrl Pts',(-2.18196589448887,1.,0.0788837727685241));
#28217=CARTESIAN_POINT('Ctrl Pts',(-2.176303712113,-1.,0.0819402680872764));
#28218=CARTESIAN_POINT('Ctrl Pts',(-2.176303712113,1.,0.0819402680872764));
#28219=CARTESIAN_POINT('Ctrl Pts',(-2.17063357870952,-1.,0.0849584620835371));
#28220=CARTESIAN_POINT('Ctrl Pts',(-2.17063357870952,1.,0.0849584620835371));
#28221=CARTESIAN_POINT('Ctrl Pts',(-2.16495552645014,-1.,0.0879381291386921));
#28222=CARTESIAN_POINT('Ctrl Pts',(-2.16495552645014,1.,0.0879381291386921));
#28223=CARTESIAN_POINT('Ctrl Pts',(-2.15926961544516,-1.,0.0908789888107264));
#28224=CARTESIAN_POINT('Ctrl Pts',(-2.15926961544516,1.,0.0908789888107264));
#28225=CARTESIAN_POINT('Ctrl Pts',(-2.1535759397817,-1.,0.0937807218867642));
#28226=CARTESIAN_POINT('Ctrl Pts',(-2.1535759397817,1.,0.0937807218867642));
#28227=CARTESIAN_POINT('Ctrl Pts',(-2.14787463531795,-1.,0.0966429852305457));
#28228=CARTESIAN_POINT('Ctrl Pts',(-2.14787463531795,1.,0.0966429852305457));
#28229=CARTESIAN_POINT('Ctrl Pts',(-2.14216588396025,-1.,0.0994654261990914));
#28230=CARTESIAN_POINT('Ctrl Pts',(-2.14216588396025,1.,0.0994654261990914));
#28231=CARTESIAN_POINT('Ctrl Pts',(-2.13644992667165,-1.,0.1022477005561));
#28232=CARTESIAN_POINT('Ctrl Pts',(-2.13644992667165,1.,0.1022477005561));
#28233=CARTESIAN_POINT('Ctrl Pts',(-2.13072704887293,-1.,0.104989479152739));
#28234=CARTESIAN_POINT('Ctrl Pts',(-2.13072704887293,1.,0.104989479152739));
#28235=CARTESIAN_POINT('Ctrl Pts',(-2.12499752307,-1.,0.10769043523109));
#28236=CARTESIAN_POINT('Ctrl Pts',(-2.12499752307,1.,0.10769043523109));
#28237=CARTESIAN_POINT('Ctrl Pts',(-2.11926155590865,-1.,0.110350236135025));
#28238=CARTESIAN_POINT('Ctrl Pts',(-2.11926155590865,1.,0.110350236135025));
#28239=CARTESIAN_POINT('Ctrl Pts',(-2.11351924490306,-1.,0.112968534419737));
#28240=CARTESIAN_POINT('Ctrl Pts',(-2.11351924490306,1.,0.112968534419737));
#28241=CARTESIAN_POINT('Ctrl Pts',(-2.10777050261309,-1.,0.115544957687926));
#28242=CARTESIAN_POINT('Ctrl Pts',(-2.10777050261309,1.,0.115544957687926));
#28243=CARTESIAN_POINT('Ctrl Pts',(-2.102015121329,-1.,0.118079107988355));
#28244=CARTESIAN_POINT('Ctrl Pts',(-2.102015121329,1.,0.118079107988355));
#28245=CARTESIAN_POINT('Ctrl Pts',(-2.0962529286773,-1.,0.120570567965122));
#28246=CARTESIAN_POINT('Ctrl Pts',(-2.0962529286773,1.,0.120570567965122));
#28247=CARTESIAN_POINT('Ctrl Pts',(-2.09048392424825,-1.,0.123018905621083));
#28248=CARTESIAN_POINT('Ctrl Pts',(-2.09048392424825,1.,0.123018905621083));
#28249=CARTESIAN_POINT('Ctrl Pts',(-2.08470840653643,-1.,0.125423679412061));
#28250=CARTESIAN_POINT('Ctrl Pts',(-2.08470840653643,1.,0.125423679412061));
#28251=CARTESIAN_POINT('Ctrl Pts',(-2.07892715110987,-1.,0.12778444527612));
#28252=CARTESIAN_POINT('Ctrl Pts',(-2.07892715110987,1.,0.12778444527612));
#28253=CARTESIAN_POINT('Ctrl Pts',(-2.07314114713063,-1.,0.130100748328403));
#28254=CARTESIAN_POINT('Ctrl Pts',(-2.07314114713063,1.,0.130100748328403));
#28255=CARTESIAN_POINT('Ctrl Pts',(-2.06735123910326,-1.,0.13237211154771));
#28256=CARTESIAN_POINT('Ctrl Pts',(-2.06735123910326,1.,0.13237211154771));
#28257=CARTESIAN_POINT('Ctrl Pts',(-2.06155781517842,-1.,0.134598026192106));
#28258=CARTESIAN_POINT('Ctrl Pts',(-2.06155781517842,1.,0.134598026192106));
#28259=CARTESIAN_POINT('Ctrl Pts',(-2.05576044414264,-1.,0.136777941218043));
#28260=CARTESIAN_POINT('Ctrl Pts',(-2.05576044414264,1.,0.136777941218043));
#28261=CARTESIAN_POINT('Ctrl Pts',(-2.04995762001328,-1.,0.138911255368966));
#28262=CARTESIAN_POINT('Ctrl Pts',(-2.04995762001328,1.,0.138911255368966));
#28263=CARTESIAN_POINT('Ctrl Pts',(-2.04414757947916,-1.,0.140997332152546));
#28264=CARTESIAN_POINT('Ctrl Pts',(-2.04414757947916,1.,0.140997332152546));
#28265=CARTESIAN_POINT('Ctrl Pts',(-2.03832911025912,-1.,0.143035515058209));
#28266=CARTESIAN_POINT('Ctrl Pts',(-2.03832911025912,1.,0.143035515058209));
#28267=CARTESIAN_POINT('Ctrl Pts',(-2.03250223739942,-1.,0.145025140186057));
#28268=CARTESIAN_POINT('Ctrl Pts',(-2.03250223739942,1.,0.145025140186057));
#28269=CARTESIAN_POINT('Ctrl Pts',(-2.02666926182017,-1.,0.146965557332583));
#28270=CARTESIAN_POINT('Ctrl Pts',(-2.02666926182017,1.,0.146965557332583));
#28271=CARTESIAN_POINT('Ctrl Pts',(-2.02083464969894,-1.,0.148856124775337));
#28272=CARTESIAN_POINT('Ctrl Pts',(-2.02083464969894,1.,0.148856124775337));
#28273=CARTESIAN_POINT('Ctrl Pts',(-2.01500291940238,-1.,0.150696157673078));
#28274=CARTESIAN_POINT('Ctrl Pts',(-2.01500291940238,1.,0.150696157673078));
#28275=CARTESIAN_POINT('Ctrl Pts',(-2.00917680318424,-1.,0.15248488362145));
#28276=CARTESIAN_POINT('Ctrl Pts',(-2.00917680318424,1.,0.15248488362145));
#28277=CARTESIAN_POINT('Ctrl Pts',(-2.00335565310543,-1.,0.154221403049722));
#28278=CARTESIAN_POINT('Ctrl Pts',(-2.00335565310543,1.,0.154221403049722));
#28279=CARTESIAN_POINT('Ctrl Pts',(-1.99753284771497,-1.,0.155904629548783));
#28280=CARTESIAN_POINT('Ctrl Pts',(-1.99753284771497,1.,0.155904629548783));
#28281=CARTESIAN_POINT('Ctrl Pts',(-1.99169810931908,-1.,0.157533331459227));
#28282=CARTESIAN_POINT('Ctrl Pts',(-1.99169810931908,1.,0.157533331459227));
#28283=CARTESIAN_POINT('Ctrl Pts',(-1.98584238283292,-1.,0.159106226437299));
#28284=CARTESIAN_POINT('Ctrl Pts',(-1.98584238283292,1.,0.159106226437299));
#28285=CARTESIAN_POINT('Ctrl Pts',(-1.97996195437559,-1.,0.160622060784611));
#28286=CARTESIAN_POINT('Ctrl Pts',(-1.97996195437559,1.,0.160622060784611));
#28287=CARTESIAN_POINT('Ctrl Pts',(-1.97406280235188,-1.,0.162079693556288));
#28288=CARTESIAN_POINT('Ctrl Pts',(-1.97406280235188,1.,0.162079693556288));
#28289=CARTESIAN_POINT('Ctrl Pts',(-1.96816512677967,-1.,0.163478185457734));
#28290=CARTESIAN_POINT('Ctrl Pts',(-1.96816512677967,1.,0.163478185457734));
#28291=CARTESIAN_POINT('Ctrl Pts',(-1.96229379940136,-1.,0.164816568920269));
#28292=CARTESIAN_POINT('Ctrl Pts',(-1.96229379940136,1.,0.164816568920269));
#28293=CARTESIAN_POINT('Ctrl Pts',(-1.9564675971873,-1.,0.166093592002812));
#28294=CARTESIAN_POINT('Ctrl Pts',(-1.9564675971873,1.,0.166093592002812));
#28295=CARTESIAN_POINT('Ctrl Pts',(-1.95069027794294,-1.,0.167307501784475));
#28296=CARTESIAN_POINT('Ctrl Pts',(-1.95069027794294,1.,0.167307501784475));
#28297=CARTESIAN_POINT('Ctrl Pts',(-1.94493757756931,-1.,0.168455741607556));
#28298=CARTESIAN_POINT('Ctrl Pts',(-1.94493757756931,1.,0.168455741607556));
#28299=CARTESIAN_POINT('Ctrl Pts',(-1.93915639211581,-1.,0.169534904817491));
#28300=CARTESIAN_POINT('Ctrl Pts',(-1.93915639211581,1.,0.169534904817491));
#28301=CARTESIAN_POINT('Ctrl Pts',(-1.93329183155539,-1.,0.170541253116201));
#28302=CARTESIAN_POINT('Ctrl Pts',(-1.93329183155539,1.,0.170541253116201));
#28303=CARTESIAN_POINT('Ctrl Pts',(-1.92731093582036,-1.,0.171471191532988));
#28304=CARTESIAN_POINT('Ctrl Pts',(-1.92731093582036,1.,0.171471191532988));
#28305=CARTESIAN_POINT('Ctrl Pts',(-1.9212233439798,-1.,0.172321621259514));
#28306=CARTESIAN_POINT('Ctrl Pts',(-1.9212233439798,1.,0.172321621259514));
#28307=CARTESIAN_POINT('Ctrl Pts',(-1.91511429159527,-1.,0.173090695383496));
#28308=CARTESIAN_POINT('Ctrl Pts',(-1.91511429159527,1.,0.173090695383496));
#28309=CARTESIAN_POINT('Ctrl Pts',(-1.90911693975267,-1.,0.173776635257817));
#28310=CARTESIAN_POINT('Ctrl Pts',(-1.90911693975267,1.,0.173776635257817));
#28311=CARTESIAN_POINT('Ctrl Pts',(-1.90335253862834,-1.,0.174375518661085));
#28312=CARTESIAN_POINT('Ctrl Pts',(-1.90335253862834,1.,0.174375518661085));
#28313=CARTESIAN_POINT('Ctrl Pts',(-1.89788101117132,-1.,0.174879405091263));
#28314=CARTESIAN_POINT('Ctrl Pts',(-1.89788101117132,1.,0.174879405091263));
#28315=CARTESIAN_POINT('Ctrl Pts',(-1.892646301985,-1.,0.175274276190844));
#28316=CARTESIAN_POINT('Ctrl Pts',(-1.892646301985,1.,0.175274276190844));
#28317=CARTESIAN_POINT('Ctrl Pts',(-1.88742606273259,-1.,0.175538155840648));
#28318=CARTESIAN_POINT('Ctrl Pts',(-1.88742606273259,1.,0.175538155840648));
#28319=CARTESIAN_POINT('Ctrl Pts',(-1.88188663145367,-1.,0.175644148889698));
#28320=CARTESIAN_POINT('Ctrl Pts',(-1.88188663145367,1.,0.175644148889698));
#28321=CARTESIAN_POINT('Ctrl Pts',(-1.87563767773588,-1.,0.175563480746485));
#28322=CARTESIAN_POINT('Ctrl Pts',(-1.87563767773588,1.,0.175563480746485));
#28323=CARTESIAN_POINT('Ctrl Pts',(-1.86828349694799,-1.,0.175268337590758));
#28324=CARTESIAN_POINT('Ctrl Pts',(-1.86828349694799,1.,0.175268337590758));
#28325=CARTESIAN_POINT('Ctrl Pts',(-1.85948367088837,-1.,0.17473525927603));
#28326=CARTESIAN_POINT('Ctrl Pts',(-1.85948367088837,1.,0.17473525927603));
#28327=CARTESIAN_POINT('Ctrl Pts',(-1.8489811319852,-1.,0.173946627587731));
#28328=CARTESIAN_POINT('Ctrl Pts',(-1.8489811319852,1.,0.173946627587731));
#28329=CARTESIAN_POINT('Ctrl Pts',(-1.83658380527692,-1.,0.1728894428919));
#28330=CARTESIAN_POINT('Ctrl Pts',(-1.83658380527692,1.,0.1728894428919));
#28331=CARTESIAN_POINT('Ctrl Pts',(-1.82215766811545,-1.,0.171554770204119));
#28332=CARTESIAN_POINT('Ctrl Pts',(-1.82215766811545,1.,0.171554770204119));
#28333=CARTESIAN_POINT('Ctrl Pts',(-1.80561530629706,-1.,0.169936923904608));
#28334=CARTESIAN_POINT('Ctrl Pts',(-1.80561530629706,1.,0.169936923904608));
#28335=CARTESIAN_POINT('Ctrl Pts',(-1.7869064998507,-1.,0.168032772805197));
#28336=CARTESIAN_POINT('Ctrl Pts',(-1.7869064998507,1.,0.168032772805197));
#28337=CARTESIAN_POINT('Ctrl Pts',(-1.77018771684844,-1.,0.1662793551464));
#28338=CARTESIAN_POINT('Ctrl Pts',(-1.77018771684844,1.,0.1662793551464));
#28339=CARTESIAN_POINT('Ctrl Pts',(-1.75666056638427,-1.,0.164834765707158));
#28340=CARTESIAN_POINT('Ctrl Pts',(-1.75666056638427,1.,0.164834765707158));
#28341=CARTESIAN_POINT('Ctrl Pts',(-1.7472034950333,-1.,0.163814161002002));
#28342=CARTESIAN_POINT('Ctrl Pts',(-1.7472034950333,1.,0.163814161002002));
#28343=CARTESIAN_POINT('Ctrl Pts',(-1.74236521665491,-1.,0.163289472382896));
#28344=CARTESIAN_POINT('Ctrl Pts',(-1.74236521665491,1.,0.163289472382896));
#28345=CARTESIAN_POINT('',(-2.19890268624765,1.,0.069476445021958));
#28346=CARTESIAN_POINT('Ctrl Pts',(-2.19890268624765,1.,0.069476445021958));
#28347=CARTESIAN_POINT('Ctrl Pts',(-2.19777582085423,1.,0.0701143536325489));
#28348=CARTESIAN_POINT('Ctrl Pts',(-2.19552129484002,1.,0.0713863779526153));
#28349=CARTESIAN_POINT('Ctrl Pts',(-2.19213712013662,1.,0.0732830357306724));
#28350=CARTESIAN_POINT('Ctrl Pts',(-2.1876201139953,1.,0.0757891465836146));
#28351=CARTESIAN_POINT('Ctrl Pts',(-2.18196589448887,1.,0.0788837727685241));
#28352=CARTESIAN_POINT('Ctrl Pts',(-2.176303712113,1.,0.0819402680872764));
#28353=CARTESIAN_POINT('Ctrl Pts',(-2.17063357870952,1.,0.0849584620835371));
#28354=CARTESIAN_POINT('Ctrl Pts',(-2.16495552645014,1.,0.0879381291386921));
#28355=CARTESIAN_POINT('Ctrl Pts',(-2.15926961544516,1.,0.0908789888107264));
#28356=CARTESIAN_POINT('Ctrl Pts',(-2.1535759397817,1.,0.0937807218867642));
#28357=CARTESIAN_POINT('Ctrl Pts',(-2.14787463531795,1.,0.0966429852305457));
#28358=CARTESIAN_POINT('Ctrl Pts',(-2.14216588396025,1.,0.0994654261990914));
#28359=CARTESIAN_POINT('Ctrl Pts',(-2.13644992667165,1.,0.1022477005561));
#28360=CARTESIAN_POINT('Ctrl Pts',(-2.13072704887293,1.,0.104989479152739));
#28361=CARTESIAN_POINT('Ctrl Pts',(-2.12499752307,1.,0.10769043523109));
#28362=CARTESIAN_POINT('Ctrl Pts',(-2.11926155590865,1.,0.110350236135025));
#28363=CARTESIAN_POINT('Ctrl Pts',(-2.11351924490306,1.,0.112968534419737));
#28364=CARTESIAN_POINT('Ctrl Pts',(-2.10777050261309,1.,0.115544957687926));
#28365=CARTESIAN_POINT('Ctrl Pts',(-2.102015121329,1.,0.118079107988355));
#28366=CARTESIAN_POINT('Ctrl Pts',(-2.0962529286773,1.,0.120570567965122));
#28367=CARTESIAN_POINT('Ctrl Pts',(-2.09048392424825,1.,0.123018905621083));
#28368=CARTESIAN_POINT('Ctrl Pts',(-2.08470840653643,1.,0.125423679412061));
#28369=CARTESIAN_POINT('Ctrl Pts',(-2.07892715110987,1.,0.12778444527612));
#28370=CARTESIAN_POINT('Ctrl Pts',(-2.07314114713063,1.,0.130100748328403));
#28371=CARTESIAN_POINT('Ctrl Pts',(-2.06735123910326,1.,0.13237211154771));
#28372=CARTESIAN_POINT('Ctrl Pts',(-2.06155781517842,1.,0.134598026192106));
#28373=CARTESIAN_POINT('Ctrl Pts',(-2.05576044414264,1.,0.136777941218043));
#28374=CARTESIAN_POINT('Ctrl Pts',(-2.04995762001328,1.,0.138911255368966));
#28375=CARTESIAN_POINT('Ctrl Pts',(-2.04414757947916,1.,0.140997332152546));
#28376=CARTESIAN_POINT('Ctrl Pts',(-2.03832911025912,1.,0.143035515058209));
#28377=CARTESIAN_POINT('Ctrl Pts',(-2.03250223739942,1.,0.145025140186057));
#28378=CARTESIAN_POINT('Ctrl Pts',(-2.02666926182017,1.,0.146965557332583));
#28379=CARTESIAN_POINT('Ctrl Pts',(-2.02083464969894,1.,0.148856124775337));
#28380=CARTESIAN_POINT('Ctrl Pts',(-2.01500291940238,1.,0.150696157673078));
#28381=CARTESIAN_POINT('Ctrl Pts',(-2.00917680318424,1.,0.15248488362145));
#28382=CARTESIAN_POINT('Ctrl Pts',(-2.00335565310543,1.,0.154221403049722));
#28383=CARTESIAN_POINT('Ctrl Pts',(-1.99753284771497,1.,0.155904629548783));
#28384=CARTESIAN_POINT('Ctrl Pts',(-1.99169810931908,1.,0.157533331459227));
#28385=CARTESIAN_POINT('Ctrl Pts',(-1.98584238283292,1.,0.159106226437299));
#28386=CARTESIAN_POINT('Ctrl Pts',(-1.97996195437559,1.,0.160622060784611));
#28387=CARTESIAN_POINT('Ctrl Pts',(-1.97406280235188,1.,0.162079693556288));
#28388=CARTESIAN_POINT('Ctrl Pts',(-1.96816512677967,1.,0.163478185457734));
#28389=CARTESIAN_POINT('Ctrl Pts',(-1.96229379940136,1.,0.164816568920269));
#28390=CARTESIAN_POINT('Ctrl Pts',(-1.9564675971873,1.,0.166093592002812));
#28391=CARTESIAN_POINT('Ctrl Pts',(-1.95069027794294,1.,0.167307501784475));
#28392=CARTESIAN_POINT('Ctrl Pts',(-1.94493757756931,1.,0.168455741607556));
#28393=CARTESIAN_POINT('Ctrl Pts',(-1.93915639211581,1.,0.169534904817491));
#28394=CARTESIAN_POINT('Ctrl Pts',(-1.93329183155539,1.,0.170541253116201));
#28395=CARTESIAN_POINT('Ctrl Pts',(-1.92731093582036,1.,0.171471191532988));
#28396=CARTESIAN_POINT('Ctrl Pts',(-1.9212233439798,1.,0.172321621259514));
#28397=CARTESIAN_POINT('Ctrl Pts',(-1.91511429159527,1.,0.173090695383496));
#28398=CARTESIAN_POINT('Ctrl Pts',(-1.90911693975267,1.,0.173776635257817));
#28399=CARTESIAN_POINT('Ctrl Pts',(-1.90335253862834,1.,0.174375518661085));
#28400=CARTESIAN_POINT('Ctrl Pts',(-1.89788101117132,1.,0.174879405091263));
#28401=CARTESIAN_POINT('Ctrl Pts',(-1.892646301985,1.,0.175274276190844));
#28402=CARTESIAN_POINT('Ctrl Pts',(-1.88742606273259,1.,0.175538155840648));
#28403=CARTESIAN_POINT('Ctrl Pts',(-1.88188663145367,1.,0.175644148889698));
#28404=CARTESIAN_POINT('Ctrl Pts',(-1.87563767773588,1.,0.175563480746485));
#28405=CARTESIAN_POINT('Ctrl Pts',(-1.86828349694799,1.,0.175268337590758));
#28406=CARTESIAN_POINT('Ctrl Pts',(-1.85948367088837,1.,0.17473525927603));
#28407=CARTESIAN_POINT('Ctrl Pts',(-1.8489811319852,1.,0.173946627587731));
#28408=CARTESIAN_POINT('Ctrl Pts',(-1.83658380527692,1.,0.1728894428919));
#28409=CARTESIAN_POINT('Ctrl Pts',(-1.82215766811545,1.,0.171554770204119));
#28410=CARTESIAN_POINT('Ctrl Pts',(-1.80561530629706,1.,0.169936923904608));
#28411=CARTESIAN_POINT('Ctrl Pts',(-1.7869064998507,1.,0.168032772805197));
#28412=CARTESIAN_POINT('Ctrl Pts',(-1.77018771684844,1.,0.1662793551464));
#28413=CARTESIAN_POINT('Ctrl Pts',(-1.75666056638427,1.,0.164834765707158));
#28414=CARTESIAN_POINT('Ctrl Pts',(-1.7472034950333,1.,0.163814161002002));
#28415=CARTESIAN_POINT('Ctrl Pts',(-1.74236521665491,1.,0.163289472382896));
#28416=CARTESIAN_POINT('',(-2.19890268624765,0.,0.069476445021958));
#28417=CARTESIAN_POINT('Origin',(-2.19890268624765,0.,-0.0694764450219585));
#28418=CARTESIAN_POINT('',(-2.19890268624765,1.,-0.0694764450219585));
#28419=CARTESIAN_POINT('',(-2.19890268624765,1.,0.069476445021958));
#28420=CARTESIAN_POINT('',(-2.19890268624765,0.,-0.0694764450219585));
#28421=CARTESIAN_POINT('Ctrl Pts',(-1.74236521665491,-1.,-0.163289472382896));
#28422=CARTESIAN_POINT('Ctrl Pts',(-1.74236521665491,1.,-0.163289472382896));
#28423=CARTESIAN_POINT('Ctrl Pts',(-1.74720349503904,-1.,-0.163814161002474));
#28424=CARTESIAN_POINT('Ctrl Pts',(-1.74720349503904,1.,-0.163814161002474));
#28425=CARTESIAN_POINT('Ctrl Pts',(-1.75666056640041,-1.,-0.164834765708484));
#28426=CARTESIAN_POINT('Ctrl Pts',(-1.75666056640041,1.,-0.164834765708484));
#28427=CARTESIAN_POINT('Ctrl Pts',(-1.77018771687692,-1.,-0.166279355148738));
#28428=CARTESIAN_POINT('Ctrl Pts',(-1.77018771687692,1.,-0.166279355148738));
#28429=CARTESIAN_POINT('Ctrl Pts',(-1.78690649988931,-1.,-0.16803277280837));
#28430=CARTESIAN_POINT('Ctrl Pts',(-1.78690649988931,1.,-0.16803277280837));
#28431=CARTESIAN_POINT('Ctrl Pts',(-1.80561530633924,-1.,-0.169936923908078));
#28432=CARTESIAN_POINT('Ctrl Pts',(-1.80561530633924,1.,-0.169936923908078));
#28433=CARTESIAN_POINT('Ctrl Pts',(-1.82215766815414,-1.,-0.171554770207306));
#28434=CARTESIAN_POINT('Ctrl Pts',(-1.82215766815414,1.,-0.171554770207306));
#28435=CARTESIAN_POINT('Ctrl Pts',(-1.83658380530747,-1.,-0.17288944289442));
#28436=CARTESIAN_POINT('Ctrl Pts',(-1.83658380530747,1.,-0.17288944289442));
#28437=CARTESIAN_POINT('Ctrl Pts',(-1.84898113200543,-1.,-0.173946627589401));
#28438=CARTESIAN_POINT('Ctrl Pts',(-1.84898113200543,1.,-0.173946627589401));
#28439=CARTESIAN_POINT('Ctrl Pts',(-1.85948367089838,-1.,-0.174735259276856));
#28440=CARTESIAN_POINT('Ctrl Pts',(-1.85948367089838,1.,-0.174735259276856));
#28441=CARTESIAN_POINT('Ctrl Pts',(-1.86828349694972,-1.,-0.175268337590901));
#28442=CARTESIAN_POINT('Ctrl Pts',(-1.86828349694972,1.,-0.175268337590901));
#28443=CARTESIAN_POINT('Ctrl Pts',(-1.87563767773249,-1.,-0.175563480746205));
#28444=CARTESIAN_POINT('Ctrl Pts',(-1.87563767773249,1.,-0.175563480746205));
#28445=CARTESIAN_POINT('Ctrl Pts',(-1.88188663144846,-1.,-0.175644148889271));
#28446=CARTESIAN_POINT('Ctrl Pts',(-1.88188663144846,1.,-0.175644148889271));
#28447=CARTESIAN_POINT('Ctrl Pts',(-1.88742606272818,-1.,-0.175538155840286));
#28448=CARTESIAN_POINT('Ctrl Pts',(-1.88742606272818,1.,-0.175538155840286));
#28449=CARTESIAN_POINT('Ctrl Pts',(-1.89264630198279,-1.,-0.175274276190664));
#28450=CARTESIAN_POINT('Ctrl Pts',(-1.89264630198279,1.,-0.175274276190664));
#28451=CARTESIAN_POINT('Ctrl Pts',(-1.89788101117148,-1.,-0.174879405091277));
#28452=CARTESIAN_POINT('Ctrl Pts',(-1.89788101117148,1.,-0.174879405091277));
#28453=CARTESIAN_POINT('Ctrl Pts',(-1.90335253863003,-1.,-0.174375518661222));
#28454=CARTESIAN_POINT('Ctrl Pts',(-1.90335253863003,1.,-0.174375518661222));
#28455=CARTESIAN_POINT('Ctrl Pts',(-1.90911693975475,-1.,-0.173776635257984));
#28456=CARTESIAN_POINT('Ctrl Pts',(-1.90911693975475,1.,-0.173776635257984));
#28457=CARTESIAN_POINT('Ctrl Pts',(-1.91511429159681,-1.,-0.173090695383619));
#28458=CARTESIAN_POINT('Ctrl Pts',(-1.91511429159681,1.,-0.173090695383619));
#28459=CARTESIAN_POINT('Ctrl Pts',(-1.92122334398034,-1.,-0.172321621259557));
#28460=CARTESIAN_POINT('Ctrl Pts',(-1.92122334398034,1.,-0.172321621259557));
#28461=CARTESIAN_POINT('Ctrl Pts',(-1.92731093582,-1.,-0.17147119153296));
#28462=CARTESIAN_POINT('Ctrl Pts',(-1.92731093582,1.,-0.17147119153296));
#28463=CARTESIAN_POINT('Ctrl Pts',(-1.93329183155455,-1.,-0.170541253116136));
#28464=CARTESIAN_POINT('Ctrl Pts',(-1.93329183155455,1.,-0.170541253116136));
#28465=CARTESIAN_POINT('Ctrl Pts',(-1.93915639211497,-1.,-0.169534904817425));
#28466=CARTESIAN_POINT('Ctrl Pts',(-1.93915639211497,1.,-0.169534904817425));
#28467=CARTESIAN_POINT('Ctrl Pts',(-1.94493757756879,-1.,-0.168455741607516));
#28468=CARTESIAN_POINT('Ctrl Pts',(-1.94493757756879,1.,-0.168455741607516));
#28469=CARTESIAN_POINT('Ctrl Pts',(-1.95069027794286,-1.,-0.167307501784469));
#28470=CARTESIAN_POINT('Ctrl Pts',(-1.95069027794286,1.,-0.167307501784469));
#28471=CARTESIAN_POINT('Ctrl Pts',(-1.95646759718755,-1.,-0.166093592002833));
#28472=CARTESIAN_POINT('Ctrl Pts',(-1.95646759718755,1.,-0.166093592002833));
#28473=CARTESIAN_POINT('Ctrl Pts',(-1.96229379940174,-1.,-0.1648165689203));
#28474=CARTESIAN_POINT('Ctrl Pts',(-1.96229379940174,1.,-0.1648165689203));
#28475=CARTESIAN_POINT('Ctrl Pts',(-1.96816512678,-1.,-0.16347818545776));
#28476=CARTESIAN_POINT('Ctrl Pts',(-1.96816512678,1.,-0.16347818545776));
#28477=CARTESIAN_POINT('Ctrl Pts',(-1.97406280235204,-1.,-0.162079693556302));
#28478=CARTESIAN_POINT('Ctrl Pts',(-1.97406280235204,1.,-0.162079693556302));
#28479=CARTESIAN_POINT('Ctrl Pts',(-1.97996195437557,-1.,-0.16062206078461));
#28480=CARTESIAN_POINT('Ctrl Pts',(-1.97996195437557,1.,-0.16062206078461));
#28481=CARTESIAN_POINT('Ctrl Pts',(-1.98584238283279,-1.,-0.159106226437289));
#28482=CARTESIAN_POINT('Ctrl Pts',(-1.98584238283279,1.,-0.159106226437289));
#28483=CARTESIAN_POINT('Ctrl Pts',(-1.99169810931893,-1.,-0.157533331459215));
#28484=CARTESIAN_POINT('Ctrl Pts',(-1.99169810931893,1.,-0.157533331459215));
#28485=CARTESIAN_POINT('Ctrl Pts',(-1.99753284771487,-1.,-0.155904629548775));
#28486=CARTESIAN_POINT('Ctrl Pts',(-1.99753284771487,1.,-0.155904629548775));
#28487=CARTESIAN_POINT('Ctrl Pts',(-2.00335565310539,-1.,-0.154221403049719));
#28488=CARTESIAN_POINT('Ctrl Pts',(-2.00335565310539,1.,-0.154221403049719));
#28489=CARTESIAN_POINT('Ctrl Pts',(-2.00917680318426,-1.,-0.152484883621452));
#28490=CARTESIAN_POINT('Ctrl Pts',(-2.00917680318426,1.,-0.152484883621452));
#28491=CARTESIAN_POINT('Ctrl Pts',(-2.01500291940243,-1.,-0.150696157673084));
#28492=CARTESIAN_POINT('Ctrl Pts',(-2.01500291940243,1.,-0.150696157673084));
#28493=CARTESIAN_POINT('Ctrl Pts',(-2.02083464969897,-1.,-0.148856124775343));
#28494=CARTESIAN_POINT('Ctrl Pts',(-2.02083464969897,1.,-0.148856124775343));
#28495=CARTESIAN_POINT('Ctrl Pts',(-2.02666926182017,-1.,-0.146965557332586));
#28496=CARTESIAN_POINT('Ctrl Pts',(-2.02666926182017,1.,-0.146965557332586));
#28497=CARTESIAN_POINT('Ctrl Pts',(-2.03250223739941,-1.,-0.145025140186058));
#28498=CARTESIAN_POINT('Ctrl Pts',(-2.03250223739941,1.,-0.145025140186058));
#28499=CARTESIAN_POINT('Ctrl Pts',(-2.03832911025913,-1.,-0.143035515058208));
#28500=CARTESIAN_POINT('Ctrl Pts',(-2.03832911025913,1.,-0.143035515058208));
#28501=CARTESIAN_POINT('Ctrl Pts',(-2.04414757947919,-1.,-0.140997332152545));
#28502=CARTESIAN_POINT('Ctrl Pts',(-2.04414757947919,1.,-0.140997332152545));
#28503=CARTESIAN_POINT('Ctrl Pts',(-2.04995762001333,-1.,-0.138911255368966));
#28504=CARTESIAN_POINT('Ctrl Pts',(-2.04995762001333,1.,-0.138911255368966));
#28505=CARTESIAN_POINT('Ctrl Pts',(-2.0557604441427,-1.,-0.136777941218044));
#28506=CARTESIAN_POINT('Ctrl Pts',(-2.0557604441427,1.,-0.136777941218044));
#28507=CARTESIAN_POINT('Ctrl Pts',(-2.06155781517844,-1.,-0.134598026192107));
#28508=CARTESIAN_POINT('Ctrl Pts',(-2.06155781517844,1.,-0.134598026192107));
#28509=CARTESIAN_POINT('Ctrl Pts',(-2.06735123910319,-1.,-0.13237211154771));
#28510=CARTESIAN_POINT('Ctrl Pts',(-2.06735123910319,1.,-0.13237211154771));
#28511=CARTESIAN_POINT('Ctrl Pts',(-2.07314114713047,-1.,-0.130100748328401));
#28512=CARTESIAN_POINT('Ctrl Pts',(-2.07314114713047,1.,-0.130100748328401));
#28513=CARTESIAN_POINT('Ctrl Pts',(-2.07892715110967,-1.,-0.127784445276116));
#28514=CARTESIAN_POINT('Ctrl Pts',(-2.07892715110967,1.,-0.127784445276116));
#28515=CARTESIAN_POINT('Ctrl Pts',(-2.08470840653628,-1.,-0.125423679412058));
#28516=CARTESIAN_POINT('Ctrl Pts',(-2.08470840653628,1.,-0.125423679412058));
#28517=CARTESIAN_POINT('Ctrl Pts',(-2.09048392424826,-1.,-0.123018905621083));
#28518=CARTESIAN_POINT('Ctrl Pts',(-2.09048392424826,1.,-0.123018905621083));
#28519=CARTESIAN_POINT('Ctrl Pts',(-2.09625292867756,-1.,-0.120570567965129));
#28520=CARTESIAN_POINT('Ctrl Pts',(-2.09625292867756,1.,-0.120570567965129));
#28521=CARTESIAN_POINT('Ctrl Pts',(-2.10201512132945,-1.,-0.118079107988368));
#28522=CARTESIAN_POINT('Ctrl Pts',(-2.10201512132945,1.,-0.118079107988368));
#28523=CARTESIAN_POINT('Ctrl Pts',(-2.10777050261359,-1.,-0.11554495768794));
#28524=CARTESIAN_POINT('Ctrl Pts',(-2.10777050261359,1.,-0.11554495768794));
#28525=CARTESIAN_POINT('Ctrl Pts',(-2.11351924490335,-1.,-0.112968534419746));
#28526=CARTESIAN_POINT('Ctrl Pts',(-2.11351924490335,1.,-0.112968534419746));
#28527=CARTESIAN_POINT('Ctrl Pts',(-2.11926155590849,-1.,-0.11035023613502));
#28528=CARTESIAN_POINT('Ctrl Pts',(-2.11926155590849,1.,-0.11035023613502));
#28529=CARTESIAN_POINT('Ctrl Pts',(-2.12499752306927,-1.,-0.107690435231068));
#28530=CARTESIAN_POINT('Ctrl Pts',(-2.12499752306927,1.,-0.107690435231068));
#28531=CARTESIAN_POINT('Ctrl Pts',(-2.1307270488718,-1.,-0.104989479152703));
#28532=CARTESIAN_POINT('Ctrl Pts',(-2.1307270488718,1.,-0.104989479152703));
#28533=CARTESIAN_POINT('Ctrl Pts',(-2.13644992667052,-1.,-0.102247700556064));
#28534=CARTESIAN_POINT('Ctrl Pts',(-2.13644992667052,1.,-0.102247700556064));
#28535=CARTESIAN_POINT('Ctrl Pts',(-2.14216588395974,-1.,-0.0994654261990744));
#28536=CARTESIAN_POINT('Ctrl Pts',(-2.14216588395974,1.,-0.0994654261990744));
#28537=CARTESIAN_POINT('Ctrl Pts',(-2.14787463531864,-1.,-0.096642985230569));
#28538=CARTESIAN_POINT('Ctrl Pts',(-2.14787463531864,1.,-0.096642985230569));
#28539=CARTESIAN_POINT('Ctrl Pts',(-2.15357593978377,-1.,-0.0937807218868346));
#28540=CARTESIAN_POINT('Ctrl Pts',(-2.15357593978377,1.,-0.0937807218868346));
#28541=CARTESIAN_POINT('Ctrl Pts',(-2.15926961544808,-1.,-0.0908789888108267));
#28542=CARTESIAN_POINT('Ctrl Pts',(-2.15926961544808,1.,-0.0908789888108267));
#28543=CARTESIAN_POINT('Ctrl Pts',(-2.16495552645275,-1.,-0.0879381291387824));
#28544=CARTESIAN_POINT('Ctrl Pts',(-2.16495552645275,1.,-0.0879381291387824));
#28545=CARTESIAN_POINT('Ctrl Pts',(-2.17063357871031,-1.,-0.0849584620835644));
#28546=CARTESIAN_POINT('Ctrl Pts',(-2.17063357871031,1.,-0.0849584620835644));
#28547=CARTESIAN_POINT('Ctrl Pts',(-2.1763037121106,-1.,-0.0819402680871941));
#28548=CARTESIAN_POINT('Ctrl Pts',(-2.1763037121106,1.,-0.0819402680871941));
#28549=CARTESIAN_POINT('Ctrl Pts',(-2.18196589448304,-1.,-0.0788837727683229));
#28550=CARTESIAN_POINT('Ctrl Pts',(-2.18196589448304,1.,-0.0788837727683229));
#28551=CARTESIAN_POINT('Ctrl Pts',(-2.1876201139874,-1.,-0.0757891465833413));
#28552=CARTESIAN_POINT('Ctrl Pts',(-2.1876201139874,1.,-0.0757891465833413));
#28553=CARTESIAN_POINT('Ctrl Pts',(-2.19213712012956,-1.,-0.0732830357304277));
#28554=CARTESIAN_POINT('Ctrl Pts',(-2.19213712012956,1.,-0.0732830357304277));
#28555=CARTESIAN_POINT('Ctrl Pts',(-2.19552129483562,-1.,-0.0713863779524629));
#28556=CARTESIAN_POINT('Ctrl Pts',(-2.19552129483562,1.,-0.0713863779524629));
#28557=CARTESIAN_POINT('Ctrl Pts',(-2.19777582085261,-1.,-0.0701143536324927));
#28558=CARTESIAN_POINT('Ctrl Pts',(-2.19777582085261,1.,-0.0701143536324927));
#28559=CARTESIAN_POINT('Ctrl Pts',(-2.19890268624765,-1.,-0.0694764450219585));
#28560=CARTESIAN_POINT('Ctrl Pts',(-2.19890268624765,1.,-0.0694764450219585));
#28561=CARTESIAN_POINT('',(-1.74236521665491,1.,-0.163289472382896));
#28562=CARTESIAN_POINT('Ctrl Pts',(-1.74236521665491,1.,-0.163289472382896));
#28563=CARTESIAN_POINT('Ctrl Pts',(-1.74720349503904,1.,-0.163814161002474));
#28564=CARTESIAN_POINT('Ctrl Pts',(-1.75666056640041,1.,-0.164834765708484));
#28565=CARTESIAN_POINT('Ctrl Pts',(-1.77018771687692,1.,-0.166279355148738));
#28566=CARTESIAN_POINT('Ctrl Pts',(-1.78690649988931,1.,-0.16803277280837));
#28567=CARTESIAN_POINT('Ctrl Pts',(-1.80561530633924,1.,-0.169936923908078));
#28568=CARTESIAN_POINT('Ctrl Pts',(-1.82215766815414,1.,-0.171554770207306));
#28569=CARTESIAN_POINT('Ctrl Pts',(-1.83658380530747,1.,-0.17288944289442));
#28570=CARTESIAN_POINT('Ctrl Pts',(-1.84898113200543,1.,-0.173946627589401));
#28571=CARTESIAN_POINT('Ctrl Pts',(-1.85948367089838,1.,-0.174735259276856));
#28572=CARTESIAN_POINT('Ctrl Pts',(-1.86828349694972,1.,-0.175268337590901));
#28573=CARTESIAN_POINT('Ctrl Pts',(-1.87563767773249,1.,-0.175563480746205));
#28574=CARTESIAN_POINT('Ctrl Pts',(-1.88188663144846,1.,-0.175644148889271));
#28575=CARTESIAN_POINT('Ctrl Pts',(-1.88742606272818,1.,-0.175538155840286));
#28576=CARTESIAN_POINT('Ctrl Pts',(-1.89264630198279,1.,-0.175274276190664));
#28577=CARTESIAN_POINT('Ctrl Pts',(-1.89788101117148,1.,-0.174879405091277));
#28578=CARTESIAN_POINT('Ctrl Pts',(-1.90335253863003,1.,-0.174375518661222));
#28579=CARTESIAN_POINT('Ctrl Pts',(-1.90911693975475,1.,-0.173776635257984));
#28580=CARTESIAN_POINT('Ctrl Pts',(-1.91511429159681,1.,-0.173090695383619));
#28581=CARTESIAN_POINT('Ctrl Pts',(-1.92122334398034,1.,-0.172321621259557));
#28582=CARTESIAN_POINT('Ctrl Pts',(-1.92731093582,1.,-0.17147119153296));
#28583=CARTESIAN_POINT('Ctrl Pts',(-1.93329183155455,1.,-0.170541253116136));
#28584=CARTESIAN_POINT('Ctrl Pts',(-1.93915639211497,1.,-0.169534904817425));
#28585=CARTESIAN_POINT('Ctrl Pts',(-1.94493757756879,1.,-0.168455741607516));
#28586=CARTESIAN_POINT('Ctrl Pts',(-1.95069027794286,1.,-0.167307501784469));
#28587=CARTESIAN_POINT('Ctrl Pts',(-1.95646759718755,1.,-0.166093592002833));
#28588=CARTESIAN_POINT('Ctrl Pts',(-1.96229379940174,1.,-0.1648165689203));
#28589=CARTESIAN_POINT('Ctrl Pts',(-1.96816512678,1.,-0.16347818545776));
#28590=CARTESIAN_POINT('Ctrl Pts',(-1.97406280235204,1.,-0.162079693556302));
#28591=CARTESIAN_POINT('Ctrl Pts',(-1.97996195437557,1.,-0.16062206078461));
#28592=CARTESIAN_POINT('Ctrl Pts',(-1.98584238283279,1.,-0.159106226437289));
#28593=CARTESIAN_POINT('Ctrl Pts',(-1.99169810931893,1.,-0.157533331459215));
#28594=CARTESIAN_POINT('Ctrl Pts',(-1.99753284771487,1.,-0.155904629548775));
#28595=CARTESIAN_POINT('Ctrl Pts',(-2.00335565310539,1.,-0.154221403049719));
#28596=CARTESIAN_POINT('Ctrl Pts',(-2.00917680318426,1.,-0.152484883621452));
#28597=CARTESIAN_POINT('Ctrl Pts',(-2.01500291940243,1.,-0.150696157673084));
#28598=CARTESIAN_POINT('Ctrl Pts',(-2.02083464969897,1.,-0.148856124775343));
#28599=CARTESIAN_POINT('Ctrl Pts',(-2.02666926182017,1.,-0.146965557332586));
#28600=CARTESIAN_POINT('Ctrl Pts',(-2.03250223739941,1.,-0.145025140186058));
#28601=CARTESIAN_POINT('Ctrl Pts',(-2.03832911025913,1.,-0.143035515058208));
#28602=CARTESIAN_POINT('Ctrl Pts',(-2.04414757947919,1.,-0.140997332152545));
#28603=CARTESIAN_POINT('Ctrl Pts',(-2.04995762001333,1.,-0.138911255368966));
#28604=CARTESIAN_POINT('Ctrl Pts',(-2.0557604441427,1.,-0.136777941218044));
#28605=CARTESIAN_POINT('Ctrl Pts',(-2.06155781517844,1.,-0.134598026192107));
#28606=CARTESIAN_POINT('Ctrl Pts',(-2.06735123910319,1.,-0.13237211154771));
#28607=CARTESIAN_POINT('Ctrl Pts',(-2.07314114713047,1.,-0.130100748328401));
#28608=CARTESIAN_POINT('Ctrl Pts',(-2.07892715110967,1.,-0.127784445276116));
#28609=CARTESIAN_POINT('Ctrl Pts',(-2.08470840653628,1.,-0.125423679412058));
#28610=CARTESIAN_POINT('Ctrl Pts',(-2.09048392424826,1.,-0.123018905621083));
#28611=CARTESIAN_POINT('Ctrl Pts',(-2.09625292867756,1.,-0.120570567965129));
#28612=CARTESIAN_POINT('Ctrl Pts',(-2.10201512132945,1.,-0.118079107988368));
#28613=CARTESIAN_POINT('Ctrl Pts',(-2.10777050261359,1.,-0.11554495768794));
#28614=CARTESIAN_POINT('Ctrl Pts',(-2.11351924490335,1.,-0.112968534419746));
#28615=CARTESIAN_POINT('Ctrl Pts',(-2.11926155590849,1.,-0.11035023613502));
#28616=CARTESIAN_POINT('Ctrl Pts',(-2.12499752306927,1.,-0.107690435231068));
#28617=CARTESIAN_POINT('Ctrl Pts',(-2.1307270488718,1.,-0.104989479152703));
#28618=CARTESIAN_POINT('Ctrl Pts',(-2.13644992667052,1.,-0.102247700556064));
#28619=CARTESIAN_POINT('Ctrl Pts',(-2.14216588395974,1.,-0.0994654261990744));
#28620=CARTESIAN_POINT('Ctrl Pts',(-2.14787463531864,1.,-0.096642985230569));
#28621=CARTESIAN_POINT('Ctrl Pts',(-2.15357593978377,1.,-0.0937807218868346));
#28622=CARTESIAN_POINT('Ctrl Pts',(-2.15926961544808,1.,-0.0908789888108267));
#28623=CARTESIAN_POINT('Ctrl Pts',(-2.16495552645275,1.,-0.0879381291387824));
#28624=CARTESIAN_POINT('Ctrl Pts',(-2.17063357871031,1.,-0.0849584620835644));
#28625=CARTESIAN_POINT('Ctrl Pts',(-2.1763037121106,1.,-0.0819402680871941));
#28626=CARTESIAN_POINT('Ctrl Pts',(-2.18196589448304,1.,-0.0788837727683229));
#28627=CARTESIAN_POINT('Ctrl Pts',(-2.1876201139874,1.,-0.0757891465833413));
#28628=CARTESIAN_POINT('Ctrl Pts',(-2.19213712012956,1.,-0.0732830357304277));
#28629=CARTESIAN_POINT('Ctrl Pts',(-2.19552129483562,1.,-0.0713863779524629));
#28630=CARTESIAN_POINT('Ctrl Pts',(-2.19777582085261,1.,-0.0701143536324927));
#28631=CARTESIAN_POINT('Ctrl Pts',(-2.19890268624765,1.,-0.0694764450219585));
#28632=CARTESIAN_POINT('',(-1.74236521665491,0.,-0.163289472382896));
#28633=CARTESIAN_POINT('Origin',(0.,0.,0.));
#28634=CARTESIAN_POINT('',(-1.7075470150345,1.,-0.383122945602004));
#28635=CARTESIAN_POINT('Origin',(0.,1.,0.));
#28636=CARTESIAN_POINT('',(-1.7075470150345,0.,-0.383122945602004));
#28637=CARTESIAN_POINT('Ctrl Pts',(-2.11275013067528,-1.,-0.61342227326009));
#28638=CARTESIAN_POINT('Ctrl Pts',(-2.11275013067528,1.,-0.61342227326009));
#28639=CARTESIAN_POINT('Ctrl Pts',(-2.11187554260142,-1.,-0.61246736556225));
#28640=CARTESIAN_POINT('Ctrl Pts',(-2.11187554260142,1.,-0.61246736556225));
#28641=CARTESIAN_POINT('Ctrl Pts',(-2.11012443807661,-1.,-0.610560911691113));
#28642=CARTESIAN_POINT('Ctrl Pts',(-2.11012443807661,1.,-0.610560911691113));
#28643=CARTESIAN_POINT('Ctrl Pts',(-2.10749199615859,-1.,-0.607711315456826));
#28644=CARTESIAN_POINT('Ctrl Pts',(-2.10749199615859,1.,-0.607711315456826));
#28645=CARTESIAN_POINT('Ctrl Pts',(-2.10397049887709,-1.,-0.603932030738212));
#28646=CARTESIAN_POINT('Ctrl Pts',(-2.10397049887709,1.,-0.603932030738212));
#28647=CARTESIAN_POINT('Ctrl Pts',(-2.09954930865331,-1.,-0.599241616422144));
#28648=CARTESIAN_POINT('Ctrl Pts',(-2.09954930865331,1.,-0.599241616422144));
#28649=CARTESIAN_POINT('Ctrl Pts',(-2.09510876220501,-1.,-0.594585006052823));
#28650=CARTESIAN_POINT('Ctrl Pts',(-2.09510876220501,1.,-0.594585006052823));
#28651=CARTESIAN_POINT('Ctrl Pts',(-2.09064881812053,-1.,-0.589962365403189));
#28652=CARTESIAN_POINT('Ctrl Pts',(-2.09064881812053,1.,-0.589962365403189));
#28653=CARTESIAN_POINT('Ctrl Pts',(-2.086169437277,-1.,-0.585373918990895));
#28654=CARTESIAN_POINT('Ctrl Pts',(-2.086169437277,1.,-0.585373918990895));
#28655=CARTESIAN_POINT('Ctrl Pts',(-2.08167059018138,-1.,-0.580819952107257));
#28656=CARTESIAN_POINT('Ctrl Pts',(-2.08167059018138,1.,-0.580819952107257));
#28657=CARTESIAN_POINT('Ctrl Pts',(-2.07715226767361,-1.,-0.576300797416274));
#28658=CARTESIAN_POINT('Ctrl Pts',(-2.07715226767361,1.,-0.576300797416274));
#28659=CARTESIAN_POINT('Ctrl Pts',(-2.07261449292757,-1.,-0.571816823242411));
#28660=CARTESIAN_POINT('Ctrl Pts',(-2.07261449292757,1.,-0.571816823242411));
#28661=CARTESIAN_POINT('Ctrl Pts',(-2.06805732997383,-1.,-0.567368421181229));
#28662=CARTESIAN_POINT('Ctrl Pts',(-2.06805732997383,1.,-0.567368421181229));
#28663=CARTESIAN_POINT('Ctrl Pts',(-2.06348090160697,-1.,-0.562955993082574));
#28664=CARTESIAN_POINT('Ctrl Pts',(-2.06348090160697,1.,-0.562955993082574));
#28665=CARTESIAN_POINT('Ctrl Pts',(-2.05888537756571,-1.,-0.558579940185467));
#28666=CARTESIAN_POINT('Ctrl Pts',(-2.05888537756571,1.,-0.558579940185467));
#28667=CARTESIAN_POINT('Ctrl Pts',(-2.05427091604482,-1.,-0.554240657464109));
#28668=CARTESIAN_POINT('Ctrl Pts',(-2.05427091604482,1.,-0.554240657464109));
#28669=CARTESIAN_POINT('Ctrl Pts',(-2.04963761077974,-1.,-0.549938525150342));
#28670=CARTESIAN_POINT('Ctrl Pts',(-2.04963761077974,1.,-0.549938525150342));
#28671=CARTESIAN_POINT('Ctrl Pts',(-2.0449854471456,-1.,-0.545673903817348));
#28672=CARTESIAN_POINT('Ctrl Pts',(-2.0449854471456,1.,-0.545673903817348));
#28673=CARTESIAN_POINT('Ctrl Pts',(-2.0403142269048,-1.,-0.54144712061552));
#28674=CARTESIAN_POINT('Ctrl Pts',(-2.0403142269048,1.,-0.54144712061552));
#28675=CARTESIAN_POINT('Ctrl Pts',(-2.03562362953993,-1.,-0.537258489833134));
#28676=CARTESIAN_POINT('Ctrl Pts',(-2.03562362953993,1.,-0.537258489833134));
#28677=CARTESIAN_POINT('Ctrl Pts',(-2.03091336214401,-1.,-0.533108355132905));
#28678=CARTESIAN_POINT('Ctrl Pts',(-2.03091336214401,1.,-0.533108355132905));
#28679=CARTESIAN_POINT('Ctrl Pts',(-2.02618329083289,-1.,-0.52899712724191));
#28680=CARTESIAN_POINT('Ctrl Pts',(-2.02618329083289,1.,-0.52899712724191));
#28681=CARTESIAN_POINT('Ctrl Pts',(-2.02143356304712,-1.,-0.524925318333518));
#28682=CARTESIAN_POINT('Ctrl Pts',(-2.02143356304712,1.,-0.524925318333518));
#28683=CARTESIAN_POINT('Ctrl Pts',(-2.01666477917305,-1.,-0.520893590399428));
#28684=CARTESIAN_POINT('Ctrl Pts',(-2.01666477917305,1.,-0.520893590399428));
#28685=CARTESIAN_POINT('Ctrl Pts',(-2.01187773939257,-1.,-0.516902681728733));
#28686=CARTESIAN_POINT('Ctrl Pts',(-2.01187773939257,1.,-0.516902681728733));
#28687=CARTESIAN_POINT('Ctrl Pts',(-2.00707309946955,-1.,-0.512953306961813));
#28688=CARTESIAN_POINT('Ctrl Pts',(-2.00707309946955,1.,-0.512953306961813));
#28689=CARTESIAN_POINT('Ctrl Pts',(-2.00225107134733,-1.,-0.509046069886152));
#28690=CARTESIAN_POINT('Ctrl Pts',(-2.00225107134733,1.,-0.509046069886152));
#28691=CARTESIAN_POINT('Ctrl Pts',(-1.99741107463567,-1.,-0.505181361323011));
#28692=CARTESIAN_POINT('Ctrl Pts',(-1.99741107463567,1.,-0.505181361323011));
#28693=CARTESIAN_POINT('Ctrl Pts',(-1.9925514912615,-1.,-0.501359287727129));
#28694=CARTESIAN_POINT('Ctrl Pts',(-1.9925514912615,1.,-0.501359287727129));
#28695=CARTESIAN_POINT('Ctrl Pts',(-1.98767044752929,-1.,-0.497579909545564));
#28696=CARTESIAN_POINT('Ctrl Pts',(-1.98767044752929,1.,-0.497579909545564));
#28697=CARTESIAN_POINT('Ctrl Pts',(-1.9827665876182,-1.,-0.493843476541492));
#28698=CARTESIAN_POINT('Ctrl Pts',(-1.9827665876182,1.,-0.493843476541492));
#28699=CARTESIAN_POINT('Ctrl Pts',(-1.97783973019229,-1.,-0.490150627860955));
#28700=CARTESIAN_POINT('Ctrl Pts',(-1.97783973019229,1.,-0.490150627860955));
#28701=CARTESIAN_POINT('Ctrl Pts',(-1.97289186263272,-1.,-0.486502692907661));
#28702=CARTESIAN_POINT('Ctrl Pts',(-1.97289186263272,1.,-0.486502692907661));
#28703=CARTESIAN_POINT('Ctrl Pts',(-1.96792703422358,-1.,-0.482901662120686));
#28704=CARTESIAN_POINT('Ctrl Pts',(-1.96792703422358,1.,-0.482901662120686));
#28705=CARTESIAN_POINT('Ctrl Pts',(-1.96294933055938,-1.,-0.479349583074846));
#28706=CARTESIAN_POINT('Ctrl Pts',(-1.96294933055938,1.,-0.479349583074846));
#28707=CARTESIAN_POINT('Ctrl Pts',(-1.95796111148175,-1.,-0.475848034683171));
#28708=CARTESIAN_POINT('Ctrl Pts',(-1.95796111148175,1.,-0.475848034683171));
#28709=CARTESIAN_POINT('Ctrl Pts',(-1.95296148278136,-1.,-0.472397672264079));
#28710=CARTESIAN_POINT('Ctrl Pts',(-1.95296148278136,1.,-0.472397672264079));
#28711=CARTESIAN_POINT('Ctrl Pts',(-1.94794381136524,-1.,-0.468997482913158));
#28712=CARTESIAN_POINT('Ctrl Pts',(-1.94794381136524,1.,-0.468997482913158));
#28713=CARTESIAN_POINT('Ctrl Pts',(-1.94289794196205,-1.,-0.465645462026064));
#28714=CARTESIAN_POINT('Ctrl Pts',(-1.94289794196205,1.,-0.465645462026064));
#28715=CARTESIAN_POINT('Ctrl Pts',(-1.93781486640834,-1.,-0.462340031009087));
#28716=CARTESIAN_POINT('Ctrl Pts',(-1.93781486640834,1.,-0.462340031009087));
#28717=CARTESIAN_POINT('Ctrl Pts',(-1.93269066517936,-1.,-0.459081234547931));
#28718=CARTESIAN_POINT('Ctrl Pts',(-1.93269066517936,1.,-0.459081234547931));
#28719=CARTESIAN_POINT('Ctrl Pts',(-1.92753067150461,-1.,-0.455872005174335));
#28720=CARTESIAN_POINT('Ctrl Pts',(-1.92753067150461,1.,-0.455872005174335));
#28721=CARTESIAN_POINT('Ctrl Pts',(-1.9223538064847,-1.,-0.452719478359356));
#28722=CARTESIAN_POINT('Ctrl Pts',(-1.9223538064847,1.,-0.452719478359356));
#28723=CARTESIAN_POINT('Ctrl Pts',(-1.91718342555717,-1.,-0.449632260106572));
#28724=CARTESIAN_POINT('Ctrl Pts',(-1.91718342555717,1.,-0.449632260106572));
#28725=CARTESIAN_POINT('Ctrl Pts',(-1.91203699981095,-1.,-0.446617343485651));
#28726=CARTESIAN_POINT('Ctrl Pts',(-1.91203699981095,1.,-0.446617343485651));
#28727=CARTESIAN_POINT('Ctrl Pts',(-1.90691756144906,-1.,-0.44367755684917));
#28728=CARTESIAN_POINT('Ctrl Pts',(-1.90691756144906,1.,-0.44367755684917));
#28729=CARTESIAN_POINT('Ctrl Pts',(-1.90180124389137,-1.,-0.44080783370416));
#28730=CARTESIAN_POINT('Ctrl Pts',(-1.90180124389137,1.,-0.44080783370416));
#28731=CARTESIAN_POINT('Ctrl Pts',(-1.89663648956549,-1.,-0.437995003948443));
#28732=CARTESIAN_POINT('Ctrl Pts',(-1.89663648956549,1.,-0.437995003948443));
#28733=CARTESIAN_POINT('Ctrl Pts',(-1.89136993975585,-1.,-0.43522566096358));
#28734=CARTESIAN_POINT('Ctrl Pts',(-1.89136993975585,1.,-0.43522566096358));
#28735=CARTESIAN_POINT('Ctrl Pts',(-1.88596913666828,-1.,-0.432493038548833));
#28736=CARTESIAN_POINT('Ctrl Pts',(-1.88596913666828,1.,-0.432493038548833));
#28737=CARTESIAN_POINT('Ctrl Pts',(-1.88044229001778,-1.,-0.429803062482217));
#28738=CARTESIAN_POINT('Ctrl Pts',(-1.88044229001778,1.,-0.429803062482217));
#28739=CARTESIAN_POINT('Ctrl Pts',(-1.87486989291333,-1.,-0.427183828518743));
#28740=CARTESIAN_POINT('Ctrl Pts',(-1.87486989291333,1.,-0.427183828518743));
#28741=CARTESIAN_POINT('Ctrl Pts',(-1.8693780394412,-1.,-0.424678177290876));
#28742=CARTESIAN_POINT('Ctrl Pts',(-1.8693780394412,1.,-0.424678177290876));
#28743=CARTESIAN_POINT('Ctrl Pts',(-1.86408083333863,-1.,-0.422327307417884));
#28744=CARTESIAN_POINT('Ctrl Pts',(-1.86408083333863,1.,-0.422327307417884));
#28745=CARTESIAN_POINT('Ctrl Pts',(-1.8590328109667,-1.,-0.420157287975583));
#28746=CARTESIAN_POINT('Ctrl Pts',(-1.8590328109667,1.,-0.420157287975583));
#28747=CARTESIAN_POINT('Ctrl Pts',(-1.8541763285645,-1.,-0.418164129144045));
#28748=CARTESIAN_POINT('Ctrl Pts',(-1.8541763285645,1.,-0.418164129144045));
#28749=CARTESIAN_POINT('Ctrl Pts',(-1.84929312930314,-1.,-0.416300022039885));
#28750=CARTESIAN_POINT('Ctrl Pts',(-1.84929312930314,1.,-0.416300022039885));
#28751=CARTESIAN_POINT('Ctrl Pts',(-1.84405757074218,-1.,-0.414487438255542));
#28752=CARTESIAN_POINT('Ctrl Pts',(-1.84405757074218,1.,-0.414487438255542));
#28753=CARTESIAN_POINT('Ctrl Pts',(-1.8380895347617,-1.,-0.412633125322945));
#28754=CARTESIAN_POINT('Ctrl Pts',(-1.8380895347617,1.,-0.412633125322945));
#28755=CARTESIAN_POINT('Ctrl Pts',(-1.83100408895047,-1.,-0.410641256301276));
#28756=CARTESIAN_POINT('Ctrl Pts',(-1.83100408895047,1.,-0.410641256301276));
#28757=CARTESIAN_POINT('Ctrl Pts',(-1.82247022677562,-1.,-0.408428948106227));
#28758=CARTESIAN_POINT('Ctrl Pts',(-1.82247022677562,1.,-0.408428948106227));
#28759=CARTESIAN_POINT('Ctrl Pts',(-1.81223801812013,-1.,-0.405933518407175));
#28760=CARTESIAN_POINT('Ctrl Pts',(-1.81223801812013,1.,-0.405933518407175));
#28761=CARTESIAN_POINT('Ctrl Pts',(-1.80012077173238,-1.,-0.403107976163396));
#28762=CARTESIAN_POINT('Ctrl Pts',(-1.80012077173238,1.,-0.403107976163396));
#28763=CARTESIAN_POINT('Ctrl Pts',(-1.78598826343754,-1.,-0.399919403774155));
#28764=CARTESIAN_POINT('Ctrl Pts',(-1.78598826343754,1.,-0.399919403774155));
#28765=CARTESIAN_POINT('Ctrl Pts',(-1.76975560043442,-1.,-0.396346196110688));
#28766=CARTESIAN_POINT('Ctrl Pts',(-1.76975560043442,1.,-0.396346196110688));
#28767=CARTESIAN_POINT('Ctrl Pts',(-1.75137405310193,-1.,-0.392375812285395));
#28768=CARTESIAN_POINT('Ctrl Pts',(-1.75137405310193,1.,-0.392375812285395));
#28769=CARTESIAN_POINT('Ctrl Pts',(-1.73493170972829,-1.,-0.388877023502615));
#28770=CARTESIAN_POINT('Ctrl Pts',(-1.73493170972829,1.,-0.388877023502615));
#28771=CARTESIAN_POINT('Ctrl Pts',(-1.72162022244582,-1.,-0.386070790323281));
#28772=CARTESIAN_POINT('Ctrl Pts',(-1.72162022244582,1.,-0.386070790323281));
#28773=CARTESIAN_POINT('Ctrl Pts',(-1.71231062891398,-1.,-0.384119047314215));
#28774=CARTESIAN_POINT('Ctrl Pts',(-1.71231062891398,1.,-0.384119047314215));
#28775=CARTESIAN_POINT('Ctrl Pts',(-1.7075470150345,-1.,-0.383122945602004));
#28776=CARTESIAN_POINT('Ctrl Pts',(-1.7075470150345,1.,-0.383122945602004));
#28777=CARTESIAN_POINT('',(-2.11275013067528,1.,-0.61342227326009));
#28778=CARTESIAN_POINT('Ctrl Pts',(-2.11275013067528,1.,-0.61342227326009));
#28779=CARTESIAN_POINT('Ctrl Pts',(-2.11187554260142,1.,-0.61246736556225));
#28780=CARTESIAN_POINT('Ctrl Pts',(-2.11012443807661,1.,-0.610560911691113));
#28781=CARTESIAN_POINT('Ctrl Pts',(-2.10749199615859,1.,-0.607711315456826));
#28782=CARTESIAN_POINT('Ctrl Pts',(-2.10397049887709,1.,-0.603932030738212));
#28783=CARTESIAN_POINT('Ctrl Pts',(-2.09954930865331,1.,-0.599241616422144));
#28784=CARTESIAN_POINT('Ctrl Pts',(-2.09510876220501,1.,-0.594585006052823));
#28785=CARTESIAN_POINT('Ctrl Pts',(-2.09064881812053,1.,-0.589962365403189));
#28786=CARTESIAN_POINT('Ctrl Pts',(-2.086169437277,1.,-0.585373918990895));
#28787=CARTESIAN_POINT('Ctrl Pts',(-2.08167059018138,1.,-0.580819952107257));
#28788=CARTESIAN_POINT('Ctrl Pts',(-2.07715226767361,1.,-0.576300797416274));
#28789=CARTESIAN_POINT('Ctrl Pts',(-2.07261449292757,1.,-0.571816823242411));
#28790=CARTESIAN_POINT('Ctrl Pts',(-2.06805732997383,1.,-0.567368421181229));
#28791=CARTESIAN_POINT('Ctrl Pts',(-2.06348090160697,1.,-0.562955993082574));
#28792=CARTESIAN_POINT('Ctrl Pts',(-2.05888537756571,1.,-0.558579940185467));
#28793=CARTESIAN_POINT('Ctrl Pts',(-2.05427091604482,1.,-0.554240657464109));
#28794=CARTESIAN_POINT('Ctrl Pts',(-2.04963761077974,1.,-0.549938525150342));
#28795=CARTESIAN_POINT('Ctrl Pts',(-2.0449854471456,1.,-0.545673903817348));
#28796=CARTESIAN_POINT('Ctrl Pts',(-2.0403142269048,1.,-0.54144712061552));
#28797=CARTESIAN_POINT('Ctrl Pts',(-2.03562362953993,1.,-0.537258489833134));
#28798=CARTESIAN_POINT('Ctrl Pts',(-2.03091336214401,1.,-0.533108355132905));
#28799=CARTESIAN_POINT('Ctrl Pts',(-2.02618329083289,1.,-0.52899712724191));
#28800=CARTESIAN_POINT('Ctrl Pts',(-2.02143356304712,1.,-0.524925318333518));
#28801=CARTESIAN_POINT('Ctrl Pts',(-2.01666477917305,1.,-0.520893590399428));
#28802=CARTESIAN_POINT('Ctrl Pts',(-2.01187773939257,1.,-0.516902681728733));
#28803=CARTESIAN_POINT('Ctrl Pts',(-2.00707309946955,1.,-0.512953306961813));
#28804=CARTESIAN_POINT('Ctrl Pts',(-2.00225107134733,1.,-0.509046069886152));
#28805=CARTESIAN_POINT('Ctrl Pts',(-1.99741107463567,1.,-0.505181361323011));
#28806=CARTESIAN_POINT('Ctrl Pts',(-1.9925514912615,1.,-0.501359287727129));
#28807=CARTESIAN_POINT('Ctrl Pts',(-1.98767044752929,1.,-0.497579909545564));
#28808=CARTESIAN_POINT('Ctrl Pts',(-1.9827665876182,1.,-0.493843476541492));
#28809=CARTESIAN_POINT('Ctrl Pts',(-1.97783973019229,1.,-0.490150627860955));
#28810=CARTESIAN_POINT('Ctrl Pts',(-1.97289186263272,1.,-0.486502692907661));
#28811=CARTESIAN_POINT('Ctrl Pts',(-1.96792703422358,1.,-0.482901662120686));
#28812=CARTESIAN_POINT('Ctrl Pts',(-1.96294933055938,1.,-0.479349583074846));
#28813=CARTESIAN_POINT('Ctrl Pts',(-1.95796111148175,1.,-0.475848034683171));
#28814=CARTESIAN_POINT('Ctrl Pts',(-1.95296148278136,1.,-0.472397672264079));
#28815=CARTESIAN_POINT('Ctrl Pts',(-1.94794381136524,1.,-0.468997482913158));
#28816=CARTESIAN_POINT('Ctrl Pts',(-1.94289794196205,1.,-0.465645462026064));
#28817=CARTESIAN_POINT('Ctrl Pts',(-1.93781486640834,1.,-0.462340031009087));
#28818=CARTESIAN_POINT('Ctrl Pts',(-1.93269066517936,1.,-0.459081234547931));
#28819=CARTESIAN_POINT('Ctrl Pts',(-1.92753067150461,1.,-0.455872005174335));
#28820=CARTESIAN_POINT('Ctrl Pts',(-1.9223538064847,1.,-0.452719478359356));
#28821=CARTESIAN_POINT('Ctrl Pts',(-1.91718342555717,1.,-0.449632260106572));
#28822=CARTESIAN_POINT('Ctrl Pts',(-1.91203699981095,1.,-0.446617343485651));
#28823=CARTESIAN_POINT('Ctrl Pts',(-1.90691756144906,1.,-0.44367755684917));
#28824=CARTESIAN_POINT('Ctrl Pts',(-1.90180124389137,1.,-0.44080783370416));
#28825=CARTESIAN_POINT('Ctrl Pts',(-1.89663648956549,1.,-0.437995003948443));
#28826=CARTESIAN_POINT('Ctrl Pts',(-1.89136993975585,1.,-0.43522566096358));
#28827=CARTESIAN_POINT('Ctrl Pts',(-1.88596913666828,1.,-0.432493038548833));
#28828=CARTESIAN_POINT('Ctrl Pts',(-1.88044229001778,1.,-0.429803062482217));
#28829=CARTESIAN_POINT('Ctrl Pts',(-1.87486989291333,1.,-0.427183828518743));
#28830=CARTESIAN_POINT('Ctrl Pts',(-1.8693780394412,1.,-0.424678177290876));
#28831=CARTESIAN_POINT('Ctrl Pts',(-1.86408083333863,1.,-0.422327307417884));
#28832=CARTESIAN_POINT('Ctrl Pts',(-1.8590328109667,1.,-0.420157287975583));
#28833=CARTESIAN_POINT('Ctrl Pts',(-1.8541763285645,1.,-0.418164129144045));
#28834=CARTESIAN_POINT('Ctrl Pts',(-1.84929312930314,1.,-0.416300022039885));
#28835=CARTESIAN_POINT('Ctrl Pts',(-1.84405757074218,1.,-0.414487438255542));
#28836=CARTESIAN_POINT('Ctrl Pts',(-1.8380895347617,1.,-0.412633125322945));
#28837=CARTESIAN_POINT('Ctrl Pts',(-1.83100408895047,1.,-0.410641256301276));
#28838=CARTESIAN_POINT('Ctrl Pts',(-1.82247022677562,1.,-0.408428948106227));
#28839=CARTESIAN_POINT('Ctrl Pts',(-1.81223801812013,1.,-0.405933518407175));
#28840=CARTESIAN_POINT('Ctrl Pts',(-1.80012077173238,1.,-0.403107976163396));
#28841=CARTESIAN_POINT('Ctrl Pts',(-1.78598826343754,1.,-0.399919403774155));
#28842=CARTESIAN_POINT('Ctrl Pts',(-1.76975560043442,1.,-0.396346196110688));
#28843=CARTESIAN_POINT('Ctrl Pts',(-1.75137405310193,1.,-0.392375812285395));
#28844=CARTESIAN_POINT('Ctrl Pts',(-1.73493170972829,1.,-0.388877023502615));
#28845=CARTESIAN_POINT('Ctrl Pts',(-1.72162022244582,1.,-0.386070790323281));
#28846=CARTESIAN_POINT('Ctrl Pts',(-1.71231062891398,1.,-0.384119047314215));
#28847=CARTESIAN_POINT('Ctrl Pts',(-1.7075470150345,1.,-0.383122945602004));
#28848=CARTESIAN_POINT('',(-2.11275013067528,0.,-0.61342227326009));
#28849=CARTESIAN_POINT('Origin',(-2.0698113262342,0.,-0.745574324794401));
#28850=CARTESIAN_POINT('',(-2.0698113262342,1.,-0.745574324794401));
#28851=CARTESIAN_POINT('',(-2.11275013067528,1.,-0.61342227326009));
#28852=CARTESIAN_POINT('',(-2.0698113262342,0.,-0.745574324794401));
#28853=CARTESIAN_POINT('Ctrl Pts',(-1.60662857109684,-1.,-0.693717979106306));
#28854=CARTESIAN_POINT('Ctrl Pts',(-1.60662857109684,1.,-0.693717979106306));
#28855=CARTESIAN_POINT('Ctrl Pts',(-1.61106790958151,-1.,-0.695712097881194));
#28856=CARTESIAN_POINT('Ctrl Pts',(-1.61106790958151,1.,-0.695712097881194));
#28857=CARTESIAN_POINT('Ctrl Pts',(-1.61974673472612,-1.,-0.699605146405088));
#28858=CARTESIAN_POINT('Ctrl Pts',(-1.61974673472612,1.,-0.699605146405088));
#28859=CARTESIAN_POINT('Ctrl Pts',(-1.63216541664676,-1.,-0.705159151988319));
#28860=CARTESIAN_POINT('Ctrl Pts',(-1.63216541664676,1.,-0.705159151988319));
#28861=CARTESIAN_POINT('Ctrl Pts',(-1.64752408832016,-1.,-0.711993139355394));
#28862=CARTESIAN_POINT('Ctrl Pts',(-1.64752408832016,1.,-0.711993139355394));
#28863=CARTESIAN_POINT('Ctrl Pts',(-1.6647288055568,-1.,-0.719585433804282));
#28864=CARTESIAN_POINT('Ctrl Pts',(-1.6647288055568,1.,-0.719585433804282));
#28865=CARTESIAN_POINT('Ctrl Pts',(-1.67996158455503,-1.,-0.726235967997433));
#28866=CARTESIAN_POINT('Ctrl Pts',(-1.67996158455503,1.,-0.726235967997433));
#28867=CARTESIAN_POINT('Ctrl Pts',(-1.69326921975743,-1.,-0.731963238697195));
#28868=CARTESIAN_POINT('Ctrl Pts',(-1.69326921975743,1.,-0.731963238697195));
#28869=CARTESIAN_POINT('Ctrl Pts',(-1.70473309006121,-1.,-0.736799665724771));
#28870=CARTESIAN_POINT('Ctrl Pts',(-1.70473309006121,1.,-0.736799665724771));
#28871=CARTESIAN_POINT('Ctrl Pts',(-1.71447789751927,-1.,-0.740795162032087));
#28872=CARTESIAN_POINT('Ctrl Pts',(-1.71447789751927,1.,-0.740795162032087));
#28873=CARTESIAN_POINT('Ctrl Pts',(-1.7226822991693,-1.,-0.744021445433764));
#28874=CARTESIAN_POINT('Ctrl Pts',(-1.7226822991693,1.,-0.744021445433764));
#28875=CARTESIAN_POINT('Ctrl Pts',(-1.72958533647399,-1.,-0.746574710096436));
#28876=CARTESIAN_POINT('Ctrl Pts',(-1.72958533647399,1.,-0.746574710096436));
#28877=CARTESIAN_POINT('Ctrl Pts',(-1.73550351679848,-1.,-0.748582462954854));
#28878=CARTESIAN_POINT('Ctrl Pts',(-1.73550351679848,1.,-0.748582462954854));
#28879=CARTESIAN_POINT('Ctrl Pts',(-1.74080458266705,-1.,-0.75019343597954));
#28880=CARTESIAN_POINT('Ctrl Pts',(-1.74080458266705,1.,-0.75019343597954));
#28881=CARTESIAN_POINT('Ctrl Pts',(-1.74585086852298,-1.,-0.751555614163629));
#28882=CARTESIAN_POINT('Ctrl Pts',(-1.74585086852298,1.,-0.751555614163629));
#28883=CARTESIAN_POINT('Ctrl Pts',(-1.75095139468809,-1.,-0.752797683531377));
#28884=CARTESIAN_POINT('Ctrl Pts',(-1.75095139468809,1.,-0.752797683531377));
#28885=CARTESIAN_POINT('Ctrl Pts',(-1.75631083600175,-1.,-0.75400925402848));
#28886=CARTESIAN_POINT('Ctrl Pts',(-1.75631083600175,1.,-0.75400925402848));
#28887=CARTESIAN_POINT('Ctrl Pts',(-1.7619781724032,-1.,-0.755220979975262));
#28888=CARTESIAN_POINT('Ctrl Pts',(-1.7619781724032,1.,-0.755220979975262));
#28889=CARTESIAN_POINT('Ctrl Pts',(-1.76789396003141,-1.,-0.756421896028403));
#28890=CARTESIAN_POINT('Ctrl Pts',(-1.76789396003141,1.,-0.756421896028403));
#28891=CARTESIAN_POINT('Ctrl Pts',(-1.77394167108342,-1.,-0.757578264077238));
#28892=CARTESIAN_POINT('Ctrl Pts',(-1.77394167108342,1.,-0.757578264077238));
#28893=CARTESIAN_POINT('Ctrl Pts',(-1.77999411220912,-1.,-0.75865062667738));
#28894=CARTESIAN_POINT('Ctrl Pts',(-1.77999411220912,1.,-0.75865062667738));
#28895=CARTESIAN_POINT('Ctrl Pts',(-1.78596964884526,-1.,-0.759614401109868));
#28896=CARTESIAN_POINT('Ctrl Pts',(-1.78596964884526,1.,-0.759614401109868));
#28897=CARTESIAN_POINT('Ctrl Pts',(-1.79185815610802,-1.,-0.760469555880425));
#28898=CARTESIAN_POINT('Ctrl Pts',(-1.79185815610802,1.,-0.760469555880425));
#28899=CARTESIAN_POINT('Ctrl Pts',(-1.79768986997735,-1.,-0.761229695230359));
#28900=CARTESIAN_POINT('Ctrl Pts',(-1.79768986997735,1.,-0.761229695230359));
#28901=CARTESIAN_POINT('Ctrl Pts',(-1.80351583877334,-1.,-0.761915336443515));
#28902=CARTESIAN_POINT('Ctrl Pts',(-1.80351583877334,1.,-0.761915336443515));
#28903=CARTESIAN_POINT('Ctrl Pts',(-1.80938551463989,-1.,-0.762546129464036));
#28904=CARTESIAN_POINT('Ctrl Pts',(-1.80938551463989,1.,-0.762546129464036));
#28905=CARTESIAN_POINT('Ctrl Pts',(-1.81532118405566,-1.,-0.763132003836783));
#28906=CARTESIAN_POINT('Ctrl Pts',(-1.81532118405566,1.,-0.763132003836783));
#28907=CARTESIAN_POINT('Ctrl Pts',(-1.82131873145297,-1.,-0.763673465462854));
#28908=CARTESIAN_POINT('Ctrl Pts',(-1.82131873145297,1.,-0.763673465462854));
#28909=CARTESIAN_POINT('Ctrl Pts',(-1.8273599120008,-1.,-0.764165902606055));
#28910=CARTESIAN_POINT('Ctrl Pts',(-1.8273599120008,1.,-0.764165902606055));
#28911=CARTESIAN_POINT('Ctrl Pts',(-1.8334207722714,-1.,-0.764602549687845));
#28912=CARTESIAN_POINT('Ctrl Pts',(-1.8334207722714,1.,-0.764602549687845));
#28913=CARTESIAN_POINT('Ctrl Pts',(-1.83948181064823,-1.,-0.764978057881687));
#28914=CARTESIAN_POINT('Ctrl Pts',(-1.83948181064823,1.,-0.764978057881687));
#28915=CARTESIAN_POINT('Ctrl Pts',(-1.8455369887591,-1.,-0.765291664861971));
#28916=CARTESIAN_POINT('Ctrl Pts',(-1.8455369887591,1.,-0.765291664861971));
#28917=CARTESIAN_POINT('Ctrl Pts',(-1.85158945130054,-1.,-0.765545710619023));
#28918=CARTESIAN_POINT('Ctrl Pts',(-1.85158945130054,1.,-0.765545710619023));
#28919=CARTESIAN_POINT('Ctrl Pts',(-1.85764741390391,-1.,-0.765744212909305));
#28920=CARTESIAN_POINT('Ctrl Pts',(-1.85764741390391,1.,-0.765744212909305));
#28921=CARTESIAN_POINT('Ctrl Pts',(-1.86372027063314,-1.,-0.765891519092557));
#28922=CARTESIAN_POINT('Ctrl Pts',(-1.86372027063314,1.,-0.765891519092557));
#28923=CARTESIAN_POINT('Ctrl Pts',(-1.86981398314345,-1.,-0.765990708546111));
#28924=CARTESIAN_POINT('Ctrl Pts',(-1.86981398314345,1.,-0.765990708546111));
#28925=CARTESIAN_POINT('Ctrl Pts',(-1.87592888967886,-1.,-0.766042837036759));
#28926=CARTESIAN_POINT('Ctrl Pts',(-1.87592888967886,1.,-0.766042837036759));
#28927=CARTESIAN_POINT('Ctrl Pts',(-1.88206215302561,-1.,-0.766047794851868));
#28928=CARTESIAN_POINT('Ctrl Pts',(-1.88206215302561,1.,-0.766047794851868));
#28929=CARTESIAN_POINT('Ctrl Pts',(-1.88820926433409,-1.,-0.76600483706209));
#28930=CARTESIAN_POINT('Ctrl Pts',(-1.88820926433409,1.,-0.76600483706209));
#28931=CARTESIAN_POINT('Ctrl Pts',(-1.89436577771389,-1.,-0.765913193856979));
#28932=CARTESIAN_POINT('Ctrl Pts',(-1.89436577771389,1.,-0.765913193856979));
#28933=CARTESIAN_POINT('Ctrl Pts',(-1.90052930393599,-1.,-0.765772772593395));
#28934=CARTESIAN_POINT('Ctrl Pts',(-1.90052930393599,1.,-0.765772772593395));
#28935=CARTESIAN_POINT('Ctrl Pts',(-1.90669961402362,-1.,-0.765584196937936));
#28936=CARTESIAN_POINT('Ctrl Pts',(-1.90669961402362,1.,-0.765584196937936));
#28937=CARTESIAN_POINT('Ctrl Pts',(-1.91287765805174,-1.,-0.765348465884739));
#28938=CARTESIAN_POINT('Ctrl Pts',(-1.91287765805174,1.,-0.765348465884739));
#28939=CARTESIAN_POINT('Ctrl Pts',(-1.91906491634197,-1.,-0.765066729667095));
#28940=CARTESIAN_POINT('Ctrl Pts',(-1.91906491634197,1.,-0.765066729667095));
#28941=CARTESIAN_POINT('Ctrl Pts',(-1.92526263537041,-1.,-0.764740025488189));
#28942=CARTESIAN_POINT('Ctrl Pts',(-1.92526263537041,1.,-0.764740025488189));
#28943=CARTESIAN_POINT('Ctrl Pts',(-1.93147105496367,-1.,-0.764369010673889));
#28944=CARTESIAN_POINT('Ctrl Pts',(-1.93147105496367,1.,-0.764369010673889));
#28945=CARTESIAN_POINT('Ctrl Pts',(-1.93768964875867,-1.,-0.763954049121393));
#28946=CARTESIAN_POINT('Ctrl Pts',(-1.93768964875867,1.,-0.763954049121393));
#28947=CARTESIAN_POINT('Ctrl Pts',(-1.94391746617626,-1.,-0.76349533353858));
#28948=CARTESIAN_POINT('Ctrl Pts',(-1.94391746617626,1.,-0.76349533353858));
#28949=CARTESIAN_POINT('Ctrl Pts',(-1.95015342590025,-1.,-0.762992990878774));
#28950=CARTESIAN_POINT('Ctrl Pts',(-1.95015342590025,1.,-0.762992990878774));
#28951=CARTESIAN_POINT('Ctrl Pts',(-1.95639665309893,-1.,-0.762447203806263));
#28952=CARTESIAN_POINT('Ctrl Pts',(-1.95639665309893,1.,-0.762447203806263));
#28953=CARTESIAN_POINT('Ctrl Pts',(-1.96264672744229,-1.,-0.761858300014575));
#28954=CARTESIAN_POINT('Ctrl Pts',(-1.96264672744229,1.,-0.761858300014575));
#28955=CARTESIAN_POINT('Ctrl Pts',(-1.96890351582545,-1.,-0.761226690483986));
#28956=CARTESIAN_POINT('Ctrl Pts',(-1.96890351582545,1.,-0.761226690483986));
#28957=CARTESIAN_POINT('Ctrl Pts',(-1.97516705321521,-1.,-0.760552825409855));
#28958=CARTESIAN_POINT('Ctrl Pts',(-1.97516705321521,1.,-0.760552825409855));
#28959=CARTESIAN_POINT('Ctrl Pts',(-1.98143741418156,-1.,-0.759837147452135));
#28960=CARTESIAN_POINT('Ctrl Pts',(-1.98143741418156,1.,-0.759837147452135));
#28961=CARTESIAN_POINT('Ctrl Pts',(-1.98771456680806,-1.,-0.759080037802242));
#28962=CARTESIAN_POINT('Ctrl Pts',(-1.98771456680806,1.,-0.759080037802242));
#28963=CARTESIAN_POINT('Ctrl Pts',(-1.9939983109871,-1.,-0.758281796766377));
#28964=CARTESIAN_POINT('Ctrl Pts',(-1.9939983109871,1.,-0.758281796766377));
#28965=CARTESIAN_POINT('Ctrl Pts',(-2.00028834739072,-1.,-0.757442676862341));
#28966=CARTESIAN_POINT('Ctrl Pts',(-2.00028834739072,1.,-0.757442676862341));
#28967=CARTESIAN_POINT('Ctrl Pts',(-2.00658431587682,-1.,-0.756562904646496));
#28968=CARTESIAN_POINT('Ctrl Pts',(-2.00658431587682,1.,-0.756562904646496));
#28969=CARTESIAN_POINT('Ctrl Pts',(-2.01288584328149,-1.,-0.7556427049581));
#28970=CARTESIAN_POINT('Ctrl Pts',(-2.01288584328149,1.,-0.7556427049581));
#28971=CARTESIAN_POINT('Ctrl Pts',(-2.01919259406003,-1.,-0.75468233072352));
#28972=CARTESIAN_POINT('Ctrl Pts',(-2.01919259406003,1.,-0.75468233072352));
#28973=CARTESIAN_POINT('Ctrl Pts',(-2.02550428623587,-1.,-0.753682061113765));
#28974=CARTESIAN_POINT('Ctrl Pts',(-2.02550428623587,1.,-0.753682061113765));
#28975=CARTESIAN_POINT('Ctrl Pts',(-2.03182068456467,-1.,-0.752642180488104));
#28976=CARTESIAN_POINT('Ctrl Pts',(-2.03182068456467,1.,-0.752642180488104));
#28977=CARTESIAN_POINT('Ctrl Pts',(-2.03814160092173,-1.,-0.751562963361383));
#28978=CARTESIAN_POINT('Ctrl Pts',(-2.03814160092173,1.,-0.751562963361383));
#28979=CARTESIAN_POINT('Ctrl Pts',(-2.04446689147754,-1.,-0.750444657874758));
#28980=CARTESIAN_POINT('Ctrl Pts',(-2.04446689147754,1.,-0.750444657874758));
#28981=CARTESIAN_POINT('Ctrl Pts',(-2.05079645591606,-1.,-0.749287468663053));
#28982=CARTESIAN_POINT('Ctrl Pts',(-2.05079645591606,1.,-0.749287468663053));
#28983=CARTESIAN_POINT('Ctrl Pts',(-2.05713023030263,-1.,-0.748091554181101));
#28984=CARTESIAN_POINT('Ctrl Pts',(-2.05713023030263,1.,-0.748091554181101));
#28985=CARTESIAN_POINT('Ctrl Pts',(-2.06220058927162,-1.,-0.747103932785504));
#28986=CARTESIAN_POINT('Ctrl Pts',(-2.06220058927162,1.,-0.747103932785504));
#28987=CARTESIAN_POINT('Ctrl Pts',(-2.06600523016401,-1.,-0.746345871542695));
#28988=CARTESIAN_POINT('Ctrl Pts',(-2.06600523016401,1.,-0.746345871542695));
#28989=CARTESIAN_POINT('Ctrl Pts',(-2.06854248895575,-1.,-0.74583279137781));
#28990=CARTESIAN_POINT('Ctrl Pts',(-2.06854248895575,1.,-0.74583279137781));
#28991=CARTESIAN_POINT('Ctrl Pts',(-2.0698113262342,-1.,-0.745574324794401));
#28992=CARTESIAN_POINT('Ctrl Pts',(-2.0698113262342,1.,-0.745574324794401));
#28993=CARTESIAN_POINT('',(-1.60662857109684,1.,-0.693717979106306));
#28994=CARTESIAN_POINT('Ctrl Pts',(-1.60662857109684,1.,-0.693717979106306));
#28995=CARTESIAN_POINT('Ctrl Pts',(-1.61106790958151,1.,-0.695712097881194));
#28996=CARTESIAN_POINT('Ctrl Pts',(-1.61974673472612,1.,-0.699605146405088));
#28997=CARTESIAN_POINT('Ctrl Pts',(-1.63216541664676,1.,-0.705159151988319));
#28998=CARTESIAN_POINT('Ctrl Pts',(-1.64752408832016,1.,-0.711993139355394));
#28999=CARTESIAN_POINT('Ctrl Pts',(-1.6647288055568,1.,-0.719585433804282));
#29000=CARTESIAN_POINT('Ctrl Pts',(-1.67996158455503,1.,-0.726235967997433));
#29001=CARTESIAN_POINT('Ctrl Pts',(-1.69326921975743,1.,-0.731963238697195));
#29002=CARTESIAN_POINT('Ctrl Pts',(-1.70473309006121,1.,-0.736799665724771));
#29003=CARTESIAN_POINT('Ctrl Pts',(-1.71447789751927,1.,-0.740795162032087));
#29004=CARTESIAN_POINT('Ctrl Pts',(-1.7226822991693,1.,-0.744021445433764));
#29005=CARTESIAN_POINT('Ctrl Pts',(-1.72958533647399,1.,-0.746574710096436));
#29006=CARTESIAN_POINT('Ctrl Pts',(-1.73550351679848,1.,-0.748582462954854));
#29007=CARTESIAN_POINT('Ctrl Pts',(-1.74080458266705,1.,-0.75019343597954));
#29008=CARTESIAN_POINT('Ctrl Pts',(-1.74585086852298,1.,-0.751555614163629));
#29009=CARTESIAN_POINT('Ctrl Pts',(-1.75095139468809,1.,-0.752797683531377));
#29010=CARTESIAN_POINT('Ctrl Pts',(-1.75631083600175,1.,-0.75400925402848));
#29011=CARTESIAN_POINT('Ctrl Pts',(-1.7619781724032,1.,-0.755220979975262));
#29012=CARTESIAN_POINT('Ctrl Pts',(-1.76789396003141,1.,-0.756421896028403));
#29013=CARTESIAN_POINT('Ctrl Pts',(-1.77394167108342,1.,-0.757578264077238));
#29014=CARTESIAN_POINT('Ctrl Pts',(-1.77999411220912,1.,-0.75865062667738));
#29015=CARTESIAN_POINT('Ctrl Pts',(-1.78596964884526,1.,-0.759614401109868));
#29016=CARTESIAN_POINT('Ctrl Pts',(-1.79185815610802,1.,-0.760469555880425));
#29017=CARTESIAN_POINT('Ctrl Pts',(-1.79768986997735,1.,-0.761229695230359));
#29018=CARTESIAN_POINT('Ctrl Pts',(-1.80351583877334,1.,-0.761915336443515));
#29019=CARTESIAN_POINT('Ctrl Pts',(-1.80938551463989,1.,-0.762546129464036));
#29020=CARTESIAN_POINT('Ctrl Pts',(-1.81532118405566,1.,-0.763132003836783));
#29021=CARTESIAN_POINT('Ctrl Pts',(-1.82131873145297,1.,-0.763673465462854));
#29022=CARTESIAN_POINT('Ctrl Pts',(-1.8273599120008,1.,-0.764165902606055));
#29023=CARTESIAN_POINT('Ctrl Pts',(-1.8334207722714,1.,-0.764602549687845));
#29024=CARTESIAN_POINT('Ctrl Pts',(-1.83948181064823,1.,-0.764978057881687));
#29025=CARTESIAN_POINT('Ctrl Pts',(-1.8455369887591,1.,-0.765291664861971));
#29026=CARTESIAN_POINT('Ctrl Pts',(-1.85158945130054,1.,-0.765545710619023));
#29027=CARTESIAN_POINT('Ctrl Pts',(-1.85764741390391,1.,-0.765744212909305));
#29028=CARTESIAN_POINT('Ctrl Pts',(-1.86372027063314,1.,-0.765891519092557));
#29029=CARTESIAN_POINT('Ctrl Pts',(-1.86981398314345,1.,-0.765990708546111));
#29030=CARTESIAN_POINT('Ctrl Pts',(-1.87592888967886,1.,-0.766042837036759));
#29031=CARTESIAN_POINT('Ctrl Pts',(-1.88206215302561,1.,-0.766047794851868));
#29032=CARTESIAN_POINT('Ctrl Pts',(-1.88820926433409,1.,-0.76600483706209));
#29033=CARTESIAN_POINT('Ctrl Pts',(-1.89436577771389,1.,-0.765913193856979));
#29034=CARTESIAN_POINT('Ctrl Pts',(-1.90052930393599,1.,-0.765772772593395));
#29035=CARTESIAN_POINT('Ctrl Pts',(-1.90669961402362,1.,-0.765584196937936));
#29036=CARTESIAN_POINT('Ctrl Pts',(-1.91287765805174,1.,-0.765348465884739));
#29037=CARTESIAN_POINT('Ctrl Pts',(-1.91906491634197,1.,-0.765066729667095));
#29038=CARTESIAN_POINT('Ctrl Pts',(-1.92526263537041,1.,-0.764740025488189));
#29039=CARTESIAN_POINT('Ctrl Pts',(-1.93147105496367,1.,-0.764369010673889));
#29040=CARTESIAN_POINT('Ctrl Pts',(-1.93768964875867,1.,-0.763954049121393));
#29041=CARTESIAN_POINT('Ctrl Pts',(-1.94391746617626,1.,-0.76349533353858));
#29042=CARTESIAN_POINT('Ctrl Pts',(-1.95015342590025,1.,-0.762992990878774));
#29043=CARTESIAN_POINT('Ctrl Pts',(-1.95639665309893,1.,-0.762447203806263));
#29044=CARTESIAN_POINT('Ctrl Pts',(-1.96264672744229,1.,-0.761858300014575));
#29045=CARTESIAN_POINT('Ctrl Pts',(-1.96890351582545,1.,-0.761226690483986));
#29046=CARTESIAN_POINT('Ctrl Pts',(-1.97516705321521,1.,-0.760552825409855));
#29047=CARTESIAN_POINT('Ctrl Pts',(-1.98143741418156,1.,-0.759837147452135));
#29048=CARTESIAN_POINT('Ctrl Pts',(-1.98771456680806,1.,-0.759080037802242));
#29049=CARTESIAN_POINT('Ctrl Pts',(-1.9939983109871,1.,-0.758281796766377));
#29050=CARTESIAN_POINT('Ctrl Pts',(-2.00028834739072,1.,-0.757442676862341));
#29051=CARTESIAN_POINT('Ctrl Pts',(-2.00658431587682,1.,-0.756562904646496));
#29052=CARTESIAN_POINT('Ctrl Pts',(-2.01288584328149,1.,-0.7556427049581));
#29053=CARTESIAN_POINT('Ctrl Pts',(-2.01919259406003,1.,-0.75468233072352));
#29054=CARTESIAN_POINT('Ctrl Pts',(-2.02550428623587,1.,-0.753682061113765));
#29055=CARTESIAN_POINT('Ctrl Pts',(-2.03182068456467,1.,-0.752642180488104));
#29056=CARTESIAN_POINT('Ctrl Pts',(-2.03814160092173,1.,-0.751562963361383));
#29057=CARTESIAN_POINT('Ctrl Pts',(-2.04446689147754,1.,-0.750444657874758));
#29058=CARTESIAN_POINT('Ctrl Pts',(-2.05079645591606,1.,-0.749287468663053));
#29059=CARTESIAN_POINT('Ctrl Pts',(-2.05713023030263,1.,-0.748091554181101));
#29060=CARTESIAN_POINT('Ctrl Pts',(-2.06220058927162,1.,-0.747103932785504));
#29061=CARTESIAN_POINT('Ctrl Pts',(-2.06600523016401,1.,-0.746345871542695));
#29062=CARTESIAN_POINT('Ctrl Pts',(-2.06854248895575,1.,-0.74583279137781));
#29063=CARTESIAN_POINT('Ctrl Pts',(-2.0698113262342,1.,-0.745574324794401));
#29064=CARTESIAN_POINT('',(-1.60662857109684,0.,-0.693717979106306));
#29065=CARTESIAN_POINT('Origin',(0.,0.,0.));
#29066=CARTESIAN_POINT('',(-1.5055822144029,1.,-0.892032620296855));
#29067=CARTESIAN_POINT('Origin',(0.,1.,0.));
#29068=CARTESIAN_POINT('',(-1.5055822144029,0.,-0.892032620296855));
#29069=CARTESIAN_POINT('Ctrl Pts',(-1.81978687191668,-1.,-1.23627494547115));
#29070=CARTESIAN_POINT('Ctrl Pts',(-1.81978687191668,1.,-1.23627494547115));
#29071=CARTESIAN_POINT('Ctrl Pts',(-1.81925017193666,-1.,-1.23509651170476));
#29072=CARTESIAN_POINT('Ctrl Pts',(-1.81925017193666,1.,-1.23509651170476));
#29073=CARTESIAN_POINT('Ctrl Pts',(-1.81817389921279,-1.,-1.2327422452705));
#29074=CARTESIAN_POINT('Ctrl Pts',(-1.81817389921279,1.,-1.2327422452705));
#29075=CARTESIAN_POINT('Ctrl Pts',(-1.8165508718364,-1.,-1.2292186489137));
#29076=CARTESIAN_POINT('Ctrl Pts',(-1.8165508718364,1.,-1.2292186489137));
#29077=CARTESIAN_POINT('Ctrl Pts',(-1.81436959210434,-1.,-1.2245361330495));
#29078=CARTESIAN_POINT('Ctrl Pts',(-1.81436959210434,1.,-1.2245361330495));
#29079=CARTESIAN_POINT('Ctrl Pts',(-1.81161420806656,-1.,-1.21870906103557));
#29080=CARTESIAN_POINT('Ctrl Pts',(-1.81161420806656,1.,-1.21870906103557));
#29081=CARTESIAN_POINT('Ctrl Pts',(-1.80882996917129,-1.,-1.21290815708314));
#29082=CARTESIAN_POINT('Ctrl Pts',(-1.80882996917129,1.,-1.21290815708314));
#29083=CARTESIAN_POINT('Ctrl Pts',(-1.80601678480707,-1.,-1.20713356605475));
#29084=CARTESIAN_POINT('Ctrl Pts',(-1.80601678480707,1.,-1.20713356605475));
#29085=CARTESIAN_POINT('Ctrl Pts',(-1.80317454838603,-1.,-1.20138548938974));
#29086=CARTESIAN_POINT('Ctrl Pts',(-1.80317454838603,1.,-1.20138548938974));
#29087=CARTESIAN_POINT('Ctrl Pts',(-1.80030314369879,-1.,-1.19566418930242));
#29088=CARTESIAN_POINT('Ctrl Pts',(-1.80030314369879,1.,-1.19566418930242));
#29089=CARTESIAN_POINT('Ctrl Pts',(-1.79740245923478,-1.,-1.18996997934445));
#29090=CARTESIAN_POINT('Ctrl Pts',(-1.79740245923478,1.,-1.18996997934445));
#29091=CARTESIAN_POINT('Ctrl Pts',(-1.79447240321515,-1.,-1.18430321697432));
#29092=CARTESIAN_POINT('Ctrl Pts',(-1.79447240321515,1.,-1.18430321697432));
#29093=CARTESIAN_POINT('Ctrl Pts',(-1.79151291552689,-1.,-1.17866429440809));
#29094=CARTESIAN_POINT('Ctrl Pts',(-1.79151291552689,1.,-1.17866429440809));
#29095=CARTESIAN_POINT('Ctrl Pts',(-1.78852398877616,-1.,-1.17305363177328));
#29096=CARTESIAN_POINT('Ctrl Pts',(-1.78852398877616,1.,-1.17305363177328));
#29097=CARTESIAN_POINT('Ctrl Pts',(-1.78550566040443,-1.,-1.16747166312303));
#29098=CARTESIAN_POINT('Ctrl Pts',(-1.78550566040443,1.,-1.16747166312303));
#29099=CARTESIAN_POINT('Ctrl Pts',(-1.78245795881009,-1.,-1.16191881298499));
#29100=CARTESIAN_POINT('Ctrl Pts',(-1.78245795881009,1.,-1.16191881298499));
#29101=CARTESIAN_POINT('Ctrl Pts',(-1.77938085564275,-1.,-1.15639547194698));
#29102=CARTESIAN_POINT('Ctrl Pts',(-1.77938085564275,1.,-1.15639547194698));
#29103=CARTESIAN_POINT('Ctrl Pts',(-1.7762742255701,-1.,-1.15090197841515));
#29104=CARTESIAN_POINT('Ctrl Pts',(-1.7762742255701,1.,-1.15090197841515));
#29105=CARTESIAN_POINT('Ctrl Pts',(-1.77313777896194,-1.,-1.1454385822692));
#29106=CARTESIAN_POINT('Ctrl Pts',(-1.77313777896194,1.,-1.1454385822692));
#29107=CARTESIAN_POINT('Ctrl Pts',(-1.76997111386769,-1.,-1.14000548336975));
#29108=CARTESIAN_POINT('Ctrl Pts',(-1.76997111386769,1.,-1.14000548336975));
#29109=CARTESIAN_POINT('Ctrl Pts',(-1.76677384551862,-1.,-1.1346029180462));
#29110=CARTESIAN_POINT('Ctrl Pts',(-1.76677384551862,1.,-1.1346029180462));
#29111=CARTESIAN_POINT('Ctrl Pts',(-1.7635457196617,-1.,-1.12923123555075));
#29112=CARTESIAN_POINT('Ctrl Pts',(-1.7635457196617,1.,-1.12923123555075));
#29113=CARTESIAN_POINT('Ctrl Pts',(-1.76028671825096,-1.,-1.12389096855086));
#29114=CARTESIAN_POINT('Ctrl Pts',(-1.76028671825096,1.,-1.12389096855086));
#29115=CARTESIAN_POINT('Ctrl Pts',(-1.75699720772105,-1.,-1.11858293216763));
#29116=CARTESIAN_POINT('Ctrl Pts',(-1.75699720772105,1.,-1.11858293216763));
#29117=CARTESIAN_POINT('Ctrl Pts',(-1.7536777209463,-1.,-1.11330807582551));
#29118=CARTESIAN_POINT('Ctrl Pts',(-1.7536777209463,1.,-1.11330807582551));
#29119=CARTESIAN_POINT('Ctrl Pts',(-1.7503286607592,-1.,-1.10806728183007));
#29120=CARTESIAN_POINT('Ctrl Pts',(-1.7503286607592,1.,-1.10806728183007));
#29121=CARTESIAN_POINT('Ctrl Pts',(-1.74695004214923,-1.,-1.10286118991143));
#29122=CARTESIAN_POINT('Ctrl Pts',(-1.74695004214923,1.,-1.10286118991143));
#29123=CARTESIAN_POINT('Ctrl Pts',(-1.74354119236208,-1.,-1.09768999241225));
#29124=CARTESIAN_POINT('Ctrl Pts',(-1.74354119236208,1.,-1.09768999241225));
#29125=CARTESIAN_POINT('Ctrl Pts',(-1.74010053962247,-1.,-1.09255329056493));
#29126=CARTESIAN_POINT('Ctrl Pts',(-1.74010053962247,1.,-1.09255329056493));
#29127=CARTESIAN_POINT('Ctrl Pts',(-1.73662628326091,-1.,-1.08745056285427));
#29128=CARTESIAN_POINT('Ctrl Pts',(-1.73662628326091,1.,-1.08745056285427));
#29129=CARTESIAN_POINT('Ctrl Pts',(-1.73311705663407,-1.,-1.08238162784749));
#29130=CARTESIAN_POINT('Ctrl Pts',(-1.73311705663407,1.,-1.08238162784749));
#29131=CARTESIAN_POINT('Ctrl Pts',(-1.72957248977424,-1.,-1.0773470373727));
#29132=CARTESIAN_POINT('Ctrl Pts',(-1.72957248977424,1.,-1.0773470373727));
#29133=CARTESIAN_POINT('Ctrl Pts',(-1.72599406198488,-1.,-1.07234866990252));
#29134=CARTESIAN_POINT('Ctrl Pts',(-1.72599406198488,1.,-1.07234866990252));
#29135=CARTESIAN_POINT('Ctrl Pts',(-1.72238500928453,-1.,-1.06738966975462));
#29136=CARTESIAN_POINT('Ctrl Pts',(-1.72238500928453,1.,-1.06738966975462));
#29137=CARTESIAN_POINT('Ctrl Pts',(-1.71874858456904,-1.,-1.06247324680647));
#29138=CARTESIAN_POINT('Ctrl Pts',(-1.71874858456904,1.,-1.06247324680647));
#29139=CARTESIAN_POINT('Ctrl Pts',(-1.7150865442702,-1.,-1.05760163192479));
#29140=CARTESIAN_POINT('Ctrl Pts',(-1.7150865442702,1.,-1.05760163192479));
#29141=CARTESIAN_POINT('Ctrl Pts',(-1.71139783543989,-1.,-1.05277517202855));
#29142=CARTESIAN_POINT('Ctrl Pts',(-1.71139783543989,1.,-1.05277517202855));
#29143=CARTESIAN_POINT('Ctrl Pts',(-1.70767646263649,-1.,-1.04799085404995));
#29144=CARTESIAN_POINT('Ctrl Pts',(-1.70767646263649,1.,-1.04799085404995));
#29145=CARTESIAN_POINT('Ctrl Pts',(-1.70391338707982,-1.,-1.04324363334554));
#29146=CARTESIAN_POINT('Ctrl Pts',(-1.70391338707982,1.,-1.04324363334554));
#29147=CARTESIAN_POINT('Ctrl Pts',(-1.70010052930962,-1.,-1.03852922490789));
#29148=CARTESIAN_POINT('Ctrl Pts',(-1.70010052930962,1.,-1.03852922490789));
#29149=CARTESIAN_POINT('Ctrl Pts',(-1.69623414782771,-1.,-1.03384646003588));
#29150=CARTESIAN_POINT('Ctrl Pts',(-1.69623414782771,1.,-1.03384646003588));
#29151=CARTESIAN_POINT('Ctrl Pts',(-1.69231840863458,-1.,-1.02919977579147));
#29152=CARTESIAN_POINT('Ctrl Pts',(-1.69231840863458,1.,-1.02919977579147));
#29153=CARTESIAN_POINT('Ctrl Pts',(-1.68836910178447,-1.,-1.02460180535255));
#29154=CARTESIAN_POINT('Ctrl Pts',(-1.68836910178447,1.,-1.02460180535255));
#29155=CARTESIAN_POINT('Ctrl Pts',(-1.68440578021706,-1.,-1.02006795074201));
#29156=CARTESIAN_POINT('Ctrl Pts',(-1.68440578021706,1.,-1.02006795074201));
#29157=CARTESIAN_POINT('Ctrl Pts',(-1.68044289894798,-1.,-1.01561026162773));
#29158=CARTESIAN_POINT('Ctrl Pts',(-1.68044289894798,1.,-1.01561026162773));
#29159=CARTESIAN_POINT('Ctrl Pts',(-1.67648246776464,-1.,-1.01123236493511));
#29160=CARTESIAN_POINT('Ctrl Pts',(-1.67648246776464,1.,-1.01123236493511));
#29161=CARTESIAN_POINT('Ctrl Pts',(-1.67250335383293,-1.,-1.00692206696414));
#29162=CARTESIAN_POINT('Ctrl Pts',(-1.67250335383293,1.,-1.00692206696414));
#29163=CARTESIAN_POINT('Ctrl Pts',(-1.66846059277303,-1.,-1.00265091003727));
#29164=CARTESIAN_POINT('Ctrl Pts',(-1.66846059277303,1.,-1.00265091003727));
#29165=CARTESIAN_POINT('Ctrl Pts',(-1.66430758030376,-1.,-0.998389654952758));
#29166=CARTESIAN_POINT('Ctrl Pts',(-1.66430758030376,1.,-0.998389654952758));
#29167=CARTESIAN_POINT('Ctrl Pts',(-1.66001553809947,-1.,-0.994121836661306));
#29168=CARTESIAN_POINT('Ctrl Pts',(-1.66001553809947,1.,-0.994121836661306));
#29169=CARTESIAN_POINT('Ctrl Pts',(-1.65559044289699,-1.,-0.989855627854165));
#29170=CARTESIAN_POINT('Ctrl Pts',(-1.65559044289699,1.,-0.989855627854165));
#29171=CARTESIAN_POINT('Ctrl Pts',(-1.65110016612638,-1.,-0.985642622920821));
#29172=CARTESIAN_POINT('Ctrl Pts',(-1.65110016612638,1.,-0.985642622920821));
#29173=CARTESIAN_POINT('Ctrl Pts',(-1.64665139190656,-1.,-0.981562530939489));
#29174=CARTESIAN_POINT('Ctrl Pts',(-1.64665139190656,1.,-0.981562530939489));
#29175=CARTESIAN_POINT('Ctrl Pts',(-1.64233990826687,-1.,-0.977689794119416));
#29176=CARTESIAN_POINT('Ctrl Pts',(-1.64233990826687,1.,-0.977689794119416));
#29177=CARTESIAN_POINT('Ctrl Pts',(-1.63820952658144,-1.,-0.974066058287418));
#29178=CARTESIAN_POINT('Ctrl Pts',(-1.63820952658144,1.,-0.974066058287418));
#29179=CARTESIAN_POINT('Ctrl Pts',(-1.63420665729798,-1.,-0.970669715997509));
#29180=CARTESIAN_POINT('Ctrl Pts',(-1.63420665729798,1.,-0.970669715997509));
#29181=CARTESIAN_POINT('Ctrl Pts',(-1.63013849959461,-1.,-0.967387853230345));
#29182=CARTESIAN_POINT('Ctrl Pts',(-1.63013849959461,1.,-0.967387853230345));
#29183=CARTESIAN_POINT('Ctrl Pts',(-1.62571930670187,-1.,-0.964046107040536));
#29184=CARTESIAN_POINT('Ctrl Pts',(-1.62571930670187,1.,-0.964046107040536));
#29185=CARTESIAN_POINT('Ctrl Pts',(-1.62061638140221,-1.,-0.960438326101729));
#29186=CARTESIAN_POINT('Ctrl Pts',(-1.62061638140221,1.,-0.960438326101729));
#29187=CARTESIAN_POINT('Ctrl Pts',(-1.61449324337085,-1.,-0.956354422920671));
#29188=CARTESIAN_POINT('Ctrl Pts',(-1.61449324337085,1.,-0.956354422920671));
#29189=CARTESIAN_POINT('Ctrl Pts',(-1.60706069896936,-1.,-0.951613284356035));
#29190=CARTESIAN_POINT('Ctrl Pts',(-1.60706069896936,1.,-0.951613284356035));
#29191=CARTESIAN_POINT('Ctrl Pts',(-1.59810042043673,-1.,-0.946078063315257));
#29192=CARTESIAN_POINT('Ctrl Pts',(-1.59810042043673,1.,-0.946078063315257));
#29193=CARTESIAN_POINT('Ctrl Pts',(-1.58744937487176,-1.,-0.939646377893399));
#29194=CARTESIAN_POINT('Ctrl Pts',(-1.58744937487176,1.,-0.939646377893399));
#29195=CARTESIAN_POINT('Ctrl Pts',(-1.57499388382243,-1.,-0.932246680108685));
#29196=CARTESIAN_POINT('Ctrl Pts',(-1.57499388382243,1.,-0.932246680108685));
#29197=CARTESIAN_POINT('Ctrl Pts',(-1.56065988578893,-1.,-0.923832188944341));
#29198=CARTESIAN_POINT('Ctrl Pts',(-1.56065988578893,1.,-0.923832188944341));
#29199=CARTESIAN_POINT('Ctrl Pts',(-1.54440491149498,-1.,-0.914375919026456));
#29200=CARTESIAN_POINT('Ctrl Pts',(-1.54440491149498,1.,-0.914375919026456));
#29201=CARTESIAN_POINT('Ctrl Pts',(-1.52984849887993,-1.,-0.905967409625651));
#29202=CARTESIAN_POINT('Ctrl Pts',(-1.52984849887993,1.,-0.905967409625651));
#29203=CARTESIAN_POINT('Ctrl Pts',(-1.51805569590094,-1.,-0.899185047483511));
#29204=CARTESIAN_POINT('Ctrl Pts',(-1.51805569590094,1.,-0.899185047483511));
#29205=CARTESIAN_POINT('Ctrl Pts',(-1.50980486806688,-1.,-0.894452006964543));
#29206=CARTESIAN_POINT('Ctrl Pts',(-1.50980486806688,1.,-0.894452006964543));
#29207=CARTESIAN_POINT('Ctrl Pts',(-1.5055822144029,-1.,-0.892032620296855));
#29208=CARTESIAN_POINT('Ctrl Pts',(-1.5055822144029,1.,-0.892032620296855));
#29209=CARTESIAN_POINT('',(-1.81978687191668,1.,-1.23627494547115));
#29210=CARTESIAN_POINT('Ctrl Pts',(-1.81978687191668,1.,-1.23627494547115));
#29211=CARTESIAN_POINT('Ctrl Pts',(-1.81925017193666,1.,-1.23509651170476));
#29212=CARTESIAN_POINT('Ctrl Pts',(-1.81817389921279,1.,-1.2327422452705));
#29213=CARTESIAN_POINT('Ctrl Pts',(-1.8165508718364,1.,-1.2292186489137));
#29214=CARTESIAN_POINT('Ctrl Pts',(-1.81436959210434,1.,-1.2245361330495));
#29215=CARTESIAN_POINT('Ctrl Pts',(-1.81161420806656,1.,-1.21870906103557));
#29216=CARTESIAN_POINT('Ctrl Pts',(-1.80882996917129,1.,-1.21290815708314));
#29217=CARTESIAN_POINT('Ctrl Pts',(-1.80601678480707,1.,-1.20713356605475));
#29218=CARTESIAN_POINT('Ctrl Pts',(-1.80317454838603,1.,-1.20138548938974));
#29219=CARTESIAN_POINT('Ctrl Pts',(-1.80030314369879,1.,-1.19566418930242));
#29220=CARTESIAN_POINT('Ctrl Pts',(-1.79740245923478,1.,-1.18996997934445));
#29221=CARTESIAN_POINT('Ctrl Pts',(-1.79447240321515,1.,-1.18430321697432));
#29222=CARTESIAN_POINT('Ctrl Pts',(-1.79151291552689,1.,-1.17866429440809));
#29223=CARTESIAN_POINT('Ctrl Pts',(-1.78852398877616,1.,-1.17305363177328));
#29224=CARTESIAN_POINT('Ctrl Pts',(-1.78550566040443,1.,-1.16747166312303));
#29225=CARTESIAN_POINT('Ctrl Pts',(-1.78245795881009,1.,-1.16191881298499));
#29226=CARTESIAN_POINT('Ctrl Pts',(-1.77938085564275,1.,-1.15639547194698));
#29227=CARTESIAN_POINT('Ctrl Pts',(-1.7762742255701,1.,-1.15090197841515));
#29228=CARTESIAN_POINT('Ctrl Pts',(-1.77313777896194,1.,-1.1454385822692));
#29229=CARTESIAN_POINT('Ctrl Pts',(-1.76997111386769,1.,-1.14000548336975));
#29230=CARTESIAN_POINT('Ctrl Pts',(-1.76677384551862,1.,-1.1346029180462));
#29231=CARTESIAN_POINT('Ctrl Pts',(-1.7635457196617,1.,-1.12923123555075));
#29232=CARTESIAN_POINT('Ctrl Pts',(-1.76028671825096,1.,-1.12389096855086));
#29233=CARTESIAN_POINT('Ctrl Pts',(-1.75699720772105,1.,-1.11858293216763));
#29234=CARTESIAN_POINT('Ctrl Pts',(-1.7536777209463,1.,-1.11330807582551));
#29235=CARTESIAN_POINT('Ctrl Pts',(-1.7503286607592,1.,-1.10806728183007));
#29236=CARTESIAN_POINT('Ctrl Pts',(-1.74695004214923,1.,-1.10286118991143));
#29237=CARTESIAN_POINT('Ctrl Pts',(-1.74354119236208,1.,-1.09768999241225));
#29238=CARTESIAN_POINT('Ctrl Pts',(-1.74010053962247,1.,-1.09255329056493));
#29239=CARTESIAN_POINT('Ctrl Pts',(-1.73662628326091,1.,-1.08745056285427));
#29240=CARTESIAN_POINT('Ctrl Pts',(-1.73311705663407,1.,-1.08238162784749));
#29241=CARTESIAN_POINT('Ctrl Pts',(-1.72957248977424,1.,-1.0773470373727));
#29242=CARTESIAN_POINT('Ctrl Pts',(-1.72599406198488,1.,-1.07234866990252));
#29243=CARTESIAN_POINT('Ctrl Pts',(-1.72238500928453,1.,-1.06738966975462));
#29244=CARTESIAN_POINT('Ctrl Pts',(-1.71874858456904,1.,-1.06247324680647));
#29245=CARTESIAN_POINT('Ctrl Pts',(-1.7150865442702,1.,-1.05760163192479));
#29246=CARTESIAN_POINT('Ctrl Pts',(-1.71139783543989,1.,-1.05277517202855));
#29247=CARTESIAN_POINT('Ctrl Pts',(-1.70767646263649,1.,-1.04799085404995));
#29248=CARTESIAN_POINT('Ctrl Pts',(-1.70391338707982,1.,-1.04324363334554));
#29249=CARTESIAN_POINT('Ctrl Pts',(-1.70010052930962,1.,-1.03852922490789));
#29250=CARTESIAN_POINT('Ctrl Pts',(-1.69623414782771,1.,-1.03384646003588));
#29251=CARTESIAN_POINT('Ctrl Pts',(-1.69231840863458,1.,-1.02919977579147));
#29252=CARTESIAN_POINT('Ctrl Pts',(-1.68836910178447,1.,-1.02460180535255));
#29253=CARTESIAN_POINT('Ctrl Pts',(-1.68440578021706,1.,-1.02006795074201));
#29254=CARTESIAN_POINT('Ctrl Pts',(-1.68044289894798,1.,-1.01561026162773));
#29255=CARTESIAN_POINT('Ctrl Pts',(-1.67648246776464,1.,-1.01123236493511));
#29256=CARTESIAN_POINT('Ctrl Pts',(-1.67250335383293,1.,-1.00692206696414));
#29257=CARTESIAN_POINT('Ctrl Pts',(-1.66846059277303,1.,-1.00265091003727));
#29258=CARTESIAN_POINT('Ctrl Pts',(-1.66430758030376,1.,-0.998389654952758));
#29259=CARTESIAN_POINT('Ctrl Pts',(-1.66001553809947,1.,-0.994121836661306));
#29260=CARTESIAN_POINT('Ctrl Pts',(-1.65559044289699,1.,-0.989855627854165));
#29261=CARTESIAN_POINT('Ctrl Pts',(-1.65110016612638,1.,-0.985642622920821));
#29262=CARTESIAN_POINT('Ctrl Pts',(-1.64665139190656,1.,-0.981562530939489));
#29263=CARTESIAN_POINT('Ctrl Pts',(-1.64233990826687,1.,-0.977689794119416));
#29264=CARTESIAN_POINT('Ctrl Pts',(-1.63820952658144,1.,-0.974066058287418));
#29265=CARTESIAN_POINT('Ctrl Pts',(-1.63420665729798,1.,-0.970669715997509));
#29266=CARTESIAN_POINT('Ctrl Pts',(-1.63013849959461,1.,-0.967387853230345));
#29267=CARTESIAN_POINT('Ctrl Pts',(-1.62571930670187,1.,-0.964046107040536));
#29268=CARTESIAN_POINT('Ctrl Pts',(-1.62061638140221,1.,-0.960438326101729));
#29269=CARTESIAN_POINT('Ctrl Pts',(-1.61449324337085,1.,-0.956354422920671));
#29270=CARTESIAN_POINT('Ctrl Pts',(-1.60706069896936,1.,-0.951613284356035));
#29271=CARTESIAN_POINT('Ctrl Pts',(-1.59810042043673,1.,-0.946078063315257));
#29272=CARTESIAN_POINT('Ctrl Pts',(-1.58744937487176,1.,-0.939646377893399));
#29273=CARTESIAN_POINT('Ctrl Pts',(-1.57499388382243,1.,-0.932246680108685));
#29274=CARTESIAN_POINT('Ctrl Pts',(-1.56065988578893,1.,-0.923832188944341));
#29275=CARTESIAN_POINT('Ctrl Pts',(-1.54440491149498,1.,-0.914375919026456));
#29276=CARTESIAN_POINT('Ctrl Pts',(-1.52984849887993,1.,-0.905967409625651));
#29277=CARTESIAN_POINT('Ctrl Pts',(-1.51805569590094,1.,-0.899185047483511));
#29278=CARTESIAN_POINT('Ctrl Pts',(-1.50980486806688,1.,-0.894452006964543));
#29279=CARTESIAN_POINT('Ctrl Pts',(-1.5055822144029,1.,-0.892032620296855));
#29280=CARTESIAN_POINT('',(-1.81978687191668,0.,-1.23627494547115));
#29281=CARTESIAN_POINT('Origin',(-1.73811241238545,0.,-1.34869019493419));
#29282=CARTESIAN_POINT('',(-1.73811241238545,1.,-1.34869019493419));
#29283=CARTESIAN_POINT('',(-1.81978687191668,1.,-1.23627494547115));
#29284=CARTESIAN_POINT('',(-1.73811241238545,0.,-1.34869019493419));
#29285=CARTESIAN_POINT('Ctrl Pts',(-1.31362392696032,-1.,-1.15624053661742));
#29286=CARTESIAN_POINT('Ctrl Pts',(-1.31362392696032,1.,-1.15624053661742));
#29287=CARTESIAN_POINT('Ctrl Pts',(-1.31722977216397,-1.,-1.15950888730809));
#29288=CARTESIAN_POINT('Ctrl Pts',(-1.31722977216397,1.,-1.15950888730809));
#29289=CARTESIAN_POINT('Ctrl Pts',(-1.32428080721772,-1.,-1.16589330093588));
#29290=CARTESIAN_POINT('Ctrl Pts',(-1.32428080721772,1.,-1.16589330093588));
#29291=CARTESIAN_POINT('Ctrl Pts',(-1.33437539347008,-1.,-1.17501305789857));
#29292=CARTESIAN_POINT('Ctrl Pts',(-1.33437539347008,1.,-1.17501305789857));
#29293=CARTESIAN_POINT('Ctrl Pts',(-1.34687054001093,-1.,-1.18625865667441));
#29294=CARTESIAN_POINT('Ctrl Pts',(-1.34687054001093,1.,-1.18625865667441));
#29295=CARTESIAN_POINT('Ctrl Pts',(-1.36088705043885,-1.,-1.1987959077932));
#29296=CARTESIAN_POINT('Ctrl Pts',(-1.36088705043885,1.,-1.1987959077932));
#29297=CARTESIAN_POINT('Ctrl Pts',(-1.37331915607905,-1.,-1.20982812925645));
#29298=CARTESIAN_POINT('Ctrl Pts',(-1.37331915607905,1.,-1.20982812925645));
#29299=CARTESIAN_POINT('Ctrl Pts',(-1.38420564527715,-1.,-1.21938737280852));
#29300=CARTESIAN_POINT('Ctrl Pts',(-1.38420564527715,1.,-1.21938737280852));
#29301=CARTESIAN_POINT('Ctrl Pts',(-1.39361389568796,-1.,-1.22752961899387));
#29302=CARTESIAN_POINT('Ctrl Pts',(-1.39361389568796,1.,-1.22752961899387));
#29303=CARTESIAN_POINT('Ctrl Pts',(-1.40164708206106,-1.,-1.23434087290423));
#29304=CARTESIAN_POINT('Ctrl Pts',(-1.40164708206106,1.,-1.23434087290423));
#29305=CARTESIAN_POINT('Ctrl Pts',(-1.40845295531283,-1.,-1.23994455029534));
#29306=CARTESIAN_POINT('Ctrl Pts',(-1.40845295531283,1.,-1.23994455029534));
#29307=CARTESIAN_POINT('Ctrl Pts',(-1.41422913175179,-1.,-1.24450600513056));
#29308=CARTESIAN_POINT('Ctrl Pts',(-1.41422913175179,1.,-1.24450600513056));
#29309=CARTESIAN_POINT('Ctrl Pts',(-1.41923722596025,-1.,-1.24824430986571));
#29310=CARTESIAN_POINT('Ctrl Pts',(-1.41923722596025,1.,-1.24824430986571));
#29311=CARTESIAN_POINT('Ctrl Pts',(-1.42378102115575,-1.,-1.2514145557001));
#29312=CARTESIAN_POINT('Ctrl Pts',(-1.42378102115575,1.,-1.2514145557001));
#29313=CARTESIAN_POINT('Ctrl Pts',(-1.42815938799387,-1.,-1.25426945222639));
#29314=CARTESIAN_POINT('Ctrl Pts',(-1.42815938799387,1.,-1.25426945222639));
#29315=CARTESIAN_POINT('Ctrl Pts',(-1.43262645609691,-1.,-1.25702687965755));
#29316=CARTESIAN_POINT('Ctrl Pts',(-1.43262645609691,1.,-1.25702687965755));
#29317=CARTESIAN_POINT('Ctrl Pts',(-1.43734919180848,-1.,-1.25983531012005));
#29318=CARTESIAN_POINT('Ctrl Pts',(-1.43734919180848,1.,-1.25983531012005));
#29319=CARTESIAN_POINT('Ctrl Pts',(-1.44236470511303,-1.,-1.26273903323859));
#29320=CARTESIAN_POINT('Ctrl Pts',(-1.44236470511303,1.,-1.26273903323859));
#29321=CARTESIAN_POINT('Ctrl Pts',(-1.44761985001662,-1.,-1.26570925118868));
#29322=CARTESIAN_POINT('Ctrl Pts',(-1.44761985001662,1.,-1.26570925118868));
#29323=CARTESIAN_POINT('Ctrl Pts',(-1.45301422764247,-1.,-1.2686778680489));
#29324=CARTESIAN_POINT('Ctrl Pts',(-1.45301422764247,1.,-1.2686778680489));
#29325=CARTESIAN_POINT('Ctrl Pts',(-1.45843906294697,-1.,-1.27156805265289));
#29326=CARTESIAN_POINT('Ctrl Pts',(-1.45843906294697,1.,-1.27156805265289));
#29327=CARTESIAN_POINT('Ctrl Pts',(-1.46382431332476,-1.,-1.27433119897822));
#29328=CARTESIAN_POINT('Ctrl Pts',(-1.46382431332476,1.,-1.27433119897822));
#29329=CARTESIAN_POINT('Ctrl Pts',(-1.46916035917133,-1.,-1.27696414831089));
#29330=CARTESIAN_POINT('Ctrl Pts',(-1.46916035917133,1.,-1.27696414831089));
#29331=CARTESIAN_POINT('Ctrl Pts',(-1.4744717526707,-1.,-1.2794891824849));
#29332=CARTESIAN_POINT('Ctrl Pts',(-1.4744717526707,1.,-1.2794891824849));
#29333=CARTESIAN_POINT('Ctrl Pts',(-1.47980070347095,-1.,-1.28194158939517));
#29334=CARTESIAN_POINT('Ctrl Pts',(-1.47980070347095,1.,-1.28194158939517));
#29335=CARTESIAN_POINT('Ctrl Pts',(-1.4851881711891,-1.,-1.28435533880201));
#29336=CARTESIAN_POINT('Ctrl Pts',(-1.4851881711891,1.,-1.28435533880201));
#29337=CARTESIAN_POINT('Ctrl Pts',(-1.4906522831278,-1.,-1.2867467611644));
#29338=CARTESIAN_POINT('Ctrl Pts',(-1.4906522831278,1.,-1.2867467611644));
#29339=CARTESIAN_POINT('Ctrl Pts',(-1.49618896881754,-1.,-1.28911506584254));
#29340=CARTESIAN_POINT('Ctrl Pts',(-1.49618896881754,1.,-1.28911506584254));
#29341=CARTESIAN_POINT('Ctrl Pts',(-1.50178230149776,-1.,-1.29145022885181));
#29342=CARTESIAN_POINT('Ctrl Pts',(-1.50178230149776,1.,-1.29145022885181));
#29343=CARTESIAN_POINT('Ctrl Pts',(-1.50741159078365,-1.,-1.29373841372842));
#29344=CARTESIAN_POINT('Ctrl Pts',(-1.50741159078365,1.,-1.29373841372842));
#29345=CARTESIAN_POINT('Ctrl Pts',(-1.51305994241402,-1.,-1.29596850710509));
#29346=CARTESIAN_POINT('Ctrl Pts',(-1.51305994241402,1.,-1.29596850710509));
#29347=CARTESIAN_POINT('Ctrl Pts',(-1.51872184912724,-1.,-1.29813791800747));
#29348=CARTESIAN_POINT('Ctrl Pts',(-1.51872184912724,1.,-1.29813791800747));
#29349=CARTESIAN_POINT('Ctrl Pts',(-1.52439957861062,-1.,-1.30024984366328));
#29350=CARTESIAN_POINT('Ctrl Pts',(-1.52439957861062,1.,-1.30024984366328));
#29351=CARTESIAN_POINT('Ctrl Pts',(-1.53009970283891,-1.,-1.30231064395568));
#29352=CARTESIAN_POINT('Ctrl Pts',(-1.53009970283891,1.,-1.30231064395568));
#29353=CARTESIAN_POINT('Ctrl Pts',(-1.53582981268977,-1.,-1.30432735639489));
#29354=CARTESIAN_POINT('Ctrl Pts',(-1.53582981268977,1.,-1.30432735639489));
#29355=CARTESIAN_POINT('Ctrl Pts',(-1.54159462645432,-1.,-1.30630475189556));
#29356=CARTESIAN_POINT('Ctrl Pts',(-1.54159462645432,1.,-1.30630475189556));
#29357=CARTESIAN_POINT('Ctrl Pts',(-1.54739413957185,-1.,-1.30824393907473));
#29358=CARTESIAN_POINT('Ctrl Pts',(-1.54739413957185,1.,-1.30824393907473));
#29359=CARTESIAN_POINT('Ctrl Pts',(-1.55322568759481,-1.,-1.31014393684222));
#29360=CARTESIAN_POINT('Ctrl Pts',(-1.55322568759481,1.,-1.31014393684222));
#29361=CARTESIAN_POINT('Ctrl Pts',(-1.55908521254821,-1.,-1.31200264341696));
#29362=CARTESIAN_POINT('Ctrl Pts',(-1.55908521254821,1.,-1.31200264341696));
#29363=CARTESIAN_POINT('Ctrl Pts',(-1.56496872402353,-1.,-1.31381795281002));
#29364=CARTESIAN_POINT('Ctrl Pts',(-1.56496872402353,1.,-1.31381795281002));
#29365=CARTESIAN_POINT('Ctrl Pts',(-1.57087397835723,-1.,-1.31558903860016));
#29366=CARTESIAN_POINT('Ctrl Pts',(-1.57087397835723,1.,-1.31558903860016));
#29367=CARTESIAN_POINT('Ctrl Pts',(-1.5768005650559,-1.,-1.31731642317187));
#29368=CARTESIAN_POINT('Ctrl Pts',(-1.5768005650559,1.,-1.31731642317187));
#29369=CARTESIAN_POINT('Ctrl Pts',(-1.58274907898834,-1.,-1.31900135021432));
#29370=CARTESIAN_POINT('Ctrl Pts',(-1.58274907898834,1.,-1.31900135021432));
#29371=CARTESIAN_POINT('Ctrl Pts',(-1.58872057258245,-1.,-1.32064537110892));
#29372=CARTESIAN_POINT('Ctrl Pts',(-1.58872057258245,1.,-1.32064537110892));
#29373=CARTESIAN_POINT('Ctrl Pts',(-1.59471591079403,-1.,-1.32224985747682));
#29374=CARTESIAN_POINT('Ctrl Pts',(-1.59471591079403,1.,-1.32224985747682));
#29375=CARTESIAN_POINT('Ctrl Pts',(-1.60073511858687,-1.,-1.32381550858256));
#29376=CARTESIAN_POINT('Ctrl Pts',(-1.60073511858687,1.,-1.32381550858256));
#29377=CARTESIAN_POINT('Ctrl Pts',(-1.60677758290954,-1.,-1.32534250785782));
#29378=CARTESIAN_POINT('Ctrl Pts',(-1.60677758290954,1.,-1.32534250785782));
#29379=CARTESIAN_POINT('Ctrl Pts',(-1.6128423401575,-1.,-1.32683074483356));
#29380=CARTESIAN_POINT('Ctrl Pts',(-1.6128423401575,1.,-1.32683074483356));
#29381=CARTESIAN_POINT('Ctrl Pts',(-1.61892832270724,-1.,-1.32828000610449));
#29382=CARTESIAN_POINT('Ctrl Pts',(-1.61892832270724,1.,-1.32828000610449));
#29383=CARTESIAN_POINT('Ctrl Pts',(-1.62503464209797,-1.,-1.3296901950568));
#29384=CARTESIAN_POINT('Ctrl Pts',(-1.62503464209797,1.,-1.3296901950568));
#29385=CARTESIAN_POINT('Ctrl Pts',(-1.63116079730923,-1.,-1.33106149345645));
#29386=CARTESIAN_POINT('Ctrl Pts',(-1.63116079730923,1.,-1.33106149345645));
#29387=CARTESIAN_POINT('Ctrl Pts',(-1.63730653475089,-1.,-1.33239425103724));
#29388=CARTESIAN_POINT('Ctrl Pts',(-1.63730653475089,1.,-1.33239425103724));
#29389=CARTESIAN_POINT('Ctrl Pts',(-1.6434717485603,-1.,-1.33368890676572));
#29390=CARTESIAN_POINT('Ctrl Pts',(-1.6434717485603,1.,-1.33368890676572));
#29391=CARTESIAN_POINT('Ctrl Pts',(-1.6496563728683,-1.,-1.33494590467993));
#29392=CARTESIAN_POINT('Ctrl Pts',(-1.6496563728683,1.,-1.33494590467993));
#29393=CARTESIAN_POINT('Ctrl Pts',(-1.65586025952593,-1.,-1.33616559745172));
#29394=CARTESIAN_POINT('Ctrl Pts',(-1.65586025952593,1.,-1.33616559745172));
#29395=CARTESIAN_POINT('Ctrl Pts',(-1.66208312541983,-1.,-1.33734820885262));
#29396=CARTESIAN_POINT('Ctrl Pts',(-1.66208312541983,1.,-1.33734820885262));
#29397=CARTESIAN_POINT('Ctrl Pts',(-1.66832460783989,-1.,-1.33849388654388));
#29398=CARTESIAN_POINT('Ctrl Pts',(-1.66832460783989,1.,-1.33849388654388));
#29399=CARTESIAN_POINT('Ctrl Pts',(-1.67458429426086,-1.,-1.3396027347034));
#29400=CARTESIAN_POINT('Ctrl Pts',(-1.67458429426086,1.,-1.3396027347034));
#29401=CARTESIAN_POINT('Ctrl Pts',(-1.68086176030362,-1.,-1.34067485185203));
#29402=CARTESIAN_POINT('Ctrl Pts',(-1.68086176030362,1.,-1.34067485185203));
#29403=CARTESIAN_POINT('Ctrl Pts',(-1.68715660868764,-1.,-1.341710374848));
#29404=CARTESIAN_POINT('Ctrl Pts',(-1.68715660868764,1.,-1.341710374848));
#29405=CARTESIAN_POINT('Ctrl Pts',(-1.6934684849687,-1.,-1.34270948206319));
#29406=CARTESIAN_POINT('Ctrl Pts',(-1.6934684849687,1.,-1.34270948206319));
#29407=CARTESIAN_POINT('Ctrl Pts',(-1.69979707754427,-1.,-1.34367237124483));
#29408=CARTESIAN_POINT('Ctrl Pts',(-1.69979707754427,1.,-1.34367237124483));
#29409=CARTESIAN_POINT('Ctrl Pts',(-1.70614212266738,-1.,-1.34459924533831));
#29410=CARTESIAN_POINT('Ctrl Pts',(-1.70614212266738,1.,-1.34459924533831));
#29411=CARTESIAN_POINT('Ctrl Pts',(-1.71250340686822,-1.,-1.34549029589416));
#29412=CARTESIAN_POINT('Ctrl Pts',(-1.71250340686822,1.,-1.34549029589416));
#29413=CARTESIAN_POINT('Ctrl Pts',(-1.7188807715049,-1.,-1.34634568653227));
#29414=CARTESIAN_POINT('Ctrl Pts',(-1.7188807715049,1.,-1.34634568653227));
#29415=CARTESIAN_POINT('Ctrl Pts',(-1.72527410680674,-1.,-1.34716554819527));
#29416=CARTESIAN_POINT('Ctrl Pts',(-1.72527410680674,1.,-1.34716554819527));
#29417=CARTESIAN_POINT('Ctrl Pts',(-1.7304014965394,-1.,-1.34779309152035));
#29418=CARTESIAN_POINT('Ctrl Pts',(-1.7304014965394,1.,-1.34779309152035));
#29419=CARTESIAN_POINT('Ctrl Pts',(-1.73425417885907,-1.,-1.34824783112887));
#29420=CARTESIAN_POINT('Ctrl Pts',(-1.73425417885907,1.,-1.34824783112887));
#29421=CARTESIAN_POINT('Ctrl Pts',(-1.73682580585691,-1.,-1.34854391898045));
#29422=CARTESIAN_POINT('Ctrl Pts',(-1.73682580585691,1.,-1.34854391898045));
#29423=CARTESIAN_POINT('Ctrl Pts',(-1.73811241238545,-1.,-1.34869019493419));
#29424=CARTESIAN_POINT('Ctrl Pts',(-1.73811241238545,1.,-1.34869019493419));
#29425=CARTESIAN_POINT('',(-1.31362392696032,1.,-1.15624053661742));
#29426=CARTESIAN_POINT('Ctrl Pts',(-1.31362392696032,1.,-1.15624053661742));
#29427=CARTESIAN_POINT('Ctrl Pts',(-1.31722977216397,1.,-1.15950888730809));
#29428=CARTESIAN_POINT('Ctrl Pts',(-1.32428080721772,1.,-1.16589330093588));
#29429=CARTESIAN_POINT('Ctrl Pts',(-1.33437539347008,1.,-1.17501305789857));
#29430=CARTESIAN_POINT('Ctrl Pts',(-1.34687054001093,1.,-1.18625865667441));
#29431=CARTESIAN_POINT('Ctrl Pts',(-1.36088705043885,1.,-1.1987959077932));
#29432=CARTESIAN_POINT('Ctrl Pts',(-1.37331915607905,1.,-1.20982812925645));
#29433=CARTESIAN_POINT('Ctrl Pts',(-1.38420564527715,1.,-1.21938737280852));
#29434=CARTESIAN_POINT('Ctrl Pts',(-1.39361389568796,1.,-1.22752961899387));
#29435=CARTESIAN_POINT('Ctrl Pts',(-1.40164708206106,1.,-1.23434087290423));
#29436=CARTESIAN_POINT('Ctrl Pts',(-1.40845295531283,1.,-1.23994455029534));
#29437=CARTESIAN_POINT('Ctrl Pts',(-1.41422913175179,1.,-1.24450600513056));
#29438=CARTESIAN_POINT('Ctrl Pts',(-1.41923722596025,1.,-1.24824430986571));
#29439=CARTESIAN_POINT('Ctrl Pts',(-1.42378102115575,1.,-1.2514145557001));
#29440=CARTESIAN_POINT('Ctrl Pts',(-1.42815938799387,1.,-1.25426945222639));
#29441=CARTESIAN_POINT('Ctrl Pts',(-1.43262645609691,1.,-1.25702687965755));
#29442=CARTESIAN_POINT('Ctrl Pts',(-1.43734919180848,1.,-1.25983531012005));
#29443=CARTESIAN_POINT('Ctrl Pts',(-1.44236470511303,1.,-1.26273903323859));
#29444=CARTESIAN_POINT('Ctrl Pts',(-1.44761985001662,1.,-1.26570925118868));
#29445=CARTESIAN_POINT('Ctrl Pts',(-1.45301422764247,1.,-1.2686778680489));
#29446=CARTESIAN_POINT('Ctrl Pts',(-1.45843906294697,1.,-1.27156805265289));
#29447=CARTESIAN_POINT('Ctrl Pts',(-1.46382431332476,1.,-1.27433119897822));
#29448=CARTESIAN_POINT('Ctrl Pts',(-1.46916035917133,1.,-1.27696414831089));
#29449=CARTESIAN_POINT('Ctrl Pts',(-1.4744717526707,1.,-1.2794891824849));
#29450=CARTESIAN_POINT('Ctrl Pts',(-1.47980070347095,1.,-1.28194158939517));
#29451=CARTESIAN_POINT('Ctrl Pts',(-1.4851881711891,1.,-1.28435533880201));
#29452=CARTESIAN_POINT('Ctrl Pts',(-1.4906522831278,1.,-1.2867467611644));
#29453=CARTESIAN_POINT('Ctrl Pts',(-1.49618896881754,1.,-1.28911506584254));
#29454=CARTESIAN_POINT('Ctrl Pts',(-1.50178230149776,1.,-1.29145022885181));
#29455=CARTESIAN_POINT('Ctrl Pts',(-1.50741159078365,1.,-1.29373841372842));
#29456=CARTESIAN_POINT('Ctrl Pts',(-1.51305994241402,1.,-1.29596850710509));
#29457=CARTESIAN_POINT('Ctrl Pts',(-1.51872184912724,1.,-1.29813791800747));
#29458=CARTESIAN_POINT('Ctrl Pts',(-1.52439957861062,1.,-1.30024984366328));
#29459=CARTESIAN_POINT('Ctrl Pts',(-1.53009970283891,1.,-1.30231064395568));
#29460=CARTESIAN_POINT('Ctrl Pts',(-1.53582981268977,1.,-1.30432735639489));
#29461=CARTESIAN_POINT('Ctrl Pts',(-1.54159462645432,1.,-1.30630475189556));
#29462=CARTESIAN_POINT('Ctrl Pts',(-1.54739413957185,1.,-1.30824393907473));
#29463=CARTESIAN_POINT('Ctrl Pts',(-1.55322568759481,1.,-1.31014393684222));
#29464=CARTESIAN_POINT('Ctrl Pts',(-1.55908521254821,1.,-1.31200264341696));
#29465=CARTESIAN_POINT('Ctrl Pts',(-1.56496872402353,1.,-1.31381795281002));
#29466=CARTESIAN_POINT('Ctrl Pts',(-1.57087397835723,1.,-1.31558903860016));
#29467=CARTESIAN_POINT('Ctrl Pts',(-1.5768005650559,1.,-1.31731642317187));
#29468=CARTESIAN_POINT('Ctrl Pts',(-1.58274907898834,1.,-1.31900135021432));
#29469=CARTESIAN_POINT('Ctrl Pts',(-1.58872057258245,1.,-1.32064537110892));
#29470=CARTESIAN_POINT('Ctrl Pts',(-1.59471591079403,1.,-1.32224985747682));
#29471=CARTESIAN_POINT('Ctrl Pts',(-1.60073511858687,1.,-1.32381550858256));
#29472=CARTESIAN_POINT('Ctrl Pts',(-1.60677758290954,1.,-1.32534250785782));
#29473=CARTESIAN_POINT('Ctrl Pts',(-1.6128423401575,1.,-1.32683074483356));
#29474=CARTESIAN_POINT('Ctrl Pts',(-1.61892832270724,1.,-1.32828000610449));
#29475=CARTESIAN_POINT('Ctrl Pts',(-1.62503464209797,1.,-1.3296901950568));
#29476=CARTESIAN_POINT('Ctrl Pts',(-1.63116079730923,1.,-1.33106149345645));
#29477=CARTESIAN_POINT('Ctrl Pts',(-1.63730653475089,1.,-1.33239425103724));
#29478=CARTESIAN_POINT('Ctrl Pts',(-1.6434717485603,1.,-1.33368890676572));
#29479=CARTESIAN_POINT('Ctrl Pts',(-1.6496563728683,1.,-1.33494590467993));
#29480=CARTESIAN_POINT('Ctrl Pts',(-1.65586025952593,1.,-1.33616559745172));
#29481=CARTESIAN_POINT('Ctrl Pts',(-1.66208312541983,1.,-1.33734820885262));
#29482=CARTESIAN_POINT('Ctrl Pts',(-1.66832460783989,1.,-1.33849388654388));
#29483=CARTESIAN_POINT('Ctrl Pts',(-1.67458429426086,1.,-1.3396027347034));
#29484=CARTESIAN_POINT('Ctrl Pts',(-1.68086176030362,1.,-1.34067485185203));
#29485=CARTESIAN_POINT('Ctrl Pts',(-1.68715660868764,1.,-1.341710374848));
#29486=CARTESIAN_POINT('Ctrl Pts',(-1.6934684849687,1.,-1.34270948206319));
#29487=CARTESIAN_POINT('Ctrl Pts',(-1.69979707754427,1.,-1.34367237124483));
#29488=CARTESIAN_POINT('Ctrl Pts',(-1.70614212266738,1.,-1.34459924533831));
#29489=CARTESIAN_POINT('Ctrl Pts',(-1.71250340686822,1.,-1.34549029589416));
#29490=CARTESIAN_POINT('Ctrl Pts',(-1.7188807715049,1.,-1.34634568653227));
#29491=CARTESIAN_POINT('Ctrl Pts',(-1.72527410680674,1.,-1.34716554819527));
#29492=CARTESIAN_POINT('Ctrl Pts',(-1.7304014965394,1.,-1.34779309152035));
#29493=CARTESIAN_POINT('Ctrl Pts',(-1.73425417885907,1.,-1.34824783112887));
#29494=CARTESIAN_POINT('Ctrl Pts',(-1.73682580585691,1.,-1.34854391898045));
#29495=CARTESIAN_POINT('Ctrl Pts',(-1.73811241238545,1.,-1.34869019493419));
#29496=CARTESIAN_POINT('',(-1.31362392696032,0.,-1.15624053661742));
#29497=CARTESIAN_POINT('Origin',(0.,0.,0.));
#29498=CARTESIAN_POINT('',(-1.15624053661742,1.,-1.31362392696033));
#29499=CARTESIAN_POINT('Origin',(0.,1.,0.));
#29500=CARTESIAN_POINT('',(-1.15624053661742,0.,-1.31362392696033));
#29501=CARTESIAN_POINT('Ctrl Pts',(-1.34869019493419,-1.,-1.73811241238545));
#29502=CARTESIAN_POINT('Ctrl Pts',(-1.34869019493419,1.,-1.73811241238545));
#29503=CARTESIAN_POINT('Ctrl Pts',(-1.34854391898145,-1.,-1.73682580585819));
#29504=CARTESIAN_POINT('Ctrl Pts',(-1.34854391898145,1.,-1.73682580585819));
#29505=CARTESIAN_POINT('Ctrl Pts',(-1.34824783113158,-1.,-1.73425417886255));
#29506=CARTESIAN_POINT('Ctrl Pts',(-1.34824783113158,1.,-1.73425417886255));
#29507=CARTESIAN_POINT('Ctrl Pts',(-1.3477930915247,-1.,-1.73040149654497));
#29508=CARTESIAN_POINT('Ctrl Pts',(-1.3477930915247,1.,-1.73040149654497));
#29509=CARTESIAN_POINT('Ctrl Pts',(-1.34716554820013,-1.,-1.72527410681298));
#29510=CARTESIAN_POINT('Ctrl Pts',(-1.34716554820013,1.,-1.72527410681298));
#29511=CARTESIAN_POINT('Ctrl Pts',(-1.34634568653586,-1.,-1.7188807715095));
#29512=CARTESIAN_POINT('Ctrl Pts',(-1.34634568653586,1.,-1.7188807715095));
#29513=CARTESIAN_POINT('Ctrl Pts',(-1.34549029589563,-1.,-1.71250340687011));
#29514=CARTESIAN_POINT('Ctrl Pts',(-1.34549029589563,1.,-1.71250340687011));
#29515=CARTESIAN_POINT('Ctrl Pts',(-1.34459924533783,-1.,-1.70614212266676));
#29516=CARTESIAN_POINT('Ctrl Pts',(-1.34459924533783,1.,-1.70614212266676));
#29517=CARTESIAN_POINT('Ctrl Pts',(-1.34367237124322,-1.,-1.69979707754221));
#29518=CARTESIAN_POINT('Ctrl Pts',(-1.34367237124322,1.,-1.69979707754221));
#29519=CARTESIAN_POINT('Ctrl Pts',(-1.34270948206139,-1.,-1.6934684849664));
#29520=CARTESIAN_POINT('Ctrl Pts',(-1.34270948206139,1.,-1.6934684849664));
#29521=CARTESIAN_POINT('Ctrl Pts',(-1.34171037484673,-1.,-1.68715660868602));
#29522=CARTESIAN_POINT('Ctrl Pts',(-1.34171037484673,1.,-1.68715660868602));
#29523=CARTESIAN_POINT('Ctrl Pts',(-1.3406748518516,-1.,-1.68086176030308));
#29524=CARTESIAN_POINT('Ctrl Pts',(-1.3406748518516,1.,-1.68086176030308));
#29525=CARTESIAN_POINT('Ctrl Pts',(-1.33960273470372,-1.,-1.67458429426126));
#29526=CARTESIAN_POINT('Ctrl Pts',(-1.33960273470372,1.,-1.67458429426126));
#29527=CARTESIAN_POINT('Ctrl Pts',(-1.33849388654458,-1.,-1.66832460784078));
#29528=CARTESIAN_POINT('Ctrl Pts',(-1.33849388654458,1.,-1.66832460784078));
#29529=CARTESIAN_POINT('Ctrl Pts',(-1.33734820885331,-1.,-1.66208312542073));
#29530=CARTESIAN_POINT('Ctrl Pts',(-1.33734820885331,1.,-1.66208312542073));
#29531=CARTESIAN_POINT('Ctrl Pts',(-1.33616559745217,-1.,-1.65586025952651));
#29532=CARTESIAN_POINT('Ctrl Pts',(-1.33616559745217,1.,-1.65586025952651));
#29533=CARTESIAN_POINT('Ctrl Pts',(-1.33494590468003,-1.,-1.64965637286843));
#29534=CARTESIAN_POINT('Ctrl Pts',(-1.33494590468003,1.,-1.64965637286843));
#29535=CARTESIAN_POINT('Ctrl Pts',(-1.33368890676554,-1.,-1.64347174856007));
#29536=CARTESIAN_POINT('Ctrl Pts',(-1.33368890676554,1.,-1.64347174856007));
#29537=CARTESIAN_POINT('Ctrl Pts',(-1.33239425103694,-1.,-1.6373065347505));
#29538=CARTESIAN_POINT('Ctrl Pts',(-1.33239425103694,1.,-1.6373065347505));
#29539=CARTESIAN_POINT('Ctrl Pts',(-1.33106149345618,-1.,-1.63116079730887));
#29540=CARTESIAN_POINT('Ctrl Pts',(-1.33106149345618,1.,-1.63116079730887));
#29541=CARTESIAN_POINT('Ctrl Pts',(-1.32969019505665,-1.,-1.62503464209777));
#29542=CARTESIAN_POINT('Ctrl Pts',(-1.32969019505665,1.,-1.62503464209777));
#29543=CARTESIAN_POINT('Ctrl Pts',(-1.32828000610448,-1.,-1.61892832270723));
#29544=CARTESIAN_POINT('Ctrl Pts',(-1.32828000610448,1.,-1.61892832270723));
#29545=CARTESIAN_POINT('Ctrl Pts',(-1.32683074483365,-1.,-1.61284234015762));
#29546=CARTESIAN_POINT('Ctrl Pts',(-1.32683074483365,1.,-1.61284234015762));
#29547=CARTESIAN_POINT('Ctrl Pts',(-1.32534250785794,-1.,-1.6067775829097));
#29548=CARTESIAN_POINT('Ctrl Pts',(-1.32534250785794,1.,-1.6067775829097));
#29549=CARTESIAN_POINT('Ctrl Pts',(-1.32381550858266,-1.,-1.600735118587));
#29550=CARTESIAN_POINT('Ctrl Pts',(-1.32381550858266,1.,-1.600735118587));
#29551=CARTESIAN_POINT('Ctrl Pts',(-1.32224985747686,-1.,-1.59471591079408));
#29552=CARTESIAN_POINT('Ctrl Pts',(-1.32224985747686,1.,-1.59471591079408));
#29553=CARTESIAN_POINT('Ctrl Pts',(-1.32064537110891,-1.,-1.58872057258244));
#29554=CARTESIAN_POINT('Ctrl Pts',(-1.32064537110891,1.,-1.58872057258244));
#29555=CARTESIAN_POINT('Ctrl Pts',(-1.31900135021428,-1.,-1.58274907898829));
#29556=CARTESIAN_POINT('Ctrl Pts',(-1.31900135021428,1.,-1.58274907898829));
#29557=CARTESIAN_POINT('Ctrl Pts',(-1.31731642317183,-1.,-1.57680056505585));
#29558=CARTESIAN_POINT('Ctrl Pts',(-1.31731642317183,1.,-1.57680056505585));
#29559=CARTESIAN_POINT('Ctrl Pts',(-1.31558903860015,-1.,-1.57087397835721));
#29560=CARTESIAN_POINT('Ctrl Pts',(-1.31558903860015,1.,-1.57087397835721));
#29561=CARTESIAN_POINT('Ctrl Pts',(-1.31381795281002,-1.,-1.56496872402352));
#29562=CARTESIAN_POINT('Ctrl Pts',(-1.31381795281002,1.,-1.56496872402352));
#29563=CARTESIAN_POINT('Ctrl Pts',(-1.31200264341696,-1.,-1.55908521254822));
#29564=CARTESIAN_POINT('Ctrl Pts',(-1.31200264341696,1.,-1.55908521254822));
#29565=CARTESIAN_POINT('Ctrl Pts',(-1.31014393684221,-1.,-1.55322568759481));
#29566=CARTESIAN_POINT('Ctrl Pts',(-1.31014393684221,1.,-1.55322568759481));
#29567=CARTESIAN_POINT('Ctrl Pts',(-1.30824393907471,-1.,-1.54739413957183));
#29568=CARTESIAN_POINT('Ctrl Pts',(-1.30824393907471,1.,-1.54739413957183));
#29569=CARTESIAN_POINT('Ctrl Pts',(-1.30630475189553,-1.,-1.54159462645428));
#29570=CARTESIAN_POINT('Ctrl Pts',(-1.30630475189553,1.,-1.54159462645428));
#29571=CARTESIAN_POINT('Ctrl Pts',(-1.30432735639487,-1.,-1.53582981268976));
#29572=CARTESIAN_POINT('Ctrl Pts',(-1.30432735639487,1.,-1.53582981268976));
#29573=CARTESIAN_POINT('Ctrl Pts',(-1.3023106439557,-1.,-1.53009970283893));
#29574=CARTESIAN_POINT('Ctrl Pts',(-1.3023106439557,1.,-1.53009970283893));
#29575=CARTESIAN_POINT('Ctrl Pts',(-1.30024984366334,-1.,-1.5243995786107));
#29576=CARTESIAN_POINT('Ctrl Pts',(-1.30024984366334,1.,-1.5243995786107));
#29577=CARTESIAN_POINT('Ctrl Pts',(-1.29813791800757,-1.,-1.51872184912735));
#29578=CARTESIAN_POINT('Ctrl Pts',(-1.29813791800757,1.,-1.51872184912735));
#29579=CARTESIAN_POINT('Ctrl Pts',(-1.29596850710518,-1.,-1.51305994241412));
#29580=CARTESIAN_POINT('Ctrl Pts',(-1.29596850710518,1.,-1.51305994241412));
#29581=CARTESIAN_POINT('Ctrl Pts',(-1.29373841372843,-1.,-1.50741159078367));
#29582=CARTESIAN_POINT('Ctrl Pts',(-1.29373841372843,1.,-1.50741159078367));
#29583=CARTESIAN_POINT('Ctrl Pts',(-1.29145022885171,-1.,-1.50178230149764));
#29584=CARTESIAN_POINT('Ctrl Pts',(-1.29145022885171,1.,-1.50178230149764));
#29585=CARTESIAN_POINT('Ctrl Pts',(-1.28911506584232,-1.,-1.49618896881729));
#29586=CARTESIAN_POINT('Ctrl Pts',(-1.28911506584232,1.,-1.49618896881729));
#29587=CARTESIAN_POINT('Ctrl Pts',(-1.28674676116415,-1.,-1.4906522831275));
#29588=CARTESIAN_POINT('Ctrl Pts',(-1.28674676116415,1.,-1.4906522831275));
#29589=CARTESIAN_POINT('Ctrl Pts',(-1.28435533880184,-1.,-1.48518817118891));
#29590=CARTESIAN_POINT('Ctrl Pts',(-1.28435533880184,1.,-1.48518817118891));
#29591=CARTESIAN_POINT('Ctrl Pts',(-1.28194158939522,-1.,-1.47980070347102));
#29592=CARTESIAN_POINT('Ctrl Pts',(-1.28194158939522,1.,-1.47980070347102));
#29593=CARTESIAN_POINT('Ctrl Pts',(-1.27948918248524,-1.,-1.4744717526711));
#29594=CARTESIAN_POINT('Ctrl Pts',(-1.27948918248524,1.,-1.4744717526711));
#29595=CARTESIAN_POINT('Ctrl Pts',(-1.27696414831144,-1.,-1.46916035917197));
#29596=CARTESIAN_POINT('Ctrl Pts',(-1.27696414831144,1.,-1.46916035917197));
#29597=CARTESIAN_POINT('Ctrl Pts',(-1.27433119897877,-1.,-1.4638243133254));
#29598=CARTESIAN_POINT('Ctrl Pts',(-1.27433119897877,1.,-1.4638243133254));
#29599=CARTESIAN_POINT('Ctrl Pts',(-1.27156805265312,-1.,-1.45843906294725));
#29600=CARTESIAN_POINT('Ctrl Pts',(-1.27156805265312,1.,-1.45843906294725));
#29601=CARTESIAN_POINT('Ctrl Pts',(-1.26867786804854,-1.,-1.45301422764205));
#29602=CARTESIAN_POINT('Ctrl Pts',(-1.26867786804854,1.,-1.45301422764205));
#29603=CARTESIAN_POINT('Ctrl Pts',(-1.26570925118767,-1.,-1.44761985001544));
#29604=CARTESIAN_POINT('Ctrl Pts',(-1.26570925118767,1.,-1.44761985001544));
#29605=CARTESIAN_POINT('Ctrl Pts',(-1.26273903323723,-1.,-1.44236470511145));
#29606=CARTESIAN_POINT('Ctrl Pts',(-1.26273903323723,1.,-1.44236470511145));
#29607=CARTESIAN_POINT('Ctrl Pts',(-1.25983531011894,-1.,-1.43734919180719));
#29608=CARTESIAN_POINT('Ctrl Pts',(-1.25983531011894,1.,-1.43734919180719));
#29609=CARTESIAN_POINT('Ctrl Pts',(-1.25702687965744,-1.,-1.43262645609679));
#29610=CARTESIAN_POINT('Ctrl Pts',(-1.25702687965744,1.,-1.43262645609679));
#29611=CARTESIAN_POINT('Ctrl Pts',(-1.25426945222783,-1.,-1.42815938799555));
#29612=CARTESIAN_POINT('Ctrl Pts',(-1.25426945222783,1.,-1.42815938799555));
#29613=CARTESIAN_POINT('Ctrl Pts',(-1.25141455570299,-1.,-1.42378102115911));
#29614=CARTESIAN_POINT('Ctrl Pts',(-1.25141455570299,1.,-1.42378102115911));
#29615=CARTESIAN_POINT('Ctrl Pts',(-1.24824430986911,-1.,-1.41923722596421));
#29616=CARTESIAN_POINT('Ctrl Pts',(-1.24824430986911,1.,-1.41923722596421));
#29617=CARTESIAN_POINT('Ctrl Pts',(-1.24450600513278,-1.,-1.41422913175437));
#29618=CARTESIAN_POINT('Ctrl Pts',(-1.24450600513278,1.,-1.41422913175437));
#29619=CARTESIAN_POINT('Ctrl Pts',(-1.23994455029421,-1.,-1.40845295531151));
#29620=CARTESIAN_POINT('Ctrl Pts',(-1.23994455029421,1.,-1.40845295531151));
#29621=CARTESIAN_POINT('Ctrl Pts',(-1.23434087289768,-1.,-1.40164708205345));
#29622=CARTESIAN_POINT('Ctrl Pts',(-1.23434087289768,1.,-1.40164708205345));
#29623=CARTESIAN_POINT('Ctrl Pts',(-1.22752961898063,-1.,-1.39361389567257));
#29624=CARTESIAN_POINT('Ctrl Pts',(-1.22752961898063,1.,-1.39361389567257));
#29625=CARTESIAN_POINT('Ctrl Pts',(-1.21938737278853,-1.,-1.38420564525391));
#29626=CARTESIAN_POINT('Ctrl Pts',(-1.21938737278853,1.,-1.38420564525391));
#29627=CARTESIAN_POINT('Ctrl Pts',(-1.20982812923113,-1.,-1.37331915604962));
#29628=CARTESIAN_POINT('Ctrl Pts',(-1.20982812923113,1.,-1.37331915604962));
#29629=CARTESIAN_POINT('Ctrl Pts',(-1.1987959077656,-1.,-1.36088705040677));
#29630=CARTESIAN_POINT('Ctrl Pts',(-1.1987959077656,1.,-1.36088705040677));
#29631=CARTESIAN_POINT('Ctrl Pts',(-1.18625865664915,-1.,-1.34687053998157));
#29632=CARTESIAN_POINT('Ctrl Pts',(-1.18625865664915,1.,-1.34687053998157));
#29633=CARTESIAN_POINT('Ctrl Pts',(-1.17501305787994,-1.,-1.33437539344842));
#29634=CARTESIAN_POINT('Ctrl Pts',(-1.17501305787994,1.,-1.33437539344842));
#29635=CARTESIAN_POINT('Ctrl Pts',(-1.16589330092532,-1.,-1.32428080720544));
#29636=CARTESIAN_POINT('Ctrl Pts',(-1.16589330092532,1.,-1.32428080720544));
#29637=CARTESIAN_POINT('Ctrl Pts',(-1.15950888730433,-1.,-1.3172297721596));
#29638=CARTESIAN_POINT('Ctrl Pts',(-1.15950888730433,1.,-1.3172297721596));
#29639=CARTESIAN_POINT('Ctrl Pts',(-1.15624053661742,-1.,-1.31362392696033));
#29640=CARTESIAN_POINT('Ctrl Pts',(-1.15624053661742,1.,-1.31362392696033));
#29641=CARTESIAN_POINT('',(-1.34869019493419,1.,-1.73811241238545));
#29642=CARTESIAN_POINT('Ctrl Pts',(-1.34869019493419,1.,-1.73811241238545));
#29643=CARTESIAN_POINT('Ctrl Pts',(-1.34854391898145,1.,-1.73682580585819));
#29644=CARTESIAN_POINT('Ctrl Pts',(-1.34824783113158,1.,-1.73425417886255));
#29645=CARTESIAN_POINT('Ctrl Pts',(-1.3477930915247,1.,-1.73040149654497));
#29646=CARTESIAN_POINT('Ctrl Pts',(-1.34716554820013,1.,-1.72527410681298));
#29647=CARTESIAN_POINT('Ctrl Pts',(-1.34634568653586,1.,-1.7188807715095));
#29648=CARTESIAN_POINT('Ctrl Pts',(-1.34549029589563,1.,-1.71250340687011));
#29649=CARTESIAN_POINT('Ctrl Pts',(-1.34459924533783,1.,-1.70614212266676));
#29650=CARTESIAN_POINT('Ctrl Pts',(-1.34367237124322,1.,-1.69979707754221));
#29651=CARTESIAN_POINT('Ctrl Pts',(-1.34270948206139,1.,-1.6934684849664));
#29652=CARTESIAN_POINT('Ctrl Pts',(-1.34171037484673,1.,-1.68715660868602));
#29653=CARTESIAN_POINT('Ctrl Pts',(-1.3406748518516,1.,-1.68086176030308));
#29654=CARTESIAN_POINT('Ctrl Pts',(-1.33960273470372,1.,-1.67458429426126));
#29655=CARTESIAN_POINT('Ctrl Pts',(-1.33849388654458,1.,-1.66832460784078));
#29656=CARTESIAN_POINT('Ctrl Pts',(-1.33734820885331,1.,-1.66208312542073));
#29657=CARTESIAN_POINT('Ctrl Pts',(-1.33616559745217,1.,-1.65586025952651));
#29658=CARTESIAN_POINT('Ctrl Pts',(-1.33494590468003,1.,-1.64965637286843));
#29659=CARTESIAN_POINT('Ctrl Pts',(-1.33368890676554,1.,-1.64347174856007));
#29660=CARTESIAN_POINT('Ctrl Pts',(-1.33239425103694,1.,-1.6373065347505));
#29661=CARTESIAN_POINT('Ctrl Pts',(-1.33106149345618,1.,-1.63116079730887));
#29662=CARTESIAN_POINT('Ctrl Pts',(-1.32969019505665,1.,-1.62503464209777));
#29663=CARTESIAN_POINT('Ctrl Pts',(-1.32828000610448,1.,-1.61892832270723));
#29664=CARTESIAN_POINT('Ctrl Pts',(-1.32683074483365,1.,-1.61284234015762));
#29665=CARTESIAN_POINT('Ctrl Pts',(-1.32534250785794,1.,-1.6067775829097));
#29666=CARTESIAN_POINT('Ctrl Pts',(-1.32381550858266,1.,-1.600735118587));
#29667=CARTESIAN_POINT('Ctrl Pts',(-1.32224985747686,1.,-1.59471591079408));
#29668=CARTESIAN_POINT('Ctrl Pts',(-1.32064537110891,1.,-1.58872057258244));
#29669=CARTESIAN_POINT('Ctrl Pts',(-1.31900135021428,1.,-1.58274907898829));
#29670=CARTESIAN_POINT('Ctrl Pts',(-1.31731642317183,1.,-1.57680056505585));
#29671=CARTESIAN_POINT('Ctrl Pts',(-1.31558903860015,1.,-1.57087397835721));
#29672=CARTESIAN_POINT('Ctrl Pts',(-1.31381795281002,1.,-1.56496872402352));
#29673=CARTESIAN_POINT('Ctrl Pts',(-1.31200264341696,1.,-1.55908521254822));
#29674=CARTESIAN_POINT('Ctrl Pts',(-1.31014393684221,1.,-1.55322568759481));
#29675=CARTESIAN_POINT('Ctrl Pts',(-1.30824393907471,1.,-1.54739413957183));
#29676=CARTESIAN_POINT('Ctrl Pts',(-1.30630475189553,1.,-1.54159462645428));
#29677=CARTESIAN_POINT('Ctrl Pts',(-1.30432735639487,1.,-1.53582981268976));
#29678=CARTESIAN_POINT('Ctrl Pts',(-1.3023106439557,1.,-1.53009970283893));
#29679=CARTESIAN_POINT('Ctrl Pts',(-1.30024984366334,1.,-1.5243995786107));
#29680=CARTESIAN_POINT('Ctrl Pts',(-1.29813791800757,1.,-1.51872184912735));
#29681=CARTESIAN_POINT('Ctrl Pts',(-1.29596850710518,1.,-1.51305994241412));
#29682=CARTESIAN_POINT('Ctrl Pts',(-1.29373841372843,1.,-1.50741159078367));
#29683=CARTESIAN_POINT('Ctrl Pts',(-1.29145022885171,1.,-1.50178230149764));
#29684=CARTESIAN_POINT('Ctrl Pts',(-1.28911506584232,1.,-1.49618896881729));
#29685=CARTESIAN_POINT('Ctrl Pts',(-1.28674676116415,1.,-1.4906522831275));
#29686=CARTESIAN_POINT('Ctrl Pts',(-1.28435533880184,1.,-1.48518817118891));
#29687=CARTESIAN_POINT('Ctrl Pts',(-1.28194158939522,1.,-1.47980070347102));
#29688=CARTESIAN_POINT('Ctrl Pts',(-1.27948918248524,1.,-1.4744717526711));
#29689=CARTESIAN_POINT('Ctrl Pts',(-1.27696414831144,1.,-1.46916035917197));
#29690=CARTESIAN_POINT('Ctrl Pts',(-1.27433119897877,1.,-1.4638243133254));
#29691=CARTESIAN_POINT('Ctrl Pts',(-1.27156805265312,1.,-1.45843906294725));
#29692=CARTESIAN_POINT('Ctrl Pts',(-1.26867786804854,1.,-1.45301422764205));
#29693=CARTESIAN_POINT('Ctrl Pts',(-1.26570925118767,1.,-1.44761985001544));
#29694=CARTESIAN_POINT('Ctrl Pts',(-1.26273903323723,1.,-1.44236470511145));
#29695=CARTESIAN_POINT('Ctrl Pts',(-1.25983531011894,1.,-1.43734919180719));
#29696=CARTESIAN_POINT('Ctrl Pts',(-1.25702687965744,1.,-1.43262645609679));
#29697=CARTESIAN_POINT('Ctrl Pts',(-1.25426945222783,1.,-1.42815938799555));
#29698=CARTESIAN_POINT('Ctrl Pts',(-1.25141455570299,1.,-1.42378102115911));
#29699=CARTESIAN_POINT('Ctrl Pts',(-1.24824430986911,1.,-1.41923722596421));
#29700=CARTESIAN_POINT('Ctrl Pts',(-1.24450600513278,1.,-1.41422913175437));
#29701=CARTESIAN_POINT('Ctrl Pts',(-1.23994455029421,1.,-1.40845295531151));
#29702=CARTESIAN_POINT('Ctrl Pts',(-1.23434087289768,1.,-1.40164708205345));
#29703=CARTESIAN_POINT('Ctrl Pts',(-1.22752961898063,1.,-1.39361389567257));
#29704=CARTESIAN_POINT('Ctrl Pts',(-1.21938737278853,1.,-1.38420564525391));
#29705=CARTESIAN_POINT('Ctrl Pts',(-1.20982812923113,1.,-1.37331915604962));
#29706=CARTESIAN_POINT('Ctrl Pts',(-1.1987959077656,1.,-1.36088705040677));
#29707=CARTESIAN_POINT('Ctrl Pts',(-1.18625865664915,1.,-1.34687053998157));
#29708=CARTESIAN_POINT('Ctrl Pts',(-1.17501305787994,1.,-1.33437539344842));
#29709=CARTESIAN_POINT('Ctrl Pts',(-1.16589330092532,1.,-1.32428080720544));
#29710=CARTESIAN_POINT('Ctrl Pts',(-1.15950888730433,1.,-1.3172297721596));
#29711=CARTESIAN_POINT('Ctrl Pts',(-1.15624053661742,1.,-1.31362392696033));
#29712=CARTESIAN_POINT('',(-1.34869019493419,0.,-1.73811241238545));
#29713=CARTESIAN_POINT('Origin',(-1.23627494547115,0.,-1.81978687191668));
#29714=CARTESIAN_POINT('',(-1.23627494547115,1.,-1.81978687191668));
#29715=CARTESIAN_POINT('',(-1.34869019493419,1.,-1.73811241238545));
#29716=CARTESIAN_POINT('',(-1.23627494547115,0.,-1.81978687191668));
#29717=CARTESIAN_POINT('Ctrl Pts',(-0.892032620296855,-1.,-1.5055822144029));
#29718=CARTESIAN_POINT('Ctrl Pts',(-0.892032620296855,1.,-1.5055822144029));
#29719=CARTESIAN_POINT('Ctrl Pts',(-0.894452006967538,-1.,-1.50980486807181));
#29720=CARTESIAN_POINT('Ctrl Pts',(-0.894452006967538,1.,-1.50980486807181));
#29721=CARTESIAN_POINT('Ctrl Pts',(-0.89918504749193,-1.,-1.51805569591479));
#29722=CARTESIAN_POINT('Ctrl Pts',(-0.89918504749193,1.,-1.51805569591479));
#29723=CARTESIAN_POINT('Ctrl Pts',(-0.905967409640499,-1.,-1.52984849890434));
#29724=CARTESIAN_POINT('Ctrl Pts',(-0.905967409640499,1.,-1.52984849890434));
#29725=CARTESIAN_POINT('Ctrl Pts',(-0.91437591904658,-1.,-1.54440491152808));
#29726=CARTESIAN_POINT('Ctrl Pts',(-0.91437591904658,1.,-1.54440491152808));
#29727=CARTESIAN_POINT('Ctrl Pts',(-0.923832188966322,-1.,-1.56065988582509));
#29728=CARTESIAN_POINT('Ctrl Pts',(-0.923832188966322,1.,-1.56065988582509));
#29729=CARTESIAN_POINT('Ctrl Pts',(-0.932246680128849,-1.,-1.57499388385561));
#29730=CARTESIAN_POINT('Ctrl Pts',(-0.932246680128849,1.,-1.57499388385561));
#29731=CARTESIAN_POINT('Ctrl Pts',(-0.939646377909319,-1.,-1.58744937489796));
#29732=CARTESIAN_POINT('Ctrl Pts',(-0.939646377909319,1.,-1.58744937489796));
#29733=CARTESIAN_POINT('Ctrl Pts',(-0.946078063325796,-1.,-1.59810042045408));
#29734=CARTESIAN_POINT('Ctrl Pts',(-0.946078063325796,1.,-1.59810042045408));
#29735=CARTESIAN_POINT('Ctrl Pts',(-0.951613284361248,-1.,-1.60706069897794));
#29736=CARTESIAN_POINT('Ctrl Pts',(-0.951613284361248,1.,-1.60706069897794));
#29737=CARTESIAN_POINT('Ctrl Pts',(-0.956354422921573,-1.,-1.61449324337233));
#29738=CARTESIAN_POINT('Ctrl Pts',(-0.956354422921573,1.,-1.61449324337233));
#29739=CARTESIAN_POINT('Ctrl Pts',(-0.960438326099958,-1.,-1.62061638139929));
#29740=CARTESIAN_POINT('Ctrl Pts',(-0.960438326099958,1.,-1.62061638139929));
#29741=CARTESIAN_POINT('Ctrl Pts',(-0.964046107037821,-1.,-1.6257193066974));
#29742=CARTESIAN_POINT('Ctrl Pts',(-0.964046107037821,1.,-1.6257193066974));
#29743=CARTESIAN_POINT('Ctrl Pts',(-0.967387853228041,-1.,-1.63013849959083));
#29744=CARTESIAN_POINT('Ctrl Pts',(-0.967387853228041,1.,-1.63013849959083));
#29745=CARTESIAN_POINT('Ctrl Pts',(-0.970669715996356,-1.,-1.63420665729609));
#29746=CARTESIAN_POINT('Ctrl Pts',(-0.970669715996356,1.,-1.63420665729609));
#29747=CARTESIAN_POINT('Ctrl Pts',(-0.974066058287501,-1.,-1.63820952658157));
#29748=CARTESIAN_POINT('Ctrl Pts',(-0.974066058287501,1.,-1.63820952658157));
#29749=CARTESIAN_POINT('Ctrl Pts',(-0.977689794120297,-1.,-1.64233990826831));
#29750=CARTESIAN_POINT('Ctrl Pts',(-0.977689794120297,1.,-1.64233990826831));
#29751=CARTESIAN_POINT('Ctrl Pts',(-0.981562530940574,-1.,-1.64665139190834));
#29752=CARTESIAN_POINT('Ctrl Pts',(-0.981562530940574,1.,-1.64665139190834));
#29753=CARTESIAN_POINT('Ctrl Pts',(-0.985642622921626,-1.,-1.6511001661277));
#29754=CARTESIAN_POINT('Ctrl Pts',(-0.985642622921626,1.,-1.6511001661277));
#29755=CARTESIAN_POINT('Ctrl Pts',(-0.98985562785445,-1.,-1.65559044289746));
#29756=CARTESIAN_POINT('Ctrl Pts',(-0.98985562785445,1.,-1.65559044289746));
#29757=CARTESIAN_POINT('Ctrl Pts',(-0.994121836661116,-1.,-1.66001553809916));
#29758=CARTESIAN_POINT('Ctrl Pts',(-0.994121836661116,1.,-1.66001553809916));
#29759=CARTESIAN_POINT('Ctrl Pts',(-0.998389654952317,-1.,-1.66430758030304));
#29760=CARTESIAN_POINT('Ctrl Pts',(-0.998389654952317,1.,-1.66430758030304));
#29761=CARTESIAN_POINT('Ctrl Pts',(-1.00265091003682,-1.,-1.66846059277231));
#29762=CARTESIAN_POINT('Ctrl Pts',(-1.00265091003682,1.,-1.66846059277231));
#29763=CARTESIAN_POINT('Ctrl Pts',(-1.00692206696387,-1.,-1.67250335383248));
#29764=CARTESIAN_POINT('Ctrl Pts',(-1.00692206696387,1.,-1.67250335383248));
#29765=CARTESIAN_POINT('Ctrl Pts',(-1.01123236493507,-1.,-1.67648246776457));
#29766=CARTESIAN_POINT('Ctrl Pts',(-1.01123236493507,1.,-1.67648246776457));
#29767=CARTESIAN_POINT('Ctrl Pts',(-1.01561026162787,-1.,-1.6804428989482));
#29768=CARTESIAN_POINT('Ctrl Pts',(-1.01561026162787,1.,-1.6804428989482));
#29769=CARTESIAN_POINT('Ctrl Pts',(-1.02006795074222,-1.,-1.68440578021739));
#29770=CARTESIAN_POINT('Ctrl Pts',(-1.02006795074222,1.,-1.68440578021739));
#29771=CARTESIAN_POINT('Ctrl Pts',(-1.02460180535272,-1.,-1.68836910178475));
#29772=CARTESIAN_POINT('Ctrl Pts',(-1.02460180535272,1.,-1.68836910178475));
#29773=CARTESIAN_POINT('Ctrl Pts',(-1.02919977579155,-1.,-1.69231840863471));
#29774=CARTESIAN_POINT('Ctrl Pts',(-1.02919977579155,1.,-1.69231840863471));
#29775=CARTESIAN_POINT('Ctrl Pts',(-1.03384646003587,-1.,-1.69623414782769));
#29776=CARTESIAN_POINT('Ctrl Pts',(-1.03384646003587,1.,-1.69623414782769));
#29777=CARTESIAN_POINT('Ctrl Pts',(-1.03852922490782,-1.,-1.70010052930951));
#29778=CARTESIAN_POINT('Ctrl Pts',(-1.03852922490782,1.,-1.70010052930951));
#29779=CARTESIAN_POINT('Ctrl Pts',(-1.04324363334546,-1.,-1.70391338707969));
#29780=CARTESIAN_POINT('Ctrl Pts',(-1.04324363334546,1.,-1.70391338707969));
#29781=CARTESIAN_POINT('Ctrl Pts',(-1.0479908540499,-1.,-1.70767646263641));
#29782=CARTESIAN_POINT('Ctrl Pts',(-1.0479908540499,1.,-1.70767646263641));
#29783=CARTESIAN_POINT('Ctrl Pts',(-1.05277517202854,-1.,-1.71139783543986));
#29784=CARTESIAN_POINT('Ctrl Pts',(-1.05277517202854,1.,-1.71139783543986));
#29785=CARTESIAN_POINT('Ctrl Pts',(-1.05760163192481,-1.,-1.71508654427022));
#29786=CARTESIAN_POINT('Ctrl Pts',(-1.05760163192481,1.,-1.71508654427022));
#29787=CARTESIAN_POINT('Ctrl Pts',(-1.0624732468065,-1.,-1.71874858456908));
#29788=CARTESIAN_POINT('Ctrl Pts',(-1.0624732468065,1.,-1.71874858456908));
#29789=CARTESIAN_POINT('Ctrl Pts',(-1.06738966975463,-1.,-1.72238500928456));
#29790=CARTESIAN_POINT('Ctrl Pts',(-1.06738966975463,1.,-1.72238500928456));
#29791=CARTESIAN_POINT('Ctrl Pts',(-1.07234866990252,-1.,-1.72599406198489));
#29792=CARTESIAN_POINT('Ctrl Pts',(-1.07234866990252,1.,-1.72599406198489));
#29793=CARTESIAN_POINT('Ctrl Pts',(-1.0773470373727,-1.,-1.72957248977424));
#29794=CARTESIAN_POINT('Ctrl Pts',(-1.0773470373727,1.,-1.72957248977424));
#29795=CARTESIAN_POINT('Ctrl Pts',(-1.08238162784749,-1.,-1.73311705663407));
#29796=CARTESIAN_POINT('Ctrl Pts',(-1.08238162784749,1.,-1.73311705663407));
#29797=CARTESIAN_POINT('Ctrl Pts',(-1.08745056285429,-1.,-1.73662628326093));
#29798=CARTESIAN_POINT('Ctrl Pts',(-1.08745056285429,1.,-1.73662628326093));
#29799=CARTESIAN_POINT('Ctrl Pts',(-1.09255329056496,-1.,-1.74010053962252));
#29800=CARTESIAN_POINT('Ctrl Pts',(-1.09255329056496,1.,-1.74010053962252));
#29801=CARTESIAN_POINT('Ctrl Pts',(-1.09768999241229,-1.,-1.74354119236212));
#29802=CARTESIAN_POINT('Ctrl Pts',(-1.09768999241229,1.,-1.74354119236212));
#29803=CARTESIAN_POINT('Ctrl Pts',(-1.10286118991144,-1.,-1.74695004214924));
#29804=CARTESIAN_POINT('Ctrl Pts',(-1.10286118991144,1.,-1.74695004214924));
#29805=CARTESIAN_POINT('Ctrl Pts',(-1.10806728183003,-1.,-1.75032866075914));
#29806=CARTESIAN_POINT('Ctrl Pts',(-1.10806728183003,1.,-1.75032866075914));
#29807=CARTESIAN_POINT('Ctrl Pts',(-1.11330807582542,-1.,-1.75367772094617));
#29808=CARTESIAN_POINT('Ctrl Pts',(-1.11330807582542,1.,-1.75367772094617));
#29809=CARTESIAN_POINT('Ctrl Pts',(-1.11858293216752,-1.,-1.75699720772089));
#29810=CARTESIAN_POINT('Ctrl Pts',(-1.11858293216752,1.,-1.75699720772089));
#29811=CARTESIAN_POINT('Ctrl Pts',(-1.12389096855078,-1.,-1.76028671825084));
#29812=CARTESIAN_POINT('Ctrl Pts',(-1.12389096855078,1.,-1.76028671825084));
#29813=CARTESIAN_POINT('Ctrl Pts',(-1.12923123555076,-1.,-1.76354571966171));
#29814=CARTESIAN_POINT('Ctrl Pts',(-1.12923123555076,1.,-1.76354571966171));
#29815=CARTESIAN_POINT('Ctrl Pts',(-1.13460291804635,-1.,-1.76677384551883));
#29816=CARTESIAN_POINT('Ctrl Pts',(-1.13460291804635,1.,-1.76677384551883));
#29817=CARTESIAN_POINT('Ctrl Pts',(-1.14000548337,-1.,-1.76997111386806));
#29818=CARTESIAN_POINT('Ctrl Pts',(-1.14000548337,1.,-1.76997111386806));
#29819=CARTESIAN_POINT('Ctrl Pts',(-1.14543858226948,-1.,-1.77313777896234));
#29820=CARTESIAN_POINT('Ctrl Pts',(-1.14543858226948,1.,-1.77313777896234));
#29821=CARTESIAN_POINT('Ctrl Pts',(-1.15090197841531,-1.,-1.77627422557034));
#29822=CARTESIAN_POINT('Ctrl Pts',(-1.15090197841531,1.,-1.77627422557034));
#29823=CARTESIAN_POINT('Ctrl Pts',(-1.15639547194689,-1.,-1.77938085564261));
#29824=CARTESIAN_POINT('Ctrl Pts',(-1.15639547194689,1.,-1.77938085564261));
#29825=CARTESIAN_POINT('Ctrl Pts',(-1.16191881298458,-1.,-1.78245795880949));
#29826=CARTESIAN_POINT('Ctrl Pts',(-1.16191881298458,1.,-1.78245795880949));
#29827=CARTESIAN_POINT('Ctrl Pts',(-1.16747166312239,-1.,-1.78550566040349));
#29828=CARTESIAN_POINT('Ctrl Pts',(-1.16747166312239,1.,-1.78550566040349));
#29829=CARTESIAN_POINT('Ctrl Pts',(-1.17305363177265,-1.,-1.78852398877523));
#29830=CARTESIAN_POINT('Ctrl Pts',(-1.17305363177265,1.,-1.78852398877523));
#29831=CARTESIAN_POINT('Ctrl Pts',(-1.17866429440781,-1.,-1.79151291552646));
#29832=CARTESIAN_POINT('Ctrl Pts',(-1.17866429440781,1.,-1.79151291552646));
#29833=CARTESIAN_POINT('Ctrl Pts',(-1.18430321697471,-1.,-1.79447240321572));
#29834=CARTESIAN_POINT('Ctrl Pts',(-1.18430321697471,1.,-1.79447240321572));
#29835=CARTESIAN_POINT('Ctrl Pts',(-1.1899699793456,-1.,-1.79740245923649));
#29836=CARTESIAN_POINT('Ctrl Pts',(-1.1899699793456,1.,-1.79740245923649));
#29837=CARTESIAN_POINT('Ctrl Pts',(-1.19566418930405,-1.,-1.80030314370121));
#29838=CARTESIAN_POINT('Ctrl Pts',(-1.19566418930405,1.,-1.80030314370121));
#29839=CARTESIAN_POINT('Ctrl Pts',(-1.2013854893912,-1.,-1.8031745483882));
#29840=CARTESIAN_POINT('Ctrl Pts',(-1.2013854893912,1.,-1.8031745483882));
#29841=CARTESIAN_POINT('Ctrl Pts',(-1.20713356605519,-1.,-1.80601678480772));
#29842=CARTESIAN_POINT('Ctrl Pts',(-1.20713356605519,1.,-1.80601678480772));
#29843=CARTESIAN_POINT('Ctrl Pts',(-1.2129081570818,-1.,-1.80882996916931));
#29844=CARTESIAN_POINT('Ctrl Pts',(-1.2129081570818,1.,-1.80882996916931));
#29845=CARTESIAN_POINT('Ctrl Pts',(-1.2187090610323,-1.,-1.81161420806172));
#29846=CARTESIAN_POINT('Ctrl Pts',(-1.2187090610323,1.,-1.81161420806172));
#29847=CARTESIAN_POINT('Ctrl Pts',(-1.22453613304507,-1.,-1.81436959209778));
#29848=CARTESIAN_POINT('Ctrl Pts',(-1.22453613304507,1.,-1.81436959209778));
#29849=CARTESIAN_POINT('Ctrl Pts',(-1.22921864890975,-1.,-1.81655087183054));
#29850=CARTESIAN_POINT('Ctrl Pts',(-1.22921864890975,1.,-1.81655087183054));
#29851=CARTESIAN_POINT('Ctrl Pts',(-1.23274224526804,-1.,-1.81817389920914));
#29852=CARTESIAN_POINT('Ctrl Pts',(-1.23274224526804,1.,-1.81817389920914));
#29853=CARTESIAN_POINT('Ctrl Pts',(-1.23509651170384,-1.,-1.81925017193531));
#29854=CARTESIAN_POINT('Ctrl Pts',(-1.23509651170384,1.,-1.81925017193531));
#29855=CARTESIAN_POINT('Ctrl Pts',(-1.23627494547115,-1.,-1.81978687191668));
#29856=CARTESIAN_POINT('Ctrl Pts',(-1.23627494547115,1.,-1.81978687191668));
#29857=CARTESIAN_POINT('',(-0.892032620296855,1.,-1.5055822144029));
#29858=CARTESIAN_POINT('Ctrl Pts',(-0.892032620296855,1.,-1.5055822144029));
#29859=CARTESIAN_POINT('Ctrl Pts',(-0.894452006967538,1.,-1.50980486807181));
#29860=CARTESIAN_POINT('Ctrl Pts',(-0.89918504749193,1.,-1.51805569591479));
#29861=CARTESIAN_POINT('Ctrl Pts',(-0.905967409640499,1.,-1.52984849890434));
#29862=CARTESIAN_POINT('Ctrl Pts',(-0.91437591904658,1.,-1.54440491152808));
#29863=CARTESIAN_POINT('Ctrl Pts',(-0.923832188966322,1.,-1.56065988582509));
#29864=CARTESIAN_POINT('Ctrl Pts',(-0.932246680128849,1.,-1.57499388385561));
#29865=CARTESIAN_POINT('Ctrl Pts',(-0.939646377909319,1.,-1.58744937489796));
#29866=CARTESIAN_POINT('Ctrl Pts',(-0.946078063325796,1.,-1.59810042045408));
#29867=CARTESIAN_POINT('Ctrl Pts',(-0.951613284361248,1.,-1.60706069897794));
#29868=CARTESIAN_POINT('Ctrl Pts',(-0.956354422921573,1.,-1.61449324337233));
#29869=CARTESIAN_POINT('Ctrl Pts',(-0.960438326099958,1.,-1.62061638139929));
#29870=CARTESIAN_POINT('Ctrl Pts',(-0.964046107037821,1.,-1.6257193066974));
#29871=CARTESIAN_POINT('Ctrl Pts',(-0.967387853228041,1.,-1.63013849959083));
#29872=CARTESIAN_POINT('Ctrl Pts',(-0.970669715996356,1.,-1.63420665729609));
#29873=CARTESIAN_POINT('Ctrl Pts',(-0.974066058287501,1.,-1.63820952658157));
#29874=CARTESIAN_POINT('Ctrl Pts',(-0.977689794120297,1.,-1.64233990826831));
#29875=CARTESIAN_POINT('Ctrl Pts',(-0.981562530940574,1.,-1.64665139190834));
#29876=CARTESIAN_POINT('Ctrl Pts',(-0.985642622921626,1.,-1.6511001661277));
#29877=CARTESIAN_POINT('Ctrl Pts',(-0.98985562785445,1.,-1.65559044289746));
#29878=CARTESIAN_POINT('Ctrl Pts',(-0.994121836661116,1.,-1.66001553809916));
#29879=CARTESIAN_POINT('Ctrl Pts',(-0.998389654952317,1.,-1.66430758030304));
#29880=CARTESIAN_POINT('Ctrl Pts',(-1.00265091003682,1.,-1.66846059277231));
#29881=CARTESIAN_POINT('Ctrl Pts',(-1.00692206696387,1.,-1.67250335383248));
#29882=CARTESIAN_POINT('Ctrl Pts',(-1.01123236493507,1.,-1.67648246776457));
#29883=CARTESIAN_POINT('Ctrl Pts',(-1.01561026162787,1.,-1.6804428989482));
#29884=CARTESIAN_POINT('Ctrl Pts',(-1.02006795074222,1.,-1.68440578021739));
#29885=CARTESIAN_POINT('Ctrl Pts',(-1.02460180535272,1.,-1.68836910178475));
#29886=CARTESIAN_POINT('Ctrl Pts',(-1.02919977579155,1.,-1.69231840863471));
#29887=CARTESIAN_POINT('Ctrl Pts',(-1.03384646003587,1.,-1.69623414782769));
#29888=CARTESIAN_POINT('Ctrl Pts',(-1.03852922490782,1.,-1.70010052930951));
#29889=CARTESIAN_POINT('Ctrl Pts',(-1.04324363334546,1.,-1.70391338707969));
#29890=CARTESIAN_POINT('Ctrl Pts',(-1.0479908540499,1.,-1.70767646263641));
#29891=CARTESIAN_POINT('Ctrl Pts',(-1.05277517202854,1.,-1.71139783543986));
#29892=CARTESIAN_POINT('Ctrl Pts',(-1.05760163192481,1.,-1.71508654427022));
#29893=CARTESIAN_POINT('Ctrl Pts',(-1.0624732468065,1.,-1.71874858456908));
#29894=CARTESIAN_POINT('Ctrl Pts',(-1.06738966975463,1.,-1.72238500928456));
#29895=CARTESIAN_POINT('Ctrl Pts',(-1.07234866990252,1.,-1.72599406198489));
#29896=CARTESIAN_POINT('Ctrl Pts',(-1.0773470373727,1.,-1.72957248977424));
#29897=CARTESIAN_POINT('Ctrl Pts',(-1.08238162784749,1.,-1.73311705663407));
#29898=CARTESIAN_POINT('Ctrl Pts',(-1.08745056285429,1.,-1.73662628326093));
#29899=CARTESIAN_POINT('Ctrl Pts',(-1.09255329056496,1.,-1.74010053962252));
#29900=CARTESIAN_POINT('Ctrl Pts',(-1.09768999241229,1.,-1.74354119236212));
#29901=CARTESIAN_POINT('Ctrl Pts',(-1.10286118991144,1.,-1.74695004214924));
#29902=CARTESIAN_POINT('Ctrl Pts',(-1.10806728183003,1.,-1.75032866075914));
#29903=CARTESIAN_POINT('Ctrl Pts',(-1.11330807582542,1.,-1.75367772094617));
#29904=CARTESIAN_POINT('Ctrl Pts',(-1.11858293216752,1.,-1.75699720772089));
#29905=CARTESIAN_POINT('Ctrl Pts',(-1.12389096855078,1.,-1.76028671825084));
#29906=CARTESIAN_POINT('Ctrl Pts',(-1.12923123555076,1.,-1.76354571966171));
#29907=CARTESIAN_POINT('Ctrl Pts',(-1.13460291804635,1.,-1.76677384551883));
#29908=CARTESIAN_POINT('Ctrl Pts',(-1.14000548337,1.,-1.76997111386806));
#29909=CARTESIAN_POINT('Ctrl Pts',(-1.14543858226948,1.,-1.77313777896234));
#29910=CARTESIAN_POINT('Ctrl Pts',(-1.15090197841531,1.,-1.77627422557034));
#29911=CARTESIAN_POINT('Ctrl Pts',(-1.15639547194689,1.,-1.77938085564261));
#29912=CARTESIAN_POINT('Ctrl Pts',(-1.16191881298458,1.,-1.78245795880949));
#29913=CARTESIAN_POINT('Ctrl Pts',(-1.16747166312239,1.,-1.78550566040349));
#29914=CARTESIAN_POINT('Ctrl Pts',(-1.17305363177265,1.,-1.78852398877523));
#29915=CARTESIAN_POINT('Ctrl Pts',(-1.17866429440781,1.,-1.79151291552646));
#29916=CARTESIAN_POINT('Ctrl Pts',(-1.18430321697471,1.,-1.79447240321572));
#29917=CARTESIAN_POINT('Ctrl Pts',(-1.1899699793456,1.,-1.79740245923649));
#29918=CARTESIAN_POINT('Ctrl Pts',(-1.19566418930405,1.,-1.80030314370121));
#29919=CARTESIAN_POINT('Ctrl Pts',(-1.2013854893912,1.,-1.8031745483882));
#29920=CARTESIAN_POINT('Ctrl Pts',(-1.20713356605519,1.,-1.80601678480772));
#29921=CARTESIAN_POINT('Ctrl Pts',(-1.2129081570818,1.,-1.80882996916931));
#29922=CARTESIAN_POINT('Ctrl Pts',(-1.2187090610323,1.,-1.81161420806172));
#29923=CARTESIAN_POINT('Ctrl Pts',(-1.22453613304507,1.,-1.81436959209778));
#29924=CARTESIAN_POINT('Ctrl Pts',(-1.22921864890975,1.,-1.81655087183054));
#29925=CARTESIAN_POINT('Ctrl Pts',(-1.23274224526804,1.,-1.81817389920914));
#29926=CARTESIAN_POINT('Ctrl Pts',(-1.23509651170384,1.,-1.81925017193531));
#29927=CARTESIAN_POINT('Ctrl Pts',(-1.23627494547115,1.,-1.81978687191668));
#29928=CARTESIAN_POINT('',(-0.892032620296856,0.,-1.5055822144029));
#29929=CARTESIAN_POINT('Origin',(0.,0.,0.));
#29930=CARTESIAN_POINT('',(-0.693717979106305,1.,-1.60662857109684));
#29931=CARTESIAN_POINT('Origin',(0.,1.,0.));
#29932=CARTESIAN_POINT('',(-0.693717979106306,0.,-1.60662857109684));
#29933=CARTESIAN_POINT('Ctrl Pts',(-0.745574324794401,-1.,-2.0698113262342));
#29934=CARTESIAN_POINT('Ctrl Pts',(-0.745574324794401,1.,-2.0698113262342));
#29935=CARTESIAN_POINT('Ctrl Pts',(-0.745832791378367,-1.,-2.06854248895728));
#29936=CARTESIAN_POINT('Ctrl Pts',(-0.745832791378367,1.,-2.06854248895728));
#29937=CARTESIAN_POINT('Ctrl Pts',(-0.7463458715442,-1.,-2.06600523016815));
#29938=CARTESIAN_POINT('Ctrl Pts',(-0.7463458715442,1.,-2.06600523016815));
#29939=CARTESIAN_POINT('Ctrl Pts',(-0.747103932787919,-1.,-2.06220058927826));
#29940=CARTESIAN_POINT('Ctrl Pts',(-0.747103932787919,1.,-2.06220058927826));
#29941=CARTESIAN_POINT('Ctrl Pts',(-0.748091554183802,-1.,-2.05713023031006));
#29942=CARTESIAN_POINT('Ctrl Pts',(-0.748091554183802,1.,-2.05713023031006));
#29943=CARTESIAN_POINT('Ctrl Pts',(-0.749287468665046,-1.,-2.05079645592154));
#29944=CARTESIAN_POINT('Ctrl Pts',(-0.749287468665046,1.,-2.05079645592154));
#29945=CARTESIAN_POINT('Ctrl Pts',(-0.750444657875576,-1.,-2.04446689147979));
#29946=CARTESIAN_POINT('Ctrl Pts',(-0.750444657875576,1.,-2.04446689147979));
#29947=CARTESIAN_POINT('Ctrl Pts',(-0.751562963361115,-1.,-2.03814160092099));
#29948=CARTESIAN_POINT('Ctrl Pts',(-0.751562963361115,1.,-2.03814160092099));
#29949=CARTESIAN_POINT('Ctrl Pts',(-0.752642180487211,-1.,-2.03182068456221));
#29950=CARTESIAN_POINT('Ctrl Pts',(-0.752642180487211,1.,-2.03182068456221));
#29951=CARTESIAN_POINT('Ctrl Pts',(-0.753682061112768,-1.,-2.02550428623313));
#29952=CARTESIAN_POINT('Ctrl Pts',(-0.753682061112768,1.,-2.02550428623313));
#29953=CARTESIAN_POINT('Ctrl Pts',(-0.754682330722816,-1.,-2.01919259405809));
#29954=CARTESIAN_POINT('Ctrl Pts',(-0.754682330722816,1.,-2.01919259405809));
#29955=CARTESIAN_POINT('Ctrl Pts',(-0.755642704957865,-1.,-2.01288584328084));
#29956=CARTESIAN_POINT('Ctrl Pts',(-0.755642704957865,1.,-2.01288584328084));
#29957=CARTESIAN_POINT('Ctrl Pts',(-0.75656290464667,-1.,-2.0065843158773));
#29958=CARTESIAN_POINT('Ctrl Pts',(-0.75656290464667,1.,-2.0065843158773));
#29959=CARTESIAN_POINT('Ctrl Pts',(-0.757442676862724,-1.,-2.00028834739178));
#29960=CARTESIAN_POINT('Ctrl Pts',(-0.757442676862724,1.,-2.00028834739178));
#29961=CARTESIAN_POINT('Ctrl Pts',(-0.758281796766761,-1.,-1.99399831098817));
#29962=CARTESIAN_POINT('Ctrl Pts',(-0.758281796766761,1.,-1.99399831098817));
#29963=CARTESIAN_POINT('Ctrl Pts',(-0.759080037802488,-1.,-1.98771456680874));
#29964=CARTESIAN_POINT('Ctrl Pts',(-0.759080037802488,1.,-1.98771456680874));
#29965=CARTESIAN_POINT('Ctrl Pts',(-0.75983714745219,-1.,-1.98143741418172));
#29966=CARTESIAN_POINT('Ctrl Pts',(-0.75983714745219,1.,-1.98143741418172));
#29967=CARTESIAN_POINT('Ctrl Pts',(-0.760552825409757,-1.,-1.97516705321494));
#29968=CARTESIAN_POINT('Ctrl Pts',(-0.760552825409757,1.,-1.97516705321494));
#29969=CARTESIAN_POINT('Ctrl Pts',(-0.76122669048382,-1.,-1.96890351582499));
#29970=CARTESIAN_POINT('Ctrl Pts',(-0.76122669048382,1.,-1.96890351582499));
#29971=CARTESIAN_POINT('Ctrl Pts',(-0.761858300014423,-1.,-1.96264672744186));
#29972=CARTESIAN_POINT('Ctrl Pts',(-0.761858300014423,1.,-1.96264672744186));
#29973=CARTESIAN_POINT('Ctrl Pts',(-0.762447203806179,-1.,-1.95639665309869));
#29974=CARTESIAN_POINT('Ctrl Pts',(-0.762447203806179,1.,-1.95639665309869));
#29975=CARTESIAN_POINT('Ctrl Pts',(-0.762992990878769,-1.,-1.95015342590024));
#29976=CARTESIAN_POINT('Ctrl Pts',(-0.762992990878769,1.,-1.95015342590024));
#29977=CARTESIAN_POINT('Ctrl Pts',(-0.763495333538629,-1.,-1.9439174661764));
#29978=CARTESIAN_POINT('Ctrl Pts',(-0.763495333538629,1.,-1.9439174661764));
#29979=CARTESIAN_POINT('Ctrl Pts',(-0.763954049121458,-1.,-1.93768964875886));
#29980=CARTESIAN_POINT('Ctrl Pts',(-0.763954049121458,1.,-1.93768964875886));
#29981=CARTESIAN_POINT('Ctrl Pts',(-0.764369010673941,-1.,-1.93147105496382));
#29982=CARTESIAN_POINT('Ctrl Pts',(-0.764369010673941,1.,-1.93147105496382));
#29983=CARTESIAN_POINT('Ctrl Pts',(-0.764740025488211,-1.,-1.92526263537048));
#29984=CARTESIAN_POINT('Ctrl Pts',(-0.764740025488211,1.,-1.92526263537048));
#29985=CARTESIAN_POINT('Ctrl Pts',(-0.765066729667088,-1.,-1.91906491634196));
#29986=CARTESIAN_POINT('Ctrl Pts',(-0.765066729667088,1.,-1.91906491634196));
#29987=CARTESIAN_POINT('Ctrl Pts',(-0.765348465884722,-1.,-1.91287765805169));
#29988=CARTESIAN_POINT('Ctrl Pts',(-0.765348465884722,1.,-1.91287765805169));
#29989=CARTESIAN_POINT('Ctrl Pts',(-0.765584196937919,-1.,-1.90669961402356));
#29990=CARTESIAN_POINT('Ctrl Pts',(-0.765584196937919,1.,-1.90669961402356));
#29991=CARTESIAN_POINT('Ctrl Pts',(-0.765772772593386,-1.,-1.90052930393596));
#29992=CARTESIAN_POINT('Ctrl Pts',(-0.765772772593386,1.,-1.90052930393596));
#29993=CARTESIAN_POINT('Ctrl Pts',(-0.765913193856978,-1.,-1.89436577771388));
#29994=CARTESIAN_POINT('Ctrl Pts',(-0.765913193856978,1.,-1.89436577771388));
#29995=CARTESIAN_POINT('Ctrl Pts',(-0.766004837062091,-1.,-1.88820926433409));
#29996=CARTESIAN_POINT('Ctrl Pts',(-0.766004837062091,1.,-1.88820926433409));
#29997=CARTESIAN_POINT('Ctrl Pts',(-0.766047794851865,-1.,-1.88206215302561));
#29998=CARTESIAN_POINT('Ctrl Pts',(-0.766047794851865,1.,-1.88206215302561));
#29999=CARTESIAN_POINT('Ctrl Pts',(-0.766042837036744,-1.,-1.87592888967883));
#30000=CARTESIAN_POINT('Ctrl Pts',(-0.766042837036744,1.,-1.87592888967883));
#30001=CARTESIAN_POINT('Ctrl Pts',(-0.765990708546091,-1.,-1.86981398314341));
#30002=CARTESIAN_POINT('Ctrl Pts',(-0.765990708546091,1.,-1.86981398314341));
#30003=CARTESIAN_POINT('Ctrl Pts',(-0.765891519092547,-1.,-1.86372027063312));
#30004=CARTESIAN_POINT('Ctrl Pts',(-0.765891519092547,1.,-1.86372027063312));
#30005=CARTESIAN_POINT('Ctrl Pts',(-0.765744212909318,-1.,-1.85764741390394));
#30006=CARTESIAN_POINT('Ctrl Pts',(-0.765744212909318,1.,-1.85764741390394));
#30007=CARTESIAN_POINT('Ctrl Pts',(-0.765545710619062,-1.,-1.85158945130063));
#30008=CARTESIAN_POINT('Ctrl Pts',(-0.765545710619062,1.,-1.85158945130063));
#30009=CARTESIAN_POINT('Ctrl Pts',(-0.765291664862029,-1.,-1.84553698875924));
#30010=CARTESIAN_POINT('Ctrl Pts',(-0.765291664862029,1.,-1.84553698875924));
#30011=CARTESIAN_POINT('Ctrl Pts',(-0.764978057881737,-1.,-1.83948181064835));
#30012=CARTESIAN_POINT('Ctrl Pts',(-0.764978057881737,1.,-1.83948181064835));
#30013=CARTESIAN_POINT('Ctrl Pts',(-0.764602549687853,-1.,-1.83342077227142));
#30014=CARTESIAN_POINT('Ctrl Pts',(-0.764602549687853,1.,-1.83342077227142));
#30015=CARTESIAN_POINT('Ctrl Pts',(-0.764165902605995,-1.,-1.82735991200065));
#30016=CARTESIAN_POINT('Ctrl Pts',(-0.764165902605995,1.,-1.82735991200065));
#30017=CARTESIAN_POINT('Ctrl Pts',(-0.763673465462726,-1.,-1.82131873145266));
#30018=CARTESIAN_POINT('Ctrl Pts',(-0.763673465462726,1.,-1.82131873145266));
#30019=CARTESIAN_POINT('Ctrl Pts',(-0.763132003836634,-1.,-1.8153211840553));
#30020=CARTESIAN_POINT('Ctrl Pts',(-0.763132003836634,1.,-1.8153211840553));
#30021=CARTESIAN_POINT('Ctrl Pts',(-0.762546129463938,-1.,-1.80938551463965));
#30022=CARTESIAN_POINT('Ctrl Pts',(-0.762546129463938,1.,-1.80938551463965));
#30023=CARTESIAN_POINT('Ctrl Pts',(-0.761915336443547,-1.,-1.80351583877342));
#30024=CARTESIAN_POINT('Ctrl Pts',(-0.761915336443547,1.,-1.80351583877342));
#30025=CARTESIAN_POINT('Ctrl Pts',(-0.761229695230558,-1.,-1.79768986997783));
#30026=CARTESIAN_POINT('Ctrl Pts',(-0.761229695230558,1.,-1.79768986997783));
#30027=CARTESIAN_POINT('Ctrl Pts',(-0.760469555880749,-1.,-1.7918581561088));
#30028=CARTESIAN_POINT('Ctrl Pts',(-0.760469555880749,1.,-1.7918581561088));
#30029=CARTESIAN_POINT('Ctrl Pts',(-0.759614401110189,-1.,-1.78596964884604));
#30030=CARTESIAN_POINT('Ctrl Pts',(-0.759614401110189,1.,-1.78596964884604));
#30031=CARTESIAN_POINT('Ctrl Pts',(-0.758650626677518,-1.,-1.77999411220945));
#30032=CARTESIAN_POINT('Ctrl Pts',(-0.758650626677518,1.,-1.77999411220945));
#30033=CARTESIAN_POINT('Ctrl Pts',(-0.757578264077029,-1.,-1.77394167108292));
#30034=CARTESIAN_POINT('Ctrl Pts',(-0.757578264077029,1.,-1.77394167108292));
#30035=CARTESIAN_POINT('Ctrl Pts',(-0.75642189602781,-1.,-1.76789396002998));
#30036=CARTESIAN_POINT('Ctrl Pts',(-0.75642189602781,1.,-1.76789396002998));
#30037=CARTESIAN_POINT('Ctrl Pts',(-0.755220979974461,-1.,-1.76197817240128));
#30038=CARTESIAN_POINT('Ctrl Pts',(-0.755220979974461,1.,-1.76197817240128));
#30039=CARTESIAN_POINT('Ctrl Pts',(-0.754009254027829,-1.,-1.75631083600019));
#30040=CARTESIAN_POINT('Ctrl Pts',(-0.754009254027829,1.,-1.75631083600019));
#30041=CARTESIAN_POINT('Ctrl Pts',(-0.752797683531314,-1.,-1.75095139468794));
#30042=CARTESIAN_POINT('Ctrl Pts',(-0.752797683531314,1.,-1.75095139468794));
#30043=CARTESIAN_POINT('Ctrl Pts',(-0.751555614164482,-1.,-1.74585086852502));
#30044=CARTESIAN_POINT('Ctrl Pts',(-0.751555614164482,1.,-1.74585086852502));
#30045=CARTESIAN_POINT('Ctrl Pts',(-0.750193435981249,-1.,-1.74080458267114));
#30046=CARTESIAN_POINT('Ctrl Pts',(-0.750193435981249,1.,-1.74080458267114));
#30047=CARTESIAN_POINT('Ctrl Pts',(-0.74858246295687,-1.,-1.7355035168033));
#30048=CARTESIAN_POINT('Ctrl Pts',(-0.74858246295687,1.,-1.7355035168033));
#30049=CARTESIAN_POINT('Ctrl Pts',(-0.746574710097752,-1.,-1.72958533647714));
#30050=CARTESIAN_POINT('Ctrl Pts',(-0.746574710097752,1.,-1.72958533647714));
#30051=CARTESIAN_POINT('Ctrl Pts',(-0.744021445433093,-1.,-1.72268229916769));
#30052=CARTESIAN_POINT('Ctrl Pts',(-0.744021445433093,1.,-1.72268229916769));
#30053=CARTESIAN_POINT('Ctrl Pts',(-0.74079516202821,-1.,-1.71447789751001));
#30054=CARTESIAN_POINT('Ctrl Pts',(-0.74079516202821,1.,-1.71447789751001));
#30055=CARTESIAN_POINT('Ctrl Pts',(-0.736799665716932,-1.,-1.70473309004249));
#30056=CARTESIAN_POINT('Ctrl Pts',(-0.736799665716932,1.,-1.70473309004249));
#30057=CARTESIAN_POINT('Ctrl Pts',(-0.731963238685357,-1.,-1.69326921972915));
#30058=CARTESIAN_POINT('Ctrl Pts',(-0.731963238685357,1.,-1.69326921972915));
#30059=CARTESIAN_POINT('Ctrl Pts',(-0.726235967982445,-1.,-1.67996158451922));
#30060=CARTESIAN_POINT('Ctrl Pts',(-0.726235967982445,1.,-1.67996158451922));
#30061=CARTESIAN_POINT('Ctrl Pts',(-0.71958543378795,-1.,-1.66472880551777));
#30062=CARTESIAN_POINT('Ctrl Pts',(-0.71958543378795,1.,-1.66472880551777));
#30063=CARTESIAN_POINT('Ctrl Pts',(-0.711993139340447,-1.,-1.64752408828442));
#30064=CARTESIAN_POINT('Ctrl Pts',(-0.711993139340447,1.,-1.64752408828442));
#30065=CARTESIAN_POINT('Ctrl Pts',(-0.705159151977294,-1.,-1.6321654166204));
#30066=CARTESIAN_POINT('Ctrl Pts',(-0.705159151977294,1.,-1.6321654166204));
#30067=CARTESIAN_POINT('Ctrl Pts',(-0.699605146398837,-1.,-1.61974673471117));
#30068=CARTESIAN_POINT('Ctrl Pts',(-0.699605146398837,1.,-1.61974673471117));
#30069=CARTESIAN_POINT('Ctrl Pts',(-0.69571209787897,-1.,-1.61106790957619));
#30070=CARTESIAN_POINT('Ctrl Pts',(-0.69571209787897,1.,-1.61106790957619));
#30071=CARTESIAN_POINT('Ctrl Pts',(-0.693717979106305,-1.,-1.60662857109684));
#30072=CARTESIAN_POINT('Ctrl Pts',(-0.693717979106305,1.,-1.60662857109684));
#30073=CARTESIAN_POINT('',(-0.745574324794401,1.,-2.0698113262342));
#30074=CARTESIAN_POINT('Ctrl Pts',(-0.745574324794401,1.,-2.0698113262342));
#30075=CARTESIAN_POINT('Ctrl Pts',(-0.745832791378367,1.,-2.06854248895728));
#30076=CARTESIAN_POINT('Ctrl Pts',(-0.7463458715442,1.,-2.06600523016815));
#30077=CARTESIAN_POINT('Ctrl Pts',(-0.747103932787919,1.,-2.06220058927826));
#30078=CARTESIAN_POINT('Ctrl Pts',(-0.748091554183802,1.,-2.05713023031006));
#30079=CARTESIAN_POINT('Ctrl Pts',(-0.749287468665046,1.,-2.05079645592154));
#30080=CARTESIAN_POINT('Ctrl Pts',(-0.750444657875576,1.,-2.04446689147979));
#30081=CARTESIAN_POINT('Ctrl Pts',(-0.751562963361115,1.,-2.03814160092099));
#30082=CARTESIAN_POINT('Ctrl Pts',(-0.752642180487211,1.,-2.03182068456221));
#30083=CARTESIAN_POINT('Ctrl Pts',(-0.753682061112768,1.,-2.02550428623313));
#30084=CARTESIAN_POINT('Ctrl Pts',(-0.754682330722816,1.,-2.01919259405809));
#30085=CARTESIAN_POINT('Ctrl Pts',(-0.755642704957865,1.,-2.01288584328084));
#30086=CARTESIAN_POINT('Ctrl Pts',(-0.75656290464667,1.,-2.0065843158773));
#30087=CARTESIAN_POINT('Ctrl Pts',(-0.757442676862724,1.,-2.00028834739178));
#30088=CARTESIAN_POINT('Ctrl Pts',(-0.758281796766761,1.,-1.99399831098817));
#30089=CARTESIAN_POINT('Ctrl Pts',(-0.759080037802488,1.,-1.98771456680874));
#30090=CARTESIAN_POINT('Ctrl Pts',(-0.75983714745219,1.,-1.98143741418172));
#30091=CARTESIAN_POINT('Ctrl Pts',(-0.760552825409757,1.,-1.97516705321494));
#30092=CARTESIAN_POINT('Ctrl Pts',(-0.76122669048382,1.,-1.96890351582499));
#30093=CARTESIAN_POINT('Ctrl Pts',(-0.761858300014423,1.,-1.96264672744186));
#30094=CARTESIAN_POINT('Ctrl Pts',(-0.762447203806179,1.,-1.95639665309869));
#30095=CARTESIAN_POINT('Ctrl Pts',(-0.762992990878769,1.,-1.95015342590024));
#30096=CARTESIAN_POINT('Ctrl Pts',(-0.763495333538629,1.,-1.9439174661764));
#30097=CARTESIAN_POINT('Ctrl Pts',(-0.763954049121458,1.,-1.93768964875886));
#30098=CARTESIAN_POINT('Ctrl Pts',(-0.764369010673941,1.,-1.93147105496382));
#30099=CARTESIAN_POINT('Ctrl Pts',(-0.764740025488211,1.,-1.92526263537048));
#30100=CARTESIAN_POINT('Ctrl Pts',(-0.765066729667088,1.,-1.91906491634196));
#30101=CARTESIAN_POINT('Ctrl Pts',(-0.765348465884722,1.,-1.91287765805169));
#30102=CARTESIAN_POINT('Ctrl Pts',(-0.765584196937919,1.,-1.90669961402356));
#30103=CARTESIAN_POINT('Ctrl Pts',(-0.765772772593386,1.,-1.90052930393596));
#30104=CARTESIAN_POINT('Ctrl Pts',(-0.765913193856978,1.,-1.89436577771388));
#30105=CARTESIAN_POINT('Ctrl Pts',(-0.766004837062091,1.,-1.88820926433409));
#30106=CARTESIAN_POINT('Ctrl Pts',(-0.766047794851865,1.,-1.88206215302561));
#30107=CARTESIAN_POINT('Ctrl Pts',(-0.766042837036744,1.,-1.87592888967883));
#30108=CARTESIAN_POINT('Ctrl Pts',(-0.765990708546091,1.,-1.86981398314341));
#30109=CARTESIAN_POINT('Ctrl Pts',(-0.765891519092547,1.,-1.86372027063312));
#30110=CARTESIAN_POINT('Ctrl Pts',(-0.765744212909318,1.,-1.85764741390394));
#30111=CARTESIAN_POINT('Ctrl Pts',(-0.765545710619062,1.,-1.85158945130063));
#30112=CARTESIAN_POINT('Ctrl Pts',(-0.765291664862029,1.,-1.84553698875924));
#30113=CARTESIAN_POINT('Ctrl Pts',(-0.764978057881737,1.,-1.83948181064835));
#30114=CARTESIAN_POINT('Ctrl Pts',(-0.764602549687853,1.,-1.83342077227142));
#30115=CARTESIAN_POINT('Ctrl Pts',(-0.764165902605995,1.,-1.82735991200065));
#30116=CARTESIAN_POINT('Ctrl Pts',(-0.763673465462726,1.,-1.82131873145266));
#30117=CARTESIAN_POINT('Ctrl Pts',(-0.763132003836634,1.,-1.8153211840553));
#30118=CARTESIAN_POINT('Ctrl Pts',(-0.762546129463938,1.,-1.80938551463965));
#30119=CARTESIAN_POINT('Ctrl Pts',(-0.761915336443547,1.,-1.80351583877342));
#30120=CARTESIAN_POINT('Ctrl Pts',(-0.761229695230558,1.,-1.79768986997783));
#30121=CARTESIAN_POINT('Ctrl Pts',(-0.760469555880749,1.,-1.7918581561088));
#30122=CARTESIAN_POINT('Ctrl Pts',(-0.759614401110189,1.,-1.78596964884604));
#30123=CARTESIAN_POINT('Ctrl Pts',(-0.758650626677518,1.,-1.77999411220945));
#30124=CARTESIAN_POINT('Ctrl Pts',(-0.757578264077029,1.,-1.77394167108292));
#30125=CARTESIAN_POINT('Ctrl Pts',(-0.75642189602781,1.,-1.76789396002998));
#30126=CARTESIAN_POINT('Ctrl Pts',(-0.755220979974461,1.,-1.76197817240128));
#30127=CARTESIAN_POINT('Ctrl Pts',(-0.754009254027829,1.,-1.75631083600019));
#30128=CARTESIAN_POINT('Ctrl Pts',(-0.752797683531314,1.,-1.75095139468794));
#30129=CARTESIAN_POINT('Ctrl Pts',(-0.751555614164482,1.,-1.74585086852502));
#30130=CARTESIAN_POINT('Ctrl Pts',(-0.750193435981249,1.,-1.74080458267114));
#30131=CARTESIAN_POINT('Ctrl Pts',(-0.74858246295687,1.,-1.7355035168033));
#30132=CARTESIAN_POINT('Ctrl Pts',(-0.746574710097752,1.,-1.72958533647714));
#30133=CARTESIAN_POINT('Ctrl Pts',(-0.744021445433093,1.,-1.72268229916769));
#30134=CARTESIAN_POINT('Ctrl Pts',(-0.74079516202821,1.,-1.71447789751001));
#30135=CARTESIAN_POINT('Ctrl Pts',(-0.736799665716932,1.,-1.70473309004249));
#30136=CARTESIAN_POINT('Ctrl Pts',(-0.731963238685357,1.,-1.69326921972915));
#30137=CARTESIAN_POINT('Ctrl Pts',(-0.726235967982445,1.,-1.67996158451922));
#30138=CARTESIAN_POINT('Ctrl Pts',(-0.71958543378795,1.,-1.66472880551777));
#30139=CARTESIAN_POINT('Ctrl Pts',(-0.711993139340447,1.,-1.64752408828442));
#30140=CARTESIAN_POINT('Ctrl Pts',(-0.705159151977294,1.,-1.6321654166204));
#30141=CARTESIAN_POINT('Ctrl Pts',(-0.699605146398837,1.,-1.61974673471117));
#30142=CARTESIAN_POINT('Ctrl Pts',(-0.69571209787897,1.,-1.61106790957619));
#30143=CARTESIAN_POINT('Ctrl Pts',(-0.693717979106305,1.,-1.60662857109684));
#30144=CARTESIAN_POINT('',(-0.745574324794401,0.,-2.0698113262342));
#30145=CARTESIAN_POINT('Origin',(-0.61342227326009,0.,-2.11275013067528));
#30146=CARTESIAN_POINT('',(-0.61342227326009,1.,-2.11275013067528));
#30147=CARTESIAN_POINT('',(-0.745574324794401,1.,-2.0698113262342));
#30148=CARTESIAN_POINT('',(-0.61342227326009,0.,-2.11275013067528));
#30149=CARTESIAN_POINT('Ctrl Pts',(-0.383122945602004,-1.,-1.7075470150345));
#30150=CARTESIAN_POINT('Ctrl Pts',(-0.383122945602004,1.,-1.7075470150345));
#30151=CARTESIAN_POINT('Ctrl Pts',(-0.384119047315542,-1.,-1.71231062891958));
#30152=CARTESIAN_POINT('Ctrl Pts',(-0.384119047315542,1.,-1.71231062891958));
#30153=CARTESIAN_POINT('Ctrl Pts',(-0.38607079032701,-1.,-1.72162022246158));
#30154=CARTESIAN_POINT('Ctrl Pts',(-0.38607079032701,1.,-1.72162022246158));
#30155=CARTESIAN_POINT('Ctrl Pts',(-0.388877023509191,-1.,-1.7349317097561));
#30156=CARTESIAN_POINT('Ctrl Pts',(-0.388877023509191,1.,-1.7349317097561));
#30157=CARTESIAN_POINT('Ctrl Pts',(-0.392375812294307,-1.,-1.75137405313962));
#30158=CARTESIAN_POINT('Ctrl Pts',(-0.392375812294307,1.,-1.75137405313962));
#30159=CARTESIAN_POINT('Ctrl Pts',(-0.39634619612042,-1.,-1.7697556004756));
#30160=CARTESIAN_POINT('Ctrl Pts',(-0.39634619612042,1.,-1.7697556004756));
#30161=CARTESIAN_POINT('Ctrl Pts',(-0.39991940378308,-1.,-1.78598826347533));
#30162=CARTESIAN_POINT('Ctrl Pts',(-0.39991940378308,1.,-1.78598826347533));
#30163=CARTESIAN_POINT('Ctrl Pts',(-0.403107976170441,-1.,-1.80012077176221));
#30164=CARTESIAN_POINT('Ctrl Pts',(-0.403107976170441,1.,-1.80012077176221));
#30165=CARTESIAN_POINT('Ctrl Pts',(-0.405933518411838,-1.,-1.81223801813988));
#30166=CARTESIAN_POINT('Ctrl Pts',(-0.405933518411838,1.,-1.81223801813988));
#30167=CARTESIAN_POINT('Ctrl Pts',(-0.408428948108533,-1.,-1.8224702267854));
#30168=CARTESIAN_POINT('Ctrl Pts',(-0.408428948108533,1.,-1.8224702267854));
#30169=CARTESIAN_POINT('Ctrl Pts',(-0.410641256301675,-1.,-1.83100408895216));
#30170=CARTESIAN_POINT('Ctrl Pts',(-0.410641256301675,1.,-1.83100408895216));
#30171=CARTESIAN_POINT('Ctrl Pts',(-0.412633125322162,-1.,-1.83808953475839));
#30172=CARTESIAN_POINT('Ctrl Pts',(-0.412633125322162,1.,-1.83808953475839));
#30173=CARTESIAN_POINT('Ctrl Pts',(-0.41448743825434,-1.,-1.8440575707371));
#30174=CARTESIAN_POINT('Ctrl Pts',(-0.41448743825434,1.,-1.8440575707371));
#30175=CARTESIAN_POINT('Ctrl Pts',(-0.416300022038864,-1.,-1.84929312929882));
#30176=CARTESIAN_POINT('Ctrl Pts',(-0.416300022038864,1.,-1.84929312929882));
#30177=CARTESIAN_POINT('Ctrl Pts',(-0.418164129143534,-1.,-1.85417632856234));
#30178=CARTESIAN_POINT('Ctrl Pts',(-0.418164129143534,1.,-1.85417632856234));
#30179=CARTESIAN_POINT('Ctrl Pts',(-0.420157287975619,-1.,-1.85903281096686));
#30180=CARTESIAN_POINT('Ctrl Pts',(-0.420157287975619,1.,-1.85903281096686));
#30181=CARTESIAN_POINT('Ctrl Pts',(-0.422327307418275,-1.,-1.86408083334028));
#30182=CARTESIAN_POINT('Ctrl Pts',(-0.422327307418275,1.,-1.86408083334028));
#30183=CARTESIAN_POINT('Ctrl Pts',(-0.424678177291359,-1.,-1.86937803944323));
#30184=CARTESIAN_POINT('Ctrl Pts',(-0.424678177291359,1.,-1.86937803944323));
#30185=CARTESIAN_POINT('Ctrl Pts',(-0.427183828519102,-1.,-1.87486989291484));
#30186=CARTESIAN_POINT('Ctrl Pts',(-0.427183828519102,1.,-1.87486989291484));
#30187=CARTESIAN_POINT('Ctrl Pts',(-0.429803062482344,-1.,-1.88044229001832));
#30188=CARTESIAN_POINT('Ctrl Pts',(-0.429803062482344,1.,-1.88044229001832));
#30189=CARTESIAN_POINT('Ctrl Pts',(-0.432493038548748,-1.,-1.88596913666793));
#30190=CARTESIAN_POINT('Ctrl Pts',(-0.432493038548748,1.,-1.88596913666793));
#30191=CARTESIAN_POINT('Ctrl Pts',(-0.435225660963383,-1.,-1.89136993975504));
#30192=CARTESIAN_POINT('Ctrl Pts',(-0.435225660963383,1.,-1.89136993975504));
#30193=CARTESIAN_POINT('Ctrl Pts',(-0.437995003948244,-1.,-1.89663648956466));
#30194=CARTESIAN_POINT('Ctrl Pts',(-0.437995003948244,1.,-1.89663648956466));
#30195=CARTESIAN_POINT('Ctrl Pts',(-0.440807833704038,-1.,-1.90180124389086));
#30196=CARTESIAN_POINT('Ctrl Pts',(-0.440807833704038,1.,-1.90180124389086));
#30197=CARTESIAN_POINT('Ctrl Pts',(-0.443677556849151,-1.,-1.90691756144898));
#30198=CARTESIAN_POINT('Ctrl Pts',(-0.443677556849151,1.,-1.90691756144898));
#30199=CARTESIAN_POINT('Ctrl Pts',(-0.446617343485711,-1.,-1.9120369998112));
#30200=CARTESIAN_POINT('Ctrl Pts',(-0.446617343485711,1.,-1.9120369998112));
#30201=CARTESIAN_POINT('Ctrl Pts',(-0.449632260106662,-1.,-1.91718342555755));
#30202=CARTESIAN_POINT('Ctrl Pts',(-0.449632260106662,1.,-1.91718342555755));
#30203=CARTESIAN_POINT('Ctrl Pts',(-0.452719478359432,-1.,-1.92235380648502));
#30204=CARTESIAN_POINT('Ctrl Pts',(-0.452719478359432,1.,-1.92235380648502));
#30205=CARTESIAN_POINT('Ctrl Pts',(-0.455872005174371,-1.,-1.92753067150476));
#30206=CARTESIAN_POINT('Ctrl Pts',(-0.455872005174371,1.,-1.92753067150476));
#30207=CARTESIAN_POINT('Ctrl Pts',(-0.459081234547926,-1.,-1.93269066517934));
#30208=CARTESIAN_POINT('Ctrl Pts',(-0.459081234547926,1.,-1.93269066517934));
#30209=CARTESIAN_POINT('Ctrl Pts',(-0.462340031009056,-1.,-1.93781486640821));
#30210=CARTESIAN_POINT('Ctrl Pts',(-0.462340031009056,1.,-1.93781486640821));
#30211=CARTESIAN_POINT('Ctrl Pts',(-0.46564546202603,-1.,-1.9428979419619));
#30212=CARTESIAN_POINT('Ctrl Pts',(-0.46564546202603,1.,-1.9428979419619));
#30213=CARTESIAN_POINT('Ctrl Pts',(-0.468997482913135,-1.,-1.94794381136514));
#30214=CARTESIAN_POINT('Ctrl Pts',(-0.468997482913135,1.,-1.94794381136514));
#30215=CARTESIAN_POINT('Ctrl Pts',(-0.472397672264072,-1.,-1.95296148278133));
#30216=CARTESIAN_POINT('Ctrl Pts',(-0.472397672264072,1.,-1.95296148278133));
#30217=CARTESIAN_POINT('Ctrl Pts',(-0.475848034683176,-1.,-1.95796111148177));
#30218=CARTESIAN_POINT('Ctrl Pts',(-0.475848034683176,1.,-1.95796111148177));
#30219=CARTESIAN_POINT('Ctrl Pts',(-0.479349583074855,-1.,-1.96294933055943));
#30220=CARTESIAN_POINT('Ctrl Pts',(-0.479349583074855,1.,-1.96294933055943));
#30221=CARTESIAN_POINT('Ctrl Pts',(-0.482901662120691,-1.,-1.96792703422362));
#30222=CARTESIAN_POINT('Ctrl Pts',(-0.482901662120691,1.,-1.96792703422362));
#30223=CARTESIAN_POINT('Ctrl Pts',(-0.486502692907659,-1.,-1.97289186263272));
#30224=CARTESIAN_POINT('Ctrl Pts',(-0.486502692907659,1.,-1.97289186263272));
#30225=CARTESIAN_POINT('Ctrl Pts',(-0.490150627860952,-1.,-1.97783973019229));
#30226=CARTESIAN_POINT('Ctrl Pts',(-0.490150627860952,1.,-1.97783973019229));
#30227=CARTESIAN_POINT('Ctrl Pts',(-0.493843476541495,-1.,-1.98276658761821));
#30228=CARTESIAN_POINT('Ctrl Pts',(-0.493843476541495,1.,-1.98276658761821));
#30229=CARTESIAN_POINT('Ctrl Pts',(-0.497579909545574,-1.,-1.98767044752932));
#30230=CARTESIAN_POINT('Ctrl Pts',(-0.497579909545574,1.,-1.98767044752932));
#30231=CARTESIAN_POINT('Ctrl Pts',(-0.501359287727146,-1.,-1.99255149126155));
#30232=CARTESIAN_POINT('Ctrl Pts',(-0.501359287727146,1.,-1.99255149126155));
#30233=CARTESIAN_POINT('Ctrl Pts',(-0.505181361323026,-1.,-1.99741107463572));
#30234=CARTESIAN_POINT('Ctrl Pts',(-0.505181361323026,1.,-1.99741107463572));
#30235=CARTESIAN_POINT('Ctrl Pts',(-0.509046069886157,-1.,-2.00225107134734));
#30236=CARTESIAN_POINT('Ctrl Pts',(-0.509046069886157,1.,-2.00225107134734));
#30237=CARTESIAN_POINT('Ctrl Pts',(-0.512953306961792,-1.,-2.00707309946949));
#30238=CARTESIAN_POINT('Ctrl Pts',(-0.512953306961792,1.,-2.00707309946949));
#30239=CARTESIAN_POINT('Ctrl Pts',(-0.516902681728687,-1.,-2.01187773939242));
#30240=CARTESIAN_POINT('Ctrl Pts',(-0.516902681728687,1.,-2.01187773939242));
#30241=CARTESIAN_POINT('Ctrl Pts',(-0.52089359039937,-1.,-2.01666477917286));
#30242=CARTESIAN_POINT('Ctrl Pts',(-0.52089359039937,1.,-2.01666477917286));
#30243=CARTESIAN_POINT('Ctrl Pts',(-0.524925318333476,-1.,-2.02143356304698));
#30244=CARTESIAN_POINT('Ctrl Pts',(-0.524925318333476,1.,-2.02143356304698));
#30245=CARTESIAN_POINT('Ctrl Pts',(-0.528997127241914,-1.,-2.0261832908329));
#30246=CARTESIAN_POINT('Ctrl Pts',(-0.528997127241914,1.,-2.0261832908329));
#30247=CARTESIAN_POINT('Ctrl Pts',(-0.533108355132977,-1.,-2.03091336214426));
#30248=CARTESIAN_POINT('Ctrl Pts',(-0.533108355132977,1.,-2.03091336214426));
#30249=CARTESIAN_POINT('Ctrl Pts',(-0.537258489833262,-1.,-2.03562362954037));
#30250=CARTESIAN_POINT('Ctrl Pts',(-0.537258489833262,1.,-2.03562362954037));
#30251=CARTESIAN_POINT('Ctrl Pts',(-0.541447120615659,-1.,-2.04031422690527));
#30252=CARTESIAN_POINT('Ctrl Pts',(-0.541447120615659,1.,-2.04031422690527));
#30253=CARTESIAN_POINT('Ctrl Pts',(-0.54567390381743,-1.,-2.04498544714588));
#30254=CARTESIAN_POINT('Ctrl Pts',(-0.54567390381743,1.,-2.04498544714588));
#30255=CARTESIAN_POINT('Ctrl Pts',(-0.549938525150295,-1.,-2.04963761077958));
#30256=CARTESIAN_POINT('Ctrl Pts',(-0.549938525150295,1.,-2.04963761077958));
#30257=CARTESIAN_POINT('Ctrl Pts',(-0.554240657463906,-1.,-2.05427091604413));
#30258=CARTESIAN_POINT('Ctrl Pts',(-0.554240657463906,1.,-2.05427091604413));
#30259=CARTESIAN_POINT('Ctrl Pts',(-0.558579940185151,-1.,-2.05888537756462));
#30260=CARTESIAN_POINT('Ctrl Pts',(-0.558579940185151,1.,-2.05888537756462));
#30261=CARTESIAN_POINT('Ctrl Pts',(-0.562955993082261,-1.,-2.06348090160589));
#30262=CARTESIAN_POINT('Ctrl Pts',(-0.562955993082261,1.,-2.06348090160589));
#30263=CARTESIAN_POINT('Ctrl Pts',(-0.567368421181087,-1.,-2.06805732997334));
#30264=CARTESIAN_POINT('Ctrl Pts',(-0.567368421181087,1.,-2.06805732997334));
#30265=CARTESIAN_POINT('Ctrl Pts',(-0.571816823242603,-1.,-2.07261449292824));
#30266=CARTESIAN_POINT('Ctrl Pts',(-0.571816823242603,1.,-2.07261449292824));
#30267=CARTESIAN_POINT('Ctrl Pts',(-0.576300797416844,-1.,-2.07715226767559));
#30268=CARTESIAN_POINT('Ctrl Pts',(-0.576300797416844,1.,-2.07715226767559));
#30269=CARTESIAN_POINT('Ctrl Pts',(-0.580819952108063,-1.,-2.08167059018418));
#30270=CARTESIAN_POINT('Ctrl Pts',(-0.580819952108063,1.,-2.08167059018418));
#30271=CARTESIAN_POINT('Ctrl Pts',(-0.585373918991617,-1.,-2.08616943727951));
#30272=CARTESIAN_POINT('Ctrl Pts',(-0.585373918991617,1.,-2.08616943727951));
#30273=CARTESIAN_POINT('Ctrl Pts',(-0.589962365403406,-1.,-2.09064881812129));
#30274=CARTESIAN_POINT('Ctrl Pts',(-0.589962365403406,1.,-2.09064881812129));
#30275=CARTESIAN_POINT('Ctrl Pts',(-0.594585006052162,-1.,-2.0951087622027));
#30276=CARTESIAN_POINT('Ctrl Pts',(-0.594585006052162,1.,-2.0951087622027));
#30277=CARTESIAN_POINT('Ctrl Pts',(-0.599241616420533,-1.,-2.0995493086477));
#30278=CARTESIAN_POINT('Ctrl Pts',(-0.599241616420533,1.,-2.0995493086477));
#30279=CARTESIAN_POINT('Ctrl Pts',(-0.60393203073603,-1.,-2.10397049886949));
#30280=CARTESIAN_POINT('Ctrl Pts',(-0.60393203073603,1.,-2.10397049886949));
#30281=CARTESIAN_POINT('Ctrl Pts',(-0.607711315454876,-1.,-2.1074919961518));
#30282=CARTESIAN_POINT('Ctrl Pts',(-0.607711315454876,1.,-2.1074919961518));
#30283=CARTESIAN_POINT('Ctrl Pts',(-0.610560911689899,-1.,-2.11012443807238));
#30284=CARTESIAN_POINT('Ctrl Pts',(-0.610560911689899,1.,-2.11012443807238));
#30285=CARTESIAN_POINT('Ctrl Pts',(-0.6124673655618,-1.,-2.11187554259986));
#30286=CARTESIAN_POINT('Ctrl Pts',(-0.6124673655618,1.,-2.11187554259986));
#30287=CARTESIAN_POINT('Ctrl Pts',(-0.61342227326009,-1.,-2.11275013067528));
#30288=CARTESIAN_POINT('Ctrl Pts',(-0.61342227326009,1.,-2.11275013067528));
#30289=CARTESIAN_POINT('',(-0.383122945602004,1.,-1.7075470150345));
#30290=CARTESIAN_POINT('Ctrl Pts',(-0.383122945602004,1.,-1.7075470150345));
#30291=CARTESIAN_POINT('Ctrl Pts',(-0.384119047315542,1.,-1.71231062891958));
#30292=CARTESIAN_POINT('Ctrl Pts',(-0.38607079032701,1.,-1.72162022246158));
#30293=CARTESIAN_POINT('Ctrl Pts',(-0.388877023509191,1.,-1.7349317097561));
#30294=CARTESIAN_POINT('Ctrl Pts',(-0.392375812294307,1.,-1.75137405313962));
#30295=CARTESIAN_POINT('Ctrl Pts',(-0.39634619612042,1.,-1.7697556004756));
#30296=CARTESIAN_POINT('Ctrl Pts',(-0.39991940378308,1.,-1.78598826347533));
#30297=CARTESIAN_POINT('Ctrl Pts',(-0.403107976170441,1.,-1.80012077176221));
#30298=CARTESIAN_POINT('Ctrl Pts',(-0.405933518411838,1.,-1.81223801813988));
#30299=CARTESIAN_POINT('Ctrl Pts',(-0.408428948108533,1.,-1.8224702267854));
#30300=CARTESIAN_POINT('Ctrl Pts',(-0.410641256301675,1.,-1.83100408895216));
#30301=CARTESIAN_POINT('Ctrl Pts',(-0.412633125322162,1.,-1.83808953475839));
#30302=CARTESIAN_POINT('Ctrl Pts',(-0.41448743825434,1.,-1.8440575707371));
#30303=CARTESIAN_POINT('Ctrl Pts',(-0.416300022038864,1.,-1.84929312929882));
#30304=CARTESIAN_POINT('Ctrl Pts',(-0.418164129143534,1.,-1.85417632856234));
#30305=CARTESIAN_POINT('Ctrl Pts',(-0.420157287975619,1.,-1.85903281096686));
#30306=CARTESIAN_POINT('Ctrl Pts',(-0.422327307418275,1.,-1.86408083334028));
#30307=CARTESIAN_POINT('Ctrl Pts',(-0.424678177291359,1.,-1.86937803944323));
#30308=CARTESIAN_POINT('Ctrl Pts',(-0.427183828519102,1.,-1.87486989291484));
#30309=CARTESIAN_POINT('Ctrl Pts',(-0.429803062482344,1.,-1.88044229001832));
#30310=CARTESIAN_POINT('Ctrl Pts',(-0.432493038548748,1.,-1.88596913666793));
#30311=CARTESIAN_POINT('Ctrl Pts',(-0.435225660963383,1.,-1.89136993975504));
#30312=CARTESIAN_POINT('Ctrl Pts',(-0.437995003948244,1.,-1.89663648956466));
#30313=CARTESIAN_POINT('Ctrl Pts',(-0.440807833704038,1.,-1.90180124389086));
#30314=CARTESIAN_POINT('Ctrl Pts',(-0.443677556849151,1.,-1.90691756144898));
#30315=CARTESIAN_POINT('Ctrl Pts',(-0.446617343485711,1.,-1.9120369998112));
#30316=CARTESIAN_POINT('Ctrl Pts',(-0.449632260106662,1.,-1.91718342555755));
#30317=CARTESIAN_POINT('Ctrl Pts',(-0.452719478359432,1.,-1.92235380648502));
#30318=CARTESIAN_POINT('Ctrl Pts',(-0.455872005174371,1.,-1.92753067150476));
#30319=CARTESIAN_POINT('Ctrl Pts',(-0.459081234547926,1.,-1.93269066517934));
#30320=CARTESIAN_POINT('Ctrl Pts',(-0.462340031009056,1.,-1.93781486640821));
#30321=CARTESIAN_POINT('Ctrl Pts',(-0.46564546202603,1.,-1.9428979419619));
#30322=CARTESIAN_POINT('Ctrl Pts',(-0.468997482913135,1.,-1.94794381136514));
#30323=CARTESIAN_POINT('Ctrl Pts',(-0.472397672264072,1.,-1.95296148278133));
#30324=CARTESIAN_POINT('Ctrl Pts',(-0.475848034683176,1.,-1.95796111148177));
#30325=CARTESIAN_POINT('Ctrl Pts',(-0.479349583074855,1.,-1.96294933055943));
#30326=CARTESIAN_POINT('Ctrl Pts',(-0.482901662120691,1.,-1.96792703422362));
#30327=CARTESIAN_POINT('Ctrl Pts',(-0.486502692907659,1.,-1.97289186263272));
#30328=CARTESIAN_POINT('Ctrl Pts',(-0.490150627860952,1.,-1.97783973019229));
#30329=CARTESIAN_POINT('Ctrl Pts',(-0.493843476541495,1.,-1.98276658761821));
#30330=CARTESIAN_POINT('Ctrl Pts',(-0.497579909545574,1.,-1.98767044752932));
#30331=CARTESIAN_POINT('Ctrl Pts',(-0.501359287727146,1.,-1.99255149126155));
#30332=CARTESIAN_POINT('Ctrl Pts',(-0.505181361323026,1.,-1.99741107463572));
#30333=CARTESIAN_POINT('Ctrl Pts',(-0.509046069886157,1.,-2.00225107134734));
#30334=CARTESIAN_POINT('Ctrl Pts',(-0.512953306961792,1.,-2.00707309946949));
#30335=CARTESIAN_POINT('Ctrl Pts',(-0.516902681728687,1.,-2.01187773939242));
#30336=CARTESIAN_POINT('Ctrl Pts',(-0.52089359039937,1.,-2.01666477917286));
#30337=CARTESIAN_POINT('Ctrl Pts',(-0.524925318333476,1.,-2.02143356304698));
#30338=CARTESIAN_POINT('Ctrl Pts',(-0.528997127241914,1.,-2.0261832908329));
#30339=CARTESIAN_POINT('Ctrl Pts',(-0.533108355132977,1.,-2.03091336214426));
#30340=CARTESIAN_POINT('Ctrl Pts',(-0.537258489833262,1.,-2.03562362954037));
#30341=CARTESIAN_POINT('Ctrl Pts',(-0.541447120615659,1.,-2.04031422690527));
#30342=CARTESIAN_POINT('Ctrl Pts',(-0.54567390381743,1.,-2.04498544714588));
#30343=CARTESIAN_POINT('Ctrl Pts',(-0.549938525150295,1.,-2.04963761077958));
#30344=CARTESIAN_POINT('Ctrl Pts',(-0.554240657463906,1.,-2.05427091604413));
#30345=CARTESIAN_POINT('Ctrl Pts',(-0.558579940185151,1.,-2.05888537756462));
#30346=CARTESIAN_POINT('Ctrl Pts',(-0.562955993082261,1.,-2.06348090160589));
#30347=CARTESIAN_POINT('Ctrl Pts',(-0.567368421181087,1.,-2.06805732997334));
#30348=CARTESIAN_POINT('Ctrl Pts',(-0.571816823242603,1.,-2.07261449292824));
#30349=CARTESIAN_POINT('Ctrl Pts',(-0.576300797416844,1.,-2.07715226767559));
#30350=CARTESIAN_POINT('Ctrl Pts',(-0.580819952108063,1.,-2.08167059018418));
#30351=CARTESIAN_POINT('Ctrl Pts',(-0.585373918991617,1.,-2.08616943727951));
#30352=CARTESIAN_POINT('Ctrl Pts',(-0.589962365403406,1.,-2.09064881812129));
#30353=CARTESIAN_POINT('Ctrl Pts',(-0.594585006052162,1.,-2.0951087622027));
#30354=CARTESIAN_POINT('Ctrl Pts',(-0.599241616420533,1.,-2.0995493086477));
#30355=CARTESIAN_POINT('Ctrl Pts',(-0.60393203073603,1.,-2.10397049886949));
#30356=CARTESIAN_POINT('Ctrl Pts',(-0.607711315454876,1.,-2.1074919961518));
#30357=CARTESIAN_POINT('Ctrl Pts',(-0.610560911689899,1.,-2.11012443807238));
#30358=CARTESIAN_POINT('Ctrl Pts',(-0.6124673655618,1.,-2.11187554259986));
#30359=CARTESIAN_POINT('Ctrl Pts',(-0.61342227326009,1.,-2.11275013067528));
#30360=CARTESIAN_POINT('',(-0.383122945602003,0.,-1.7075470150345));
#30361=CARTESIAN_POINT('Origin',(0.,0.,0.));
#30362=CARTESIAN_POINT('',(-0.163289472382896,1.,-1.74236521665491));
#30363=CARTESIAN_POINT('Origin',(0.,1.,0.));
#30364=CARTESIAN_POINT('',(-0.163289472382896,0.,-1.74236521665491));
#30365=CARTESIAN_POINT('Ctrl Pts',(-0.0694764450219581,-1.,-2.19890268624765));
#30366=CARTESIAN_POINT('Ctrl Pts',(-0.0694764450219581,1.,-2.19890268624765));
#30367=CARTESIAN_POINT('Ctrl Pts',(-0.070114353632549,-1.,-2.19777582085423));
#30368=CARTESIAN_POINT('Ctrl Pts',(-0.070114353632549,1.,-2.19777582085423));
#30369=CARTESIAN_POINT('Ctrl Pts',(-0.0713863779526154,-1.,-2.19552129484002));
#30370=CARTESIAN_POINT('Ctrl Pts',(-0.0713863779526154,1.,-2.19552129484002));
#30371=CARTESIAN_POINT('Ctrl Pts',(-0.0732830357306725,-1.,-2.19213712013662));
#30372=CARTESIAN_POINT('Ctrl Pts',(-0.0732830357306725,1.,-2.19213712013662));
#30373=CARTESIAN_POINT('Ctrl Pts',(-0.0757891465836148,-1.,-2.1876201139953));
#30374=CARTESIAN_POINT('Ctrl Pts',(-0.0757891465836148,1.,-2.1876201139953));
#30375=CARTESIAN_POINT('Ctrl Pts',(-0.0788837727685243,-1.,-2.18196589448887));
#30376=CARTESIAN_POINT('Ctrl Pts',(-0.0788837727685243,1.,-2.18196589448887));
#30377=CARTESIAN_POINT('Ctrl Pts',(-0.0819402680872765,-1.,-2.176303712113));
#30378=CARTESIAN_POINT('Ctrl Pts',(-0.0819402680872765,1.,-2.176303712113));
#30379=CARTESIAN_POINT('Ctrl Pts',(-0.0849584620835372,-1.,-2.17063357870952));
#30380=CARTESIAN_POINT('Ctrl Pts',(-0.0849584620835372,1.,-2.17063357870952));
#30381=CARTESIAN_POINT('Ctrl Pts',(-0.0879381291386923,-1.,-2.16495552645014));
#30382=CARTESIAN_POINT('Ctrl Pts',(-0.0879381291386923,1.,-2.16495552645014));
#30383=CARTESIAN_POINT('Ctrl Pts',(-0.0908789888107265,-1.,-2.15926961544516));
#30384=CARTESIAN_POINT('Ctrl Pts',(-0.0908789888107265,1.,-2.15926961544516));
#30385=CARTESIAN_POINT('Ctrl Pts',(-0.0937807218867643,-1.,-2.1535759397817));
#30386=CARTESIAN_POINT('Ctrl Pts',(-0.0937807218867643,1.,-2.1535759397817));
#30387=CARTESIAN_POINT('Ctrl Pts',(-0.0966429852305459,-1.,-2.14787463531795));
#30388=CARTESIAN_POINT('Ctrl Pts',(-0.0966429852305459,1.,-2.14787463531795));
#30389=CARTESIAN_POINT('Ctrl Pts',(-0.0994654261990915,-1.,-2.14216588396025));
#30390=CARTESIAN_POINT('Ctrl Pts',(-0.0994654261990915,1.,-2.14216588396025));
#30391=CARTESIAN_POINT('Ctrl Pts',(-0.1022477005561,-1.,-2.13644992667165));
#30392=CARTESIAN_POINT('Ctrl Pts',(-0.1022477005561,1.,-2.13644992667165));
#30393=CARTESIAN_POINT('Ctrl Pts',(-0.104989479152739,-1.,-2.13072704887293));
#30394=CARTESIAN_POINT('Ctrl Pts',(-0.104989479152739,1.,-2.13072704887293));
#30395=CARTESIAN_POINT('Ctrl Pts',(-0.10769043523109,-1.,-2.12499752307));
#30396=CARTESIAN_POINT('Ctrl Pts',(-0.10769043523109,1.,-2.12499752307));
#30397=CARTESIAN_POINT('Ctrl Pts',(-0.110350236135025,-1.,-2.11926155590865));
#30398=CARTESIAN_POINT('Ctrl Pts',(-0.110350236135025,1.,-2.11926155590865));
#30399=CARTESIAN_POINT('Ctrl Pts',(-0.112968534419737,-1.,-2.11351924490306));
#30400=CARTESIAN_POINT('Ctrl Pts',(-0.112968534419737,1.,-2.11351924490306));
#30401=CARTESIAN_POINT('Ctrl Pts',(-0.115544957687926,-1.,-2.10777050261309));
#30402=CARTESIAN_POINT('Ctrl Pts',(-0.115544957687926,1.,-2.10777050261309));
#30403=CARTESIAN_POINT('Ctrl Pts',(-0.118079107988355,-1.,-2.102015121329));
#30404=CARTESIAN_POINT('Ctrl Pts',(-0.118079107988355,1.,-2.102015121329));
#30405=CARTESIAN_POINT('Ctrl Pts',(-0.120570567965122,-1.,-2.0962529286773));
#30406=CARTESIAN_POINT('Ctrl Pts',(-0.120570567965122,1.,-2.0962529286773));
#30407=CARTESIAN_POINT('Ctrl Pts',(-0.123018905621083,-1.,-2.09048392424825));
#30408=CARTESIAN_POINT('Ctrl Pts',(-0.123018905621083,1.,-2.09048392424825));
#30409=CARTESIAN_POINT('Ctrl Pts',(-0.125423679412061,-1.,-2.08470840653643));
#30410=CARTESIAN_POINT('Ctrl Pts',(-0.125423679412061,1.,-2.08470840653643));
#30411=CARTESIAN_POINT('Ctrl Pts',(-0.12778444527612,-1.,-2.07892715110987));
#30412=CARTESIAN_POINT('Ctrl Pts',(-0.12778444527612,1.,-2.07892715110987));
#30413=CARTESIAN_POINT('Ctrl Pts',(-0.130100748328403,-1.,-2.07314114713063));
#30414=CARTESIAN_POINT('Ctrl Pts',(-0.130100748328403,1.,-2.07314114713063));
#30415=CARTESIAN_POINT('Ctrl Pts',(-0.13237211154771,-1.,-2.06735123910326));
#30416=CARTESIAN_POINT('Ctrl Pts',(-0.13237211154771,1.,-2.06735123910326));
#30417=CARTESIAN_POINT('Ctrl Pts',(-0.134598026192106,-1.,-2.06155781517842));
#30418=CARTESIAN_POINT('Ctrl Pts',(-0.134598026192106,1.,-2.06155781517842));
#30419=CARTESIAN_POINT('Ctrl Pts',(-0.136777941218044,-1.,-2.05576044414264));
#30420=CARTESIAN_POINT('Ctrl Pts',(-0.136777941218044,1.,-2.05576044414264));
#30421=CARTESIAN_POINT('Ctrl Pts',(-0.138911255368966,-1.,-2.04995762001328));
#30422=CARTESIAN_POINT('Ctrl Pts',(-0.138911255368966,1.,-2.04995762001328));
#30423=CARTESIAN_POINT('Ctrl Pts',(-0.140997332152546,-1.,-2.04414757947916));
#30424=CARTESIAN_POINT('Ctrl Pts',(-0.140997332152546,1.,-2.04414757947916));
#30425=CARTESIAN_POINT('Ctrl Pts',(-0.143035515058209,-1.,-2.03832911025912));
#30426=CARTESIAN_POINT('Ctrl Pts',(-0.143035515058209,1.,-2.03832911025912));
#30427=CARTESIAN_POINT('Ctrl Pts',(-0.145025140186057,-1.,-2.03250223739942));
#30428=CARTESIAN_POINT('Ctrl Pts',(-0.145025140186057,1.,-2.03250223739942));
#30429=CARTESIAN_POINT('Ctrl Pts',(-0.146965557332583,-1.,-2.02666926182017));
#30430=CARTESIAN_POINT('Ctrl Pts',(-0.146965557332583,1.,-2.02666926182017));
#30431=CARTESIAN_POINT('Ctrl Pts',(-0.148856124775337,-1.,-2.02083464969894));
#30432=CARTESIAN_POINT('Ctrl Pts',(-0.148856124775337,1.,-2.02083464969894));
#30433=CARTESIAN_POINT('Ctrl Pts',(-0.150696157673078,-1.,-2.01500291940238));
#30434=CARTESIAN_POINT('Ctrl Pts',(-0.150696157673078,1.,-2.01500291940238));
#30435=CARTESIAN_POINT('Ctrl Pts',(-0.15248488362145,-1.,-2.00917680318424));
#30436=CARTESIAN_POINT('Ctrl Pts',(-0.15248488362145,1.,-2.00917680318424));
#30437=CARTESIAN_POINT('Ctrl Pts',(-0.154221403049722,-1.,-2.00335565310543));
#30438=CARTESIAN_POINT('Ctrl Pts',(-0.154221403049722,1.,-2.00335565310543));
#30439=CARTESIAN_POINT('Ctrl Pts',(-0.155904629548783,-1.,-1.99753284771497));
#30440=CARTESIAN_POINT('Ctrl Pts',(-0.155904629548783,1.,-1.99753284771497));
#30441=CARTESIAN_POINT('Ctrl Pts',(-0.157533331459227,-1.,-1.99169810931908));
#30442=CARTESIAN_POINT('Ctrl Pts',(-0.157533331459227,1.,-1.99169810931908));
#30443=CARTESIAN_POINT('Ctrl Pts',(-0.159106226437299,-1.,-1.98584238283292));
#30444=CARTESIAN_POINT('Ctrl Pts',(-0.159106226437299,1.,-1.98584238283292));
#30445=CARTESIAN_POINT('Ctrl Pts',(-0.160622060784611,-1.,-1.97996195437559));
#30446=CARTESIAN_POINT('Ctrl Pts',(-0.160622060784611,1.,-1.97996195437559));
#30447=CARTESIAN_POINT('Ctrl Pts',(-0.162079693556289,-1.,-1.97406280235188));
#30448=CARTESIAN_POINT('Ctrl Pts',(-0.162079693556289,1.,-1.97406280235188));
#30449=CARTESIAN_POINT('Ctrl Pts',(-0.163478185457734,-1.,-1.96816512677967));
#30450=CARTESIAN_POINT('Ctrl Pts',(-0.163478185457734,1.,-1.96816512677967));
#30451=CARTESIAN_POINT('Ctrl Pts',(-0.164816568920269,-1.,-1.96229379940136));
#30452=CARTESIAN_POINT('Ctrl Pts',(-0.164816568920269,1.,-1.96229379940136));
#30453=CARTESIAN_POINT('Ctrl Pts',(-0.166093592002812,-1.,-1.9564675971873));
#30454=CARTESIAN_POINT('Ctrl Pts',(-0.166093592002812,1.,-1.9564675971873));
#30455=CARTESIAN_POINT('Ctrl Pts',(-0.167307501784475,-1.,-1.95069027794294));
#30456=CARTESIAN_POINT('Ctrl Pts',(-0.167307501784475,1.,-1.95069027794294));
#30457=CARTESIAN_POINT('Ctrl Pts',(-0.168455741607556,-1.,-1.94493757756931));
#30458=CARTESIAN_POINT('Ctrl Pts',(-0.168455741607556,1.,-1.94493757756931));
#30459=CARTESIAN_POINT('Ctrl Pts',(-0.169534904817491,-1.,-1.93915639211581));
#30460=CARTESIAN_POINT('Ctrl Pts',(-0.169534904817491,1.,-1.93915639211581));
#30461=CARTESIAN_POINT('Ctrl Pts',(-0.170541253116202,-1.,-1.93329183155539));
#30462=CARTESIAN_POINT('Ctrl Pts',(-0.170541253116202,1.,-1.93329183155539));
#30463=CARTESIAN_POINT('Ctrl Pts',(-0.171471191532988,-1.,-1.92731093582036));
#30464=CARTESIAN_POINT('Ctrl Pts',(-0.171471191532988,1.,-1.92731093582036));
#30465=CARTESIAN_POINT('Ctrl Pts',(-0.172321621259514,-1.,-1.9212233439798));
#30466=CARTESIAN_POINT('Ctrl Pts',(-0.172321621259514,1.,-1.9212233439798));
#30467=CARTESIAN_POINT('Ctrl Pts',(-0.173090695383496,-1.,-1.91511429159527));
#30468=CARTESIAN_POINT('Ctrl Pts',(-0.173090695383496,1.,-1.91511429159527));
#30469=CARTESIAN_POINT('Ctrl Pts',(-0.173776635257817,-1.,-1.90911693975267));
#30470=CARTESIAN_POINT('Ctrl Pts',(-0.173776635257817,1.,-1.90911693975267));
#30471=CARTESIAN_POINT('Ctrl Pts',(-0.174375518661085,-1.,-1.90335253862834));
#30472=CARTESIAN_POINT('Ctrl Pts',(-0.174375518661085,1.,-1.90335253862834));
#30473=CARTESIAN_POINT('Ctrl Pts',(-0.174879405091263,-1.,-1.89788101117132));
#30474=CARTESIAN_POINT('Ctrl Pts',(-0.174879405091263,1.,-1.89788101117132));
#30475=CARTESIAN_POINT('Ctrl Pts',(-0.175274276190844,-1.,-1.892646301985));
#30476=CARTESIAN_POINT('Ctrl Pts',(-0.175274276190844,1.,-1.892646301985));
#30477=CARTESIAN_POINT('Ctrl Pts',(-0.175538155840648,-1.,-1.88742606273259));
#30478=CARTESIAN_POINT('Ctrl Pts',(-0.175538155840648,1.,-1.88742606273259));
#30479=CARTESIAN_POINT('Ctrl Pts',(-0.175644148889699,-1.,-1.88188663145367));
#30480=CARTESIAN_POINT('Ctrl Pts',(-0.175644148889699,1.,-1.88188663145367));
#30481=CARTESIAN_POINT('Ctrl Pts',(-0.175563480746485,-1.,-1.87563767773588));
#30482=CARTESIAN_POINT('Ctrl Pts',(-0.175563480746485,1.,-1.87563767773588));
#30483=CARTESIAN_POINT('Ctrl Pts',(-0.175268337590758,-1.,-1.86828349694799));
#30484=CARTESIAN_POINT('Ctrl Pts',(-0.175268337590758,1.,-1.86828349694799));
#30485=CARTESIAN_POINT('Ctrl Pts',(-0.17473525927603,-1.,-1.85948367088837));
#30486=CARTESIAN_POINT('Ctrl Pts',(-0.17473525927603,1.,-1.85948367088837));
#30487=CARTESIAN_POINT('Ctrl Pts',(-0.173946627587731,-1.,-1.8489811319852));
#30488=CARTESIAN_POINT('Ctrl Pts',(-0.173946627587731,1.,-1.8489811319852));
#30489=CARTESIAN_POINT('Ctrl Pts',(-0.1728894428919,-1.,-1.83658380527692));
#30490=CARTESIAN_POINT('Ctrl Pts',(-0.1728894428919,1.,-1.83658380527692));
#30491=CARTESIAN_POINT('Ctrl Pts',(-0.171554770204119,-1.,-1.82215766811545));
#30492=CARTESIAN_POINT('Ctrl Pts',(-0.171554770204119,1.,-1.82215766811545));
#30493=CARTESIAN_POINT('Ctrl Pts',(-0.169936923904608,-1.,-1.80561530629706));
#30494=CARTESIAN_POINT('Ctrl Pts',(-0.169936923904608,1.,-1.80561530629706));
#30495=CARTESIAN_POINT('Ctrl Pts',(-0.168032772805197,-1.,-1.7869064998507));
#30496=CARTESIAN_POINT('Ctrl Pts',(-0.168032772805197,1.,-1.7869064998507));
#30497=CARTESIAN_POINT('Ctrl Pts',(-0.1662793551464,-1.,-1.77018771684844));
#30498=CARTESIAN_POINT('Ctrl Pts',(-0.1662793551464,1.,-1.77018771684844));
#30499=CARTESIAN_POINT('Ctrl Pts',(-0.164834765707158,-1.,-1.75666056638427));
#30500=CARTESIAN_POINT('Ctrl Pts',(-0.164834765707158,1.,-1.75666056638427));
#30501=CARTESIAN_POINT('Ctrl Pts',(-0.163814161002002,-1.,-1.7472034950333));
#30502=CARTESIAN_POINT('Ctrl Pts',(-0.163814161002002,1.,-1.7472034950333));
#30503=CARTESIAN_POINT('Ctrl Pts',(-0.163289472382896,-1.,-1.74236521665491));
#30504=CARTESIAN_POINT('Ctrl Pts',(-0.163289472382896,1.,-1.74236521665491));
#30505=CARTESIAN_POINT('',(-0.0694764450219581,1.,-2.19890268624765));
#30506=CARTESIAN_POINT('Ctrl Pts',(-0.0694764450219581,1.,-2.19890268624765));
#30507=CARTESIAN_POINT('Ctrl Pts',(-0.070114353632549,1.,-2.19777582085423));
#30508=CARTESIAN_POINT('Ctrl Pts',(-0.0713863779526154,1.,-2.19552129484002));
#30509=CARTESIAN_POINT('Ctrl Pts',(-0.0732830357306725,1.,-2.19213712013662));
#30510=CARTESIAN_POINT('Ctrl Pts',(-0.0757891465836148,1.,-2.1876201139953));
#30511=CARTESIAN_POINT('Ctrl Pts',(-0.0788837727685243,1.,-2.18196589448887));
#30512=CARTESIAN_POINT('Ctrl Pts',(-0.0819402680872765,1.,-2.176303712113));
#30513=CARTESIAN_POINT('Ctrl Pts',(-0.0849584620835372,1.,-2.17063357870952));
#30514=CARTESIAN_POINT('Ctrl Pts',(-0.0879381291386923,1.,-2.16495552645014));
#30515=CARTESIAN_POINT('Ctrl Pts',(-0.0908789888107265,1.,-2.15926961544516));
#30516=CARTESIAN_POINT('Ctrl Pts',(-0.0937807218867643,1.,-2.1535759397817));
#30517=CARTESIAN_POINT('Ctrl Pts',(-0.0966429852305459,1.,-2.14787463531795));
#30518=CARTESIAN_POINT('Ctrl Pts',(-0.0994654261990915,1.,-2.14216588396025));
#30519=CARTESIAN_POINT('Ctrl Pts',(-0.1022477005561,1.,-2.13644992667165));
#30520=CARTESIAN_POINT('Ctrl Pts',(-0.104989479152739,1.,-2.13072704887293));
#30521=CARTESIAN_POINT('Ctrl Pts',(-0.10769043523109,1.,-2.12499752307));
#30522=CARTESIAN_POINT('Ctrl Pts',(-0.110350236135025,1.,-2.11926155590865));
#30523=CARTESIAN_POINT('Ctrl Pts',(-0.112968534419737,1.,-2.11351924490306));
#30524=CARTESIAN_POINT('Ctrl Pts',(-0.115544957687926,1.,-2.10777050261309));
#30525=CARTESIAN_POINT('Ctrl Pts',(-0.118079107988355,1.,-2.102015121329));
#30526=CARTESIAN_POINT('Ctrl Pts',(-0.120570567965122,1.,-2.0962529286773));
#30527=CARTESIAN_POINT('Ctrl Pts',(-0.123018905621083,1.,-2.09048392424825));
#30528=CARTESIAN_POINT('Ctrl Pts',(-0.125423679412061,1.,-2.08470840653643));
#30529=CARTESIAN_POINT('Ctrl Pts',(-0.12778444527612,1.,-2.07892715110987));
#30530=CARTESIAN_POINT('Ctrl Pts',(-0.130100748328403,1.,-2.07314114713063));
#30531=CARTESIAN_POINT('Ctrl Pts',(-0.13237211154771,1.,-2.06735123910326));
#30532=CARTESIAN_POINT('Ctrl Pts',(-0.134598026192106,1.,-2.06155781517842));
#30533=CARTESIAN_POINT('Ctrl Pts',(-0.136777941218044,1.,-2.05576044414264));
#30534=CARTESIAN_POINT('Ctrl Pts',(-0.138911255368966,1.,-2.04995762001328));
#30535=CARTESIAN_POINT('Ctrl Pts',(-0.140997332152546,1.,-2.04414757947916));
#30536=CARTESIAN_POINT('Ctrl Pts',(-0.143035515058209,1.,-2.03832911025912));
#30537=CARTESIAN_POINT('Ctrl Pts',(-0.145025140186057,1.,-2.03250223739942));
#30538=CARTESIAN_POINT('Ctrl Pts',(-0.146965557332583,1.,-2.02666926182017));
#30539=CARTESIAN_POINT('Ctrl Pts',(-0.148856124775337,1.,-2.02083464969894));
#30540=CARTESIAN_POINT('Ctrl Pts',(-0.150696157673078,1.,-2.01500291940238));
#30541=CARTESIAN_POINT('Ctrl Pts',(-0.15248488362145,1.,-2.00917680318424));
#30542=CARTESIAN_POINT('Ctrl Pts',(-0.154221403049722,1.,-2.00335565310543));
#30543=CARTESIAN_POINT('Ctrl Pts',(-0.155904629548783,1.,-1.99753284771497));
#30544=CARTESIAN_POINT('Ctrl Pts',(-0.157533331459227,1.,-1.99169810931908));
#30545=CARTESIAN_POINT('Ctrl Pts',(-0.159106226437299,1.,-1.98584238283292));
#30546=CARTESIAN_POINT('Ctrl Pts',(-0.160622060784611,1.,-1.97996195437559));
#30547=CARTESIAN_POINT('Ctrl Pts',(-0.162079693556289,1.,-1.97406280235188));
#30548=CARTESIAN_POINT('Ctrl Pts',(-0.163478185457734,1.,-1.96816512677967));
#30549=CARTESIAN_POINT('Ctrl Pts',(-0.164816568920269,1.,-1.96229379940136));
#30550=CARTESIAN_POINT('Ctrl Pts',(-0.166093592002812,1.,-1.9564675971873));
#30551=CARTESIAN_POINT('Ctrl Pts',(-0.167307501784475,1.,-1.95069027794294));
#30552=CARTESIAN_POINT('Ctrl Pts',(-0.168455741607556,1.,-1.94493757756931));
#30553=CARTESIAN_POINT('Ctrl Pts',(-0.169534904817491,1.,-1.93915639211581));
#30554=CARTESIAN_POINT('Ctrl Pts',(-0.170541253116202,1.,-1.93329183155539));
#30555=CARTESIAN_POINT('Ctrl Pts',(-0.171471191532988,1.,-1.92731093582036));
#30556=CARTESIAN_POINT('Ctrl Pts',(-0.172321621259514,1.,-1.9212233439798));
#30557=CARTESIAN_POINT('Ctrl Pts',(-0.173090695383496,1.,-1.91511429159527));
#30558=CARTESIAN_POINT('Ctrl Pts',(-0.173776635257817,1.,-1.90911693975267));
#30559=CARTESIAN_POINT('Ctrl Pts',(-0.174375518661085,1.,-1.90335253862834));
#30560=CARTESIAN_POINT('Ctrl Pts',(-0.174879405091263,1.,-1.89788101117132));
#30561=CARTESIAN_POINT('Ctrl Pts',(-0.175274276190844,1.,-1.892646301985));
#30562=CARTESIAN_POINT('Ctrl Pts',(-0.175538155840648,1.,-1.88742606273259));
#30563=CARTESIAN_POINT('Ctrl Pts',(-0.175644148889699,1.,-1.88188663145367));
#30564=CARTESIAN_POINT('Ctrl Pts',(-0.175563480746485,1.,-1.87563767773588));
#30565=CARTESIAN_POINT('Ctrl Pts',(-0.175268337590758,1.,-1.86828349694799));
#30566=CARTESIAN_POINT('Ctrl Pts',(-0.17473525927603,1.,-1.85948367088837));
#30567=CARTESIAN_POINT('Ctrl Pts',(-0.173946627587731,1.,-1.8489811319852));
#30568=CARTESIAN_POINT('Ctrl Pts',(-0.1728894428919,1.,-1.83658380527692));
#30569=CARTESIAN_POINT('Ctrl Pts',(-0.171554770204119,1.,-1.82215766811545));
#30570=CARTESIAN_POINT('Ctrl Pts',(-0.169936923904608,1.,-1.80561530629706));
#30571=CARTESIAN_POINT('Ctrl Pts',(-0.168032772805197,1.,-1.7869064998507));
#30572=CARTESIAN_POINT('Ctrl Pts',(-0.1662793551464,1.,-1.77018771684844));
#30573=CARTESIAN_POINT('Ctrl Pts',(-0.164834765707158,1.,-1.75666056638427));
#30574=CARTESIAN_POINT('Ctrl Pts',(-0.163814161002002,1.,-1.7472034950333));
#30575=CARTESIAN_POINT('Ctrl Pts',(-0.163289472382896,1.,-1.74236521665491));
#30576=CARTESIAN_POINT('',(-0.0694764450219581,0.,-2.19890268624765));
#30577=CARTESIAN_POINT('Origin',(0.0694764450219584,0.,-2.19890268624765));
#30578=CARTESIAN_POINT('',(0.0694764450219584,1.,-2.19890268624765));
#30579=CARTESIAN_POINT('',(-0.0694764450219581,1.,-2.19890268624765));
#30580=CARTESIAN_POINT('',(0.0694764450219584,0.,-2.19890268624765));
#30581=CARTESIAN_POINT('Ctrl Pts',(0.163289472382896,-1.,-1.74236521665491));
#30582=CARTESIAN_POINT('Ctrl Pts',(0.163289472382896,1.,-1.74236521665491));
#30583=CARTESIAN_POINT('Ctrl Pts',(0.163814161002474,-1.,-1.74720349503904));
#30584=CARTESIAN_POINT('Ctrl Pts',(0.163814161002474,1.,-1.74720349503904));
#30585=CARTESIAN_POINT('Ctrl Pts',(0.164834765708484,-1.,-1.75666056640041));
#30586=CARTESIAN_POINT('Ctrl Pts',(0.164834765708484,1.,-1.75666056640041));
#30587=CARTESIAN_POINT('Ctrl Pts',(0.166279355148738,-1.,-1.77018771687692));
#30588=CARTESIAN_POINT('Ctrl Pts',(0.166279355148738,1.,-1.77018771687692));
#30589=CARTESIAN_POINT('Ctrl Pts',(0.16803277280837,-1.,-1.78690649988931));
#30590=CARTESIAN_POINT('Ctrl Pts',(0.16803277280837,1.,-1.78690649988931));
#30591=CARTESIAN_POINT('Ctrl Pts',(0.169936923908078,-1.,-1.80561530633924));
#30592=CARTESIAN_POINT('Ctrl Pts',(0.169936923908078,1.,-1.80561530633924));
#30593=CARTESIAN_POINT('Ctrl Pts',(0.171554770207306,-1.,-1.82215766815414));
#30594=CARTESIAN_POINT('Ctrl Pts',(0.171554770207306,1.,-1.82215766815414));
#30595=CARTESIAN_POINT('Ctrl Pts',(0.17288944289442,-1.,-1.83658380530747));
#30596=CARTESIAN_POINT('Ctrl Pts',(0.17288944289442,1.,-1.83658380530747));
#30597=CARTESIAN_POINT('Ctrl Pts',(0.173946627589401,-1.,-1.84898113200543));
#30598=CARTESIAN_POINT('Ctrl Pts',(0.173946627589401,1.,-1.84898113200543));
#30599=CARTESIAN_POINT('Ctrl Pts',(0.174735259276856,-1.,-1.85948367089838));
#30600=CARTESIAN_POINT('Ctrl Pts',(0.174735259276856,1.,-1.85948367089838));
#30601=CARTESIAN_POINT('Ctrl Pts',(0.175268337590901,-1.,-1.86828349694972));
#30602=CARTESIAN_POINT('Ctrl Pts',(0.175268337590901,1.,-1.86828349694972));
#30603=CARTESIAN_POINT('Ctrl Pts',(0.175563480746205,-1.,-1.87563767773249));
#30604=CARTESIAN_POINT('Ctrl Pts',(0.175563480746205,1.,-1.87563767773249));
#30605=CARTESIAN_POINT('Ctrl Pts',(0.175644148889271,-1.,-1.88188663144846));
#30606=CARTESIAN_POINT('Ctrl Pts',(0.175644148889271,1.,-1.88188663144846));
#30607=CARTESIAN_POINT('Ctrl Pts',(0.175538155840286,-1.,-1.88742606272818));
#30608=CARTESIAN_POINT('Ctrl Pts',(0.175538155840286,1.,-1.88742606272818));
#30609=CARTESIAN_POINT('Ctrl Pts',(0.175274276190664,-1.,-1.89264630198279));
#30610=CARTESIAN_POINT('Ctrl Pts',(0.175274276190664,1.,-1.89264630198279));
#30611=CARTESIAN_POINT('Ctrl Pts',(0.174879405091277,-1.,-1.89788101117148));
#30612=CARTESIAN_POINT('Ctrl Pts',(0.174879405091277,1.,-1.89788101117148));
#30613=CARTESIAN_POINT('Ctrl Pts',(0.174375518661222,-1.,-1.90335253863003));
#30614=CARTESIAN_POINT('Ctrl Pts',(0.174375518661222,1.,-1.90335253863003));
#30615=CARTESIAN_POINT('Ctrl Pts',(0.173776635257984,-1.,-1.90911693975475));
#30616=CARTESIAN_POINT('Ctrl Pts',(0.173776635257984,1.,-1.90911693975475));
#30617=CARTESIAN_POINT('Ctrl Pts',(0.173090695383619,-1.,-1.91511429159681));
#30618=CARTESIAN_POINT('Ctrl Pts',(0.173090695383619,1.,-1.91511429159681));
#30619=CARTESIAN_POINT('Ctrl Pts',(0.172321621259557,-1.,-1.92122334398034));
#30620=CARTESIAN_POINT('Ctrl Pts',(0.172321621259557,1.,-1.92122334398034));
#30621=CARTESIAN_POINT('Ctrl Pts',(0.17147119153296,-1.,-1.92731093582));
#30622=CARTESIAN_POINT('Ctrl Pts',(0.17147119153296,1.,-1.92731093582));
#30623=CARTESIAN_POINT('Ctrl Pts',(0.170541253116136,-1.,-1.93329183155455));
#30624=CARTESIAN_POINT('Ctrl Pts',(0.170541253116136,1.,-1.93329183155455));
#30625=CARTESIAN_POINT('Ctrl Pts',(0.169534904817425,-1.,-1.93915639211497));
#30626=CARTESIAN_POINT('Ctrl Pts',(0.169534904817425,1.,-1.93915639211497));
#30627=CARTESIAN_POINT('Ctrl Pts',(0.168455741607516,-1.,-1.94493757756879));
#30628=CARTESIAN_POINT('Ctrl Pts',(0.168455741607516,1.,-1.94493757756879));
#30629=CARTESIAN_POINT('Ctrl Pts',(0.167307501784469,-1.,-1.95069027794286));
#30630=CARTESIAN_POINT('Ctrl Pts',(0.167307501784469,1.,-1.95069027794286));
#30631=CARTESIAN_POINT('Ctrl Pts',(0.166093592002833,-1.,-1.95646759718755));
#30632=CARTESIAN_POINT('Ctrl Pts',(0.166093592002833,1.,-1.95646759718755));
#30633=CARTESIAN_POINT('Ctrl Pts',(0.1648165689203,-1.,-1.96229379940174));
#30634=CARTESIAN_POINT('Ctrl Pts',(0.1648165689203,1.,-1.96229379940174));
#30635=CARTESIAN_POINT('Ctrl Pts',(0.16347818545776,-1.,-1.96816512678));
#30636=CARTESIAN_POINT('Ctrl Pts',(0.16347818545776,1.,-1.96816512678));
#30637=CARTESIAN_POINT('Ctrl Pts',(0.162079693556302,-1.,-1.97406280235204));
#30638=CARTESIAN_POINT('Ctrl Pts',(0.162079693556302,1.,-1.97406280235204));
#30639=CARTESIAN_POINT('Ctrl Pts',(0.16062206078461,-1.,-1.97996195437557));
#30640=CARTESIAN_POINT('Ctrl Pts',(0.16062206078461,1.,-1.97996195437557));
#30641=CARTESIAN_POINT('Ctrl Pts',(0.159106226437288,-1.,-1.98584238283279));
#30642=CARTESIAN_POINT('Ctrl Pts',(0.159106226437288,1.,-1.98584238283279));
#30643=CARTESIAN_POINT('Ctrl Pts',(0.157533331459215,-1.,-1.99169810931893));
#30644=CARTESIAN_POINT('Ctrl Pts',(0.157533331459215,1.,-1.99169810931893));
#30645=CARTESIAN_POINT('Ctrl Pts',(0.155904629548774,-1.,-1.99753284771487));
#30646=CARTESIAN_POINT('Ctrl Pts',(0.155904629548774,1.,-1.99753284771487));
#30647=CARTESIAN_POINT('Ctrl Pts',(0.154221403049719,-1.,-2.00335565310539));
#30648=CARTESIAN_POINT('Ctrl Pts',(0.154221403049719,1.,-2.00335565310539));
#30649=CARTESIAN_POINT('Ctrl Pts',(0.152484883621452,-1.,-2.00917680318426));
#30650=CARTESIAN_POINT('Ctrl Pts',(0.152484883621452,1.,-2.00917680318426));
#30651=CARTESIAN_POINT('Ctrl Pts',(0.150696157673084,-1.,-2.01500291940243));
#30652=CARTESIAN_POINT('Ctrl Pts',(0.150696157673084,1.,-2.01500291940243));
#30653=CARTESIAN_POINT('Ctrl Pts',(0.148856124775343,-1.,-2.02083464969897));
#30654=CARTESIAN_POINT('Ctrl Pts',(0.148856124775343,1.,-2.02083464969897));
#30655=CARTESIAN_POINT('Ctrl Pts',(0.146965557332586,-1.,-2.02666926182017));
#30656=CARTESIAN_POINT('Ctrl Pts',(0.146965557332586,1.,-2.02666926182017));
#30657=CARTESIAN_POINT('Ctrl Pts',(0.145025140186058,-1.,-2.03250223739941));
#30658=CARTESIAN_POINT('Ctrl Pts',(0.145025140186058,1.,-2.03250223739941));
#30659=CARTESIAN_POINT('Ctrl Pts',(0.143035515058208,-1.,-2.03832911025913));
#30660=CARTESIAN_POINT('Ctrl Pts',(0.143035515058208,1.,-2.03832911025913));
#30661=CARTESIAN_POINT('Ctrl Pts',(0.140997332152545,-1.,-2.04414757947919));
#30662=CARTESIAN_POINT('Ctrl Pts',(0.140997332152545,1.,-2.04414757947919));
#30663=CARTESIAN_POINT('Ctrl Pts',(0.138911255368966,-1.,-2.04995762001333));
#30664=CARTESIAN_POINT('Ctrl Pts',(0.138911255368966,1.,-2.04995762001333));
#30665=CARTESIAN_POINT('Ctrl Pts',(0.136777941218044,-1.,-2.0557604441427));
#30666=CARTESIAN_POINT('Ctrl Pts',(0.136777941218044,1.,-2.0557604441427));
#30667=CARTESIAN_POINT('Ctrl Pts',(0.134598026192107,-1.,-2.06155781517844));
#30668=CARTESIAN_POINT('Ctrl Pts',(0.134598026192107,1.,-2.06155781517844));
#30669=CARTESIAN_POINT('Ctrl Pts',(0.13237211154771,-1.,-2.06735123910319));
#30670=CARTESIAN_POINT('Ctrl Pts',(0.13237211154771,1.,-2.06735123910319));
#30671=CARTESIAN_POINT('Ctrl Pts',(0.1301007483284,-1.,-2.07314114713047));
#30672=CARTESIAN_POINT('Ctrl Pts',(0.1301007483284,1.,-2.07314114713047));
#30673=CARTESIAN_POINT('Ctrl Pts',(0.127784445276116,-1.,-2.07892715110967));
#30674=CARTESIAN_POINT('Ctrl Pts',(0.127784445276116,1.,-2.07892715110967));
#30675=CARTESIAN_POINT('Ctrl Pts',(0.125423679412058,-1.,-2.08470840653628));
#30676=CARTESIAN_POINT('Ctrl Pts',(0.125423679412058,1.,-2.08470840653628));
#30677=CARTESIAN_POINT('Ctrl Pts',(0.123018905621083,-1.,-2.09048392424826));
#30678=CARTESIAN_POINT('Ctrl Pts',(0.123018905621083,1.,-2.09048392424826));
#30679=CARTESIAN_POINT('Ctrl Pts',(0.120570567965129,-1.,-2.09625292867756));
#30680=CARTESIAN_POINT('Ctrl Pts',(0.120570567965129,1.,-2.09625292867756));
#30681=CARTESIAN_POINT('Ctrl Pts',(0.118079107988368,-1.,-2.10201512132945));
#30682=CARTESIAN_POINT('Ctrl Pts',(0.118079107988368,1.,-2.10201512132945));
#30683=CARTESIAN_POINT('Ctrl Pts',(0.11554495768794,-1.,-2.10777050261359));
#30684=CARTESIAN_POINT('Ctrl Pts',(0.11554495768794,1.,-2.10777050261359));
#30685=CARTESIAN_POINT('Ctrl Pts',(0.112968534419746,-1.,-2.11351924490335));
#30686=CARTESIAN_POINT('Ctrl Pts',(0.112968534419746,1.,-2.11351924490335));
#30687=CARTESIAN_POINT('Ctrl Pts',(0.11035023613502,-1.,-2.11926155590849));
#30688=CARTESIAN_POINT('Ctrl Pts',(0.11035023613502,1.,-2.11926155590849));
#30689=CARTESIAN_POINT('Ctrl Pts',(0.107690435231068,-1.,-2.12499752306927));
#30690=CARTESIAN_POINT('Ctrl Pts',(0.107690435231068,1.,-2.12499752306927));
#30691=CARTESIAN_POINT('Ctrl Pts',(0.104989479152703,-1.,-2.1307270488718));
#30692=CARTESIAN_POINT('Ctrl Pts',(0.104989479152703,1.,-2.1307270488718));
#30693=CARTESIAN_POINT('Ctrl Pts',(0.102247700556064,-1.,-2.13644992667052));
#30694=CARTESIAN_POINT('Ctrl Pts',(0.102247700556064,1.,-2.13644992667052));
#30695=CARTESIAN_POINT('Ctrl Pts',(0.0994654261990743,-1.,-2.14216588395974));
#30696=CARTESIAN_POINT('Ctrl Pts',(0.0994654261990743,1.,-2.14216588395974));
#30697=CARTESIAN_POINT('Ctrl Pts',(0.0966429852305689,-1.,-2.14787463531864));
#30698=CARTESIAN_POINT('Ctrl Pts',(0.0966429852305689,1.,-2.14787463531864));
#30699=CARTESIAN_POINT('Ctrl Pts',(0.0937807218868345,-1.,-2.15357593978377));
#30700=CARTESIAN_POINT('Ctrl Pts',(0.0937807218868345,1.,-2.15357593978377));
#30701=CARTESIAN_POINT('Ctrl Pts',(0.0908789888108266,-1.,-2.15926961544808));
#30702=CARTESIAN_POINT('Ctrl Pts',(0.0908789888108266,1.,-2.15926961544808));
#30703=CARTESIAN_POINT('Ctrl Pts',(0.0879381291387823,-1.,-2.16495552645275));
#30704=CARTESIAN_POINT('Ctrl Pts',(0.0879381291387823,1.,-2.16495552645275));
#30705=CARTESIAN_POINT('Ctrl Pts',(0.0849584620835643,-1.,-2.17063357871031));
#30706=CARTESIAN_POINT('Ctrl Pts',(0.0849584620835643,1.,-2.17063357871031));
#30707=CARTESIAN_POINT('Ctrl Pts',(0.0819402680871939,-1.,-2.1763037121106));
#30708=CARTESIAN_POINT('Ctrl Pts',(0.0819402680871939,1.,-2.1763037121106));
#30709=CARTESIAN_POINT('Ctrl Pts',(0.0788837727683228,-1.,-2.18196589448304));
#30710=CARTESIAN_POINT('Ctrl Pts',(0.0788837727683228,1.,-2.18196589448304));
#30711=CARTESIAN_POINT('Ctrl Pts',(0.0757891465833411,-1.,-2.1876201139874));
#30712=CARTESIAN_POINT('Ctrl Pts',(0.0757891465833411,1.,-2.1876201139874));
#30713=CARTESIAN_POINT('Ctrl Pts',(0.0732830357304276,-1.,-2.19213712012956));
#30714=CARTESIAN_POINT('Ctrl Pts',(0.0732830357304276,1.,-2.19213712012956));
#30715=CARTESIAN_POINT('Ctrl Pts',(0.0713863779524627,-1.,-2.19552129483562));
#30716=CARTESIAN_POINT('Ctrl Pts',(0.0713863779524627,1.,-2.19552129483562));
#30717=CARTESIAN_POINT('Ctrl Pts',(0.0701143536324926,-1.,-2.19777582085261));
#30718=CARTESIAN_POINT('Ctrl Pts',(0.0701143536324926,1.,-2.19777582085261));
#30719=CARTESIAN_POINT('Ctrl Pts',(0.0694764450219584,-1.,-2.19890268624765));
#30720=CARTESIAN_POINT('Ctrl Pts',(0.0694764450219584,1.,-2.19890268624765));
#30721=CARTESIAN_POINT('',(0.163289472382896,1.,-1.74236521665491));
#30722=CARTESIAN_POINT('Ctrl Pts',(0.163289472382896,1.,-1.74236521665491));
#30723=CARTESIAN_POINT('Ctrl Pts',(0.163814161002474,1.,-1.74720349503904));
#30724=CARTESIAN_POINT('Ctrl Pts',(0.164834765708484,1.,-1.75666056640041));
#30725=CARTESIAN_POINT('Ctrl Pts',(0.166279355148738,1.,-1.77018771687692));
#30726=CARTESIAN_POINT('Ctrl Pts',(0.16803277280837,1.,-1.78690649988931));
#30727=CARTESIAN_POINT('Ctrl Pts',(0.169936923908078,1.,-1.80561530633924));
#30728=CARTESIAN_POINT('Ctrl Pts',(0.171554770207306,1.,-1.82215766815414));
#30729=CARTESIAN_POINT('Ctrl Pts',(0.17288944289442,1.,-1.83658380530747));
#30730=CARTESIAN_POINT('Ctrl Pts',(0.173946627589401,1.,-1.84898113200543));
#30731=CARTESIAN_POINT('Ctrl Pts',(0.174735259276856,1.,-1.85948367089838));
#30732=CARTESIAN_POINT('Ctrl Pts',(0.175268337590901,1.,-1.86828349694972));
#30733=CARTESIAN_POINT('Ctrl Pts',(0.175563480746205,1.,-1.87563767773249));
#30734=CARTESIAN_POINT('Ctrl Pts',(0.175644148889271,1.,-1.88188663144846));
#30735=CARTESIAN_POINT('Ctrl Pts',(0.175538155840286,1.,-1.88742606272818));
#30736=CARTESIAN_POINT('Ctrl Pts',(0.175274276190664,1.,-1.89264630198279));
#30737=CARTESIAN_POINT('Ctrl Pts',(0.174879405091277,1.,-1.89788101117148));
#30738=CARTESIAN_POINT('Ctrl Pts',(0.174375518661222,1.,-1.90335253863003));
#30739=CARTESIAN_POINT('Ctrl Pts',(0.173776635257984,1.,-1.90911693975475));
#30740=CARTESIAN_POINT('Ctrl Pts',(0.173090695383619,1.,-1.91511429159681));
#30741=CARTESIAN_POINT('Ctrl Pts',(0.172321621259557,1.,-1.92122334398034));
#30742=CARTESIAN_POINT('Ctrl Pts',(0.17147119153296,1.,-1.92731093582));
#30743=CARTESIAN_POINT('Ctrl Pts',(0.170541253116136,1.,-1.93329183155455));
#30744=CARTESIAN_POINT('Ctrl Pts',(0.169534904817425,1.,-1.93915639211497));
#30745=CARTESIAN_POINT('Ctrl Pts',(0.168455741607516,1.,-1.94493757756879));
#30746=CARTESIAN_POINT('Ctrl Pts',(0.167307501784469,1.,-1.95069027794286));
#30747=CARTESIAN_POINT('Ctrl Pts',(0.166093592002833,1.,-1.95646759718755));
#30748=CARTESIAN_POINT('Ctrl Pts',(0.1648165689203,1.,-1.96229379940174));
#30749=CARTESIAN_POINT('Ctrl Pts',(0.16347818545776,1.,-1.96816512678));
#30750=CARTESIAN_POINT('Ctrl Pts',(0.162079693556302,1.,-1.97406280235204));
#30751=CARTESIAN_POINT('Ctrl Pts',(0.16062206078461,1.,-1.97996195437557));
#30752=CARTESIAN_POINT('Ctrl Pts',(0.159106226437288,1.,-1.98584238283279));
#30753=CARTESIAN_POINT('Ctrl Pts',(0.157533331459215,1.,-1.99169810931893));
#30754=CARTESIAN_POINT('Ctrl Pts',(0.155904629548774,1.,-1.99753284771487));
#30755=CARTESIAN_POINT('Ctrl Pts',(0.154221403049719,1.,-2.00335565310539));
#30756=CARTESIAN_POINT('Ctrl Pts',(0.152484883621452,1.,-2.00917680318426));
#30757=CARTESIAN_POINT('Ctrl Pts',(0.150696157673084,1.,-2.01500291940243));
#30758=CARTESIAN_POINT('Ctrl Pts',(0.148856124775343,1.,-2.02083464969897));
#30759=CARTESIAN_POINT('Ctrl Pts',(0.146965557332586,1.,-2.02666926182017));
#30760=CARTESIAN_POINT('Ctrl Pts',(0.145025140186058,1.,-2.03250223739941));
#30761=CARTESIAN_POINT('Ctrl Pts',(0.143035515058208,1.,-2.03832911025913));
#30762=CARTESIAN_POINT('Ctrl Pts',(0.140997332152545,1.,-2.04414757947919));
#30763=CARTESIAN_POINT('Ctrl Pts',(0.138911255368966,1.,-2.04995762001333));
#30764=CARTESIAN_POINT('Ctrl Pts',(0.136777941218044,1.,-2.0557604441427));
#30765=CARTESIAN_POINT('Ctrl Pts',(0.134598026192107,1.,-2.06155781517844));
#30766=CARTESIAN_POINT('Ctrl Pts',(0.13237211154771,1.,-2.06735123910319));
#30767=CARTESIAN_POINT('Ctrl Pts',(0.1301007483284,1.,-2.07314114713047));
#30768=CARTESIAN_POINT('Ctrl Pts',(0.127784445276116,1.,-2.07892715110967));
#30769=CARTESIAN_POINT('Ctrl Pts',(0.125423679412058,1.,-2.08470840653628));
#30770=CARTESIAN_POINT('Ctrl Pts',(0.123018905621083,1.,-2.09048392424826));
#30771=CARTESIAN_POINT('Ctrl Pts',(0.120570567965129,1.,-2.09625292867756));
#30772=CARTESIAN_POINT('Ctrl Pts',(0.118079107988368,1.,-2.10201512132945));
#30773=CARTESIAN_POINT('Ctrl Pts',(0.11554495768794,1.,-2.10777050261359));
#30774=CARTESIAN_POINT('Ctrl Pts',(0.112968534419746,1.,-2.11351924490335));
#30775=CARTESIAN_POINT('Ctrl Pts',(0.11035023613502,1.,-2.11926155590849));
#30776=CARTESIAN_POINT('Ctrl Pts',(0.107690435231068,1.,-2.12499752306927));
#30777=CARTESIAN_POINT('Ctrl Pts',(0.104989479152703,1.,-2.1307270488718));
#30778=CARTESIAN_POINT('Ctrl Pts',(0.102247700556064,1.,-2.13644992667052));
#30779=CARTESIAN_POINT('Ctrl Pts',(0.0994654261990743,1.,-2.14216588395974));
#30780=CARTESIAN_POINT('Ctrl Pts',(0.0966429852305689,1.,-2.14787463531864));
#30781=CARTESIAN_POINT('Ctrl Pts',(0.0937807218868345,1.,-2.15357593978377));
#30782=CARTESIAN_POINT('Ctrl Pts',(0.0908789888108266,1.,-2.15926961544808));
#30783=CARTESIAN_POINT('Ctrl Pts',(0.0879381291387823,1.,-2.16495552645275));
#30784=CARTESIAN_POINT('Ctrl Pts',(0.0849584620835643,1.,-2.17063357871031));
#30785=CARTESIAN_POINT('Ctrl Pts',(0.0819402680871939,1.,-2.1763037121106));
#30786=CARTESIAN_POINT('Ctrl Pts',(0.0788837727683228,1.,-2.18196589448304));
#30787=CARTESIAN_POINT('Ctrl Pts',(0.0757891465833411,1.,-2.1876201139874));
#30788=CARTESIAN_POINT('Ctrl Pts',(0.0732830357304276,1.,-2.19213712012956));
#30789=CARTESIAN_POINT('Ctrl Pts',(0.0713863779524627,1.,-2.19552129483562));
#30790=CARTESIAN_POINT('Ctrl Pts',(0.0701143536324926,1.,-2.19777582085261));
#30791=CARTESIAN_POINT('Ctrl Pts',(0.0694764450219584,1.,-2.19890268624765));
#30792=CARTESIAN_POINT('',(0.163289472382896,0.,-1.74236521665491));
#30793=CARTESIAN_POINT('Origin',(0.,0.,0.));
#30794=CARTESIAN_POINT('',(0.383122945602004,1.,-1.7075470150345));
#30795=CARTESIAN_POINT('Origin',(0.,1.,0.));
#30796=CARTESIAN_POINT('',(0.383122945602004,0.,-1.7075470150345));
#30797=CARTESIAN_POINT('Ctrl Pts',(0.61342227326009,-1.,-2.11275013067528));
#30798=CARTESIAN_POINT('Ctrl Pts',(0.61342227326009,1.,-2.11275013067528));
#30799=CARTESIAN_POINT('Ctrl Pts',(0.61246736556225,-1.,-2.11187554260142));
#30800=CARTESIAN_POINT('Ctrl Pts',(0.61246736556225,1.,-2.11187554260142));
#30801=CARTESIAN_POINT('Ctrl Pts',(0.610560911691113,-1.,-2.11012443807661));
#30802=CARTESIAN_POINT('Ctrl Pts',(0.610560911691113,1.,-2.11012443807661));
#30803=CARTESIAN_POINT('Ctrl Pts',(0.607711315456826,-1.,-2.10749199615859));
#30804=CARTESIAN_POINT('Ctrl Pts',(0.607711315456826,1.,-2.10749199615859));
#30805=CARTESIAN_POINT('Ctrl Pts',(0.603932030738212,-1.,-2.10397049887709));
#30806=CARTESIAN_POINT('Ctrl Pts',(0.603932030738212,1.,-2.10397049887709));
#30807=CARTESIAN_POINT('Ctrl Pts',(0.599241616422144,-1.,-2.09954930865331));
#30808=CARTESIAN_POINT('Ctrl Pts',(0.599241616422144,1.,-2.09954930865331));
#30809=CARTESIAN_POINT('Ctrl Pts',(0.594585006052823,-1.,-2.09510876220501));
#30810=CARTESIAN_POINT('Ctrl Pts',(0.594585006052823,1.,-2.09510876220501));
#30811=CARTESIAN_POINT('Ctrl Pts',(0.589962365403189,-1.,-2.09064881812053));
#30812=CARTESIAN_POINT('Ctrl Pts',(0.589962365403189,1.,-2.09064881812053));
#30813=CARTESIAN_POINT('Ctrl Pts',(0.585373918990895,-1.,-2.086169437277));
#30814=CARTESIAN_POINT('Ctrl Pts',(0.585373918990895,1.,-2.086169437277));
#30815=CARTESIAN_POINT('Ctrl Pts',(0.580819952107256,-1.,-2.08167059018138));
#30816=CARTESIAN_POINT('Ctrl Pts',(0.580819952107256,1.,-2.08167059018138));
#30817=CARTESIAN_POINT('Ctrl Pts',(0.576300797416274,-1.,-2.07715226767361));
#30818=CARTESIAN_POINT('Ctrl Pts',(0.576300797416274,1.,-2.07715226767361));
#30819=CARTESIAN_POINT('Ctrl Pts',(0.571816823242411,-1.,-2.07261449292758));
#30820=CARTESIAN_POINT('Ctrl Pts',(0.571816823242411,1.,-2.07261449292758));
#30821=CARTESIAN_POINT('Ctrl Pts',(0.567368421181229,-1.,-2.06805732997383));
#30822=CARTESIAN_POINT('Ctrl Pts',(0.567368421181229,1.,-2.06805732997383));
#30823=CARTESIAN_POINT('Ctrl Pts',(0.562955993082574,-1.,-2.06348090160697));
#30824=CARTESIAN_POINT('Ctrl Pts',(0.562955993082574,1.,-2.06348090160697));
#30825=CARTESIAN_POINT('Ctrl Pts',(0.558579940185467,-1.,-2.05888537756571));
#30826=CARTESIAN_POINT('Ctrl Pts',(0.558579940185467,1.,-2.05888537756571));
#30827=CARTESIAN_POINT('Ctrl Pts',(0.554240657464109,-1.,-2.05427091604482));
#30828=CARTESIAN_POINT('Ctrl Pts',(0.554240657464109,1.,-2.05427091604482));
#30829=CARTESIAN_POINT('Ctrl Pts',(0.549938525150342,-1.,-2.04963761077974));
#30830=CARTESIAN_POINT('Ctrl Pts',(0.549938525150342,1.,-2.04963761077974));
#30831=CARTESIAN_POINT('Ctrl Pts',(0.545673903817348,-1.,-2.0449854471456));
#30832=CARTESIAN_POINT('Ctrl Pts',(0.545673903817348,1.,-2.0449854471456));
#30833=CARTESIAN_POINT('Ctrl Pts',(0.54144712061552,-1.,-2.0403142269048));
#30834=CARTESIAN_POINT('Ctrl Pts',(0.54144712061552,1.,-2.0403142269048));
#30835=CARTESIAN_POINT('Ctrl Pts',(0.537258489833134,-1.,-2.03562362953993));
#30836=CARTESIAN_POINT('Ctrl Pts',(0.537258489833134,1.,-2.03562362953993));
#30837=CARTESIAN_POINT('Ctrl Pts',(0.533108355132905,-1.,-2.03091336214401));
#30838=CARTESIAN_POINT('Ctrl Pts',(0.533108355132905,1.,-2.03091336214401));
#30839=CARTESIAN_POINT('Ctrl Pts',(0.52899712724191,-1.,-2.02618329083289));
#30840=CARTESIAN_POINT('Ctrl Pts',(0.52899712724191,1.,-2.02618329083289));
#30841=CARTESIAN_POINT('Ctrl Pts',(0.524925318333518,-1.,-2.02143356304712));
#30842=CARTESIAN_POINT('Ctrl Pts',(0.524925318333518,1.,-2.02143356304712));
#30843=CARTESIAN_POINT('Ctrl Pts',(0.520893590399428,-1.,-2.01666477917306));
#30844=CARTESIAN_POINT('Ctrl Pts',(0.520893590399428,1.,-2.01666477917306));
#30845=CARTESIAN_POINT('Ctrl Pts',(0.516902681728733,-1.,-2.01187773939257));
#30846=CARTESIAN_POINT('Ctrl Pts',(0.516902681728733,1.,-2.01187773939257));
#30847=CARTESIAN_POINT('Ctrl Pts',(0.512953306961813,-1.,-2.00707309946955));
#30848=CARTESIAN_POINT('Ctrl Pts',(0.512953306961813,1.,-2.00707309946955));
#30849=CARTESIAN_POINT('Ctrl Pts',(0.509046069886152,-1.,-2.00225107134733));
#30850=CARTESIAN_POINT('Ctrl Pts',(0.509046069886152,1.,-2.00225107134733));
#30851=CARTESIAN_POINT('Ctrl Pts',(0.505181361323011,-1.,-1.99741107463567));
#30852=CARTESIAN_POINT('Ctrl Pts',(0.505181361323011,1.,-1.99741107463567));
#30853=CARTESIAN_POINT('Ctrl Pts',(0.501359287727129,-1.,-1.9925514912615));
#30854=CARTESIAN_POINT('Ctrl Pts',(0.501359287727129,1.,-1.9925514912615));
#30855=CARTESIAN_POINT('Ctrl Pts',(0.497579909545564,-1.,-1.98767044752929));
#30856=CARTESIAN_POINT('Ctrl Pts',(0.497579909545564,1.,-1.98767044752929));
#30857=CARTESIAN_POINT('Ctrl Pts',(0.493843476541492,-1.,-1.9827665876182));
#30858=CARTESIAN_POINT('Ctrl Pts',(0.493843476541492,1.,-1.9827665876182));
#30859=CARTESIAN_POINT('Ctrl Pts',(0.490150627860955,-1.,-1.97783973019229));
#30860=CARTESIAN_POINT('Ctrl Pts',(0.490150627860955,1.,-1.97783973019229));
#30861=CARTESIAN_POINT('Ctrl Pts',(0.486502692907661,-1.,-1.97289186263272));
#30862=CARTESIAN_POINT('Ctrl Pts',(0.486502692907661,1.,-1.97289186263272));
#30863=CARTESIAN_POINT('Ctrl Pts',(0.482901662120686,-1.,-1.96792703422358));
#30864=CARTESIAN_POINT('Ctrl Pts',(0.482901662120686,1.,-1.96792703422358));
#30865=CARTESIAN_POINT('Ctrl Pts',(0.479349583074846,-1.,-1.96294933055938));
#30866=CARTESIAN_POINT('Ctrl Pts',(0.479349583074846,1.,-1.96294933055938));
#30867=CARTESIAN_POINT('Ctrl Pts',(0.475848034683171,-1.,-1.95796111148175));
#30868=CARTESIAN_POINT('Ctrl Pts',(0.475848034683171,1.,-1.95796111148175));
#30869=CARTESIAN_POINT('Ctrl Pts',(0.472397672264079,-1.,-1.95296148278136));
#30870=CARTESIAN_POINT('Ctrl Pts',(0.472397672264079,1.,-1.95296148278136));
#30871=CARTESIAN_POINT('Ctrl Pts',(0.468997482913158,-1.,-1.94794381136524));
#30872=CARTESIAN_POINT('Ctrl Pts',(0.468997482913158,1.,-1.94794381136524));
#30873=CARTESIAN_POINT('Ctrl Pts',(0.465645462026064,-1.,-1.94289794196205));
#30874=CARTESIAN_POINT('Ctrl Pts',(0.465645462026064,1.,-1.94289794196205));
#30875=CARTESIAN_POINT('Ctrl Pts',(0.462340031009087,-1.,-1.93781486640834));
#30876=CARTESIAN_POINT('Ctrl Pts',(0.462340031009087,1.,-1.93781486640834));
#30877=CARTESIAN_POINT('Ctrl Pts',(0.459081234547931,-1.,-1.93269066517936));
#30878=CARTESIAN_POINT('Ctrl Pts',(0.459081234547931,1.,-1.93269066517936));
#30879=CARTESIAN_POINT('Ctrl Pts',(0.455872005174335,-1.,-1.92753067150461));
#30880=CARTESIAN_POINT('Ctrl Pts',(0.455872005174335,1.,-1.92753067150461));
#30881=CARTESIAN_POINT('Ctrl Pts',(0.452719478359356,-1.,-1.9223538064847));
#30882=CARTESIAN_POINT('Ctrl Pts',(0.452719478359356,1.,-1.9223538064847));
#30883=CARTESIAN_POINT('Ctrl Pts',(0.449632260106572,-1.,-1.91718342555717));
#30884=CARTESIAN_POINT('Ctrl Pts',(0.449632260106572,1.,-1.91718342555717));
#30885=CARTESIAN_POINT('Ctrl Pts',(0.446617343485651,-1.,-1.91203699981095));
#30886=CARTESIAN_POINT('Ctrl Pts',(0.446617343485651,1.,-1.91203699981095));
#30887=CARTESIAN_POINT('Ctrl Pts',(0.44367755684917,-1.,-1.90691756144906));
#30888=CARTESIAN_POINT('Ctrl Pts',(0.44367755684917,1.,-1.90691756144906));
#30889=CARTESIAN_POINT('Ctrl Pts',(0.44080783370416,-1.,-1.90180124389137));
#30890=CARTESIAN_POINT('Ctrl Pts',(0.44080783370416,1.,-1.90180124389137));
#30891=CARTESIAN_POINT('Ctrl Pts',(0.437995003948443,-1.,-1.89663648956549));
#30892=CARTESIAN_POINT('Ctrl Pts',(0.437995003948443,1.,-1.89663648956549));
#30893=CARTESIAN_POINT('Ctrl Pts',(0.43522566096358,-1.,-1.89136993975585));
#30894=CARTESIAN_POINT('Ctrl Pts',(0.43522566096358,1.,-1.89136993975585));
#30895=CARTESIAN_POINT('Ctrl Pts',(0.432493038548833,-1.,-1.88596913666828));
#30896=CARTESIAN_POINT('Ctrl Pts',(0.432493038548833,1.,-1.88596913666828));
#30897=CARTESIAN_POINT('Ctrl Pts',(0.429803062482217,-1.,-1.88044229001779));
#30898=CARTESIAN_POINT('Ctrl Pts',(0.429803062482217,1.,-1.88044229001779));
#30899=CARTESIAN_POINT('Ctrl Pts',(0.427183828518743,-1.,-1.87486989291334));
#30900=CARTESIAN_POINT('Ctrl Pts',(0.427183828518743,1.,-1.87486989291334));
#30901=CARTESIAN_POINT('Ctrl Pts',(0.424678177290876,-1.,-1.8693780394412));
#30902=CARTESIAN_POINT('Ctrl Pts',(0.424678177290876,1.,-1.8693780394412));
#30903=CARTESIAN_POINT('Ctrl Pts',(0.422327307417884,-1.,-1.86408083333863));
#30904=CARTESIAN_POINT('Ctrl Pts',(0.422327307417884,1.,-1.86408083333863));
#30905=CARTESIAN_POINT('Ctrl Pts',(0.420157287975583,-1.,-1.8590328109667));
#30906=CARTESIAN_POINT('Ctrl Pts',(0.420157287975583,1.,-1.8590328109667));
#30907=CARTESIAN_POINT('Ctrl Pts',(0.418164129144045,-1.,-1.8541763285645));
#30908=CARTESIAN_POINT('Ctrl Pts',(0.418164129144045,1.,-1.8541763285645));
#30909=CARTESIAN_POINT('Ctrl Pts',(0.416300022039885,-1.,-1.84929312930314));
#30910=CARTESIAN_POINT('Ctrl Pts',(0.416300022039885,1.,-1.84929312930314));
#30911=CARTESIAN_POINT('Ctrl Pts',(0.414487438255542,-1.,-1.84405757074218));
#30912=CARTESIAN_POINT('Ctrl Pts',(0.414487438255542,1.,-1.84405757074218));
#30913=CARTESIAN_POINT('Ctrl Pts',(0.412633125322945,-1.,-1.8380895347617));
#30914=CARTESIAN_POINT('Ctrl Pts',(0.412633125322945,1.,-1.8380895347617));
#30915=CARTESIAN_POINT('Ctrl Pts',(0.410641256301276,-1.,-1.83100408895047));
#30916=CARTESIAN_POINT('Ctrl Pts',(0.410641256301276,1.,-1.83100408895047));
#30917=CARTESIAN_POINT('Ctrl Pts',(0.408428948106227,-1.,-1.82247022677562));
#30918=CARTESIAN_POINT('Ctrl Pts',(0.408428948106227,1.,-1.82247022677562));
#30919=CARTESIAN_POINT('Ctrl Pts',(0.405933518407175,-1.,-1.81223801812013));
#30920=CARTESIAN_POINT('Ctrl Pts',(0.405933518407175,1.,-1.81223801812013));
#30921=CARTESIAN_POINT('Ctrl Pts',(0.403107976163396,-1.,-1.80012077173238));
#30922=CARTESIAN_POINT('Ctrl Pts',(0.403107976163396,1.,-1.80012077173238));
#30923=CARTESIAN_POINT('Ctrl Pts',(0.399919403774155,-1.,-1.78598826343754));
#30924=CARTESIAN_POINT('Ctrl Pts',(0.399919403774155,1.,-1.78598826343754));
#30925=CARTESIAN_POINT('Ctrl Pts',(0.396346196110688,-1.,-1.76975560043442));
#30926=CARTESIAN_POINT('Ctrl Pts',(0.396346196110688,1.,-1.76975560043442));
#30927=CARTESIAN_POINT('Ctrl Pts',(0.392375812285395,-1.,-1.75137405310193));
#30928=CARTESIAN_POINT('Ctrl Pts',(0.392375812285395,1.,-1.75137405310193));
#30929=CARTESIAN_POINT('Ctrl Pts',(0.388877023502615,-1.,-1.73493170972829));
#30930=CARTESIAN_POINT('Ctrl Pts',(0.388877023502615,1.,-1.73493170972829));
#30931=CARTESIAN_POINT('Ctrl Pts',(0.386070790323281,-1.,-1.72162022244582));
#30932=CARTESIAN_POINT('Ctrl Pts',(0.386070790323281,1.,-1.72162022244582));
#30933=CARTESIAN_POINT('Ctrl Pts',(0.384119047314215,-1.,-1.71231062891398));
#30934=CARTESIAN_POINT('Ctrl Pts',(0.384119047314215,1.,-1.71231062891398));
#30935=CARTESIAN_POINT('Ctrl Pts',(0.383122945602004,-1.,-1.7075470150345));
#30936=CARTESIAN_POINT('Ctrl Pts',(0.383122945602004,1.,-1.7075470150345));
#30937=CARTESIAN_POINT('',(0.61342227326009,1.,-2.11275013067528));
#30938=CARTESIAN_POINT('Ctrl Pts',(0.61342227326009,1.,-2.11275013067528));
#30939=CARTESIAN_POINT('Ctrl Pts',(0.61246736556225,1.,-2.11187554260142));
#30940=CARTESIAN_POINT('Ctrl Pts',(0.610560911691113,1.,-2.11012443807661));
#30941=CARTESIAN_POINT('Ctrl Pts',(0.607711315456826,1.,-2.10749199615859));
#30942=CARTESIAN_POINT('Ctrl Pts',(0.603932030738212,1.,-2.10397049887709));
#30943=CARTESIAN_POINT('Ctrl Pts',(0.599241616422144,1.,-2.09954930865331));
#30944=CARTESIAN_POINT('Ctrl Pts',(0.594585006052823,1.,-2.09510876220501));
#30945=CARTESIAN_POINT('Ctrl Pts',(0.589962365403189,1.,-2.09064881812053));
#30946=CARTESIAN_POINT('Ctrl Pts',(0.585373918990895,1.,-2.086169437277));
#30947=CARTESIAN_POINT('Ctrl Pts',(0.580819952107256,1.,-2.08167059018138));
#30948=CARTESIAN_POINT('Ctrl Pts',(0.576300797416274,1.,-2.07715226767361));
#30949=CARTESIAN_POINT('Ctrl Pts',(0.571816823242411,1.,-2.07261449292758));
#30950=CARTESIAN_POINT('Ctrl Pts',(0.567368421181229,1.,-2.06805732997383));
#30951=CARTESIAN_POINT('Ctrl Pts',(0.562955993082574,1.,-2.06348090160697));
#30952=CARTESIAN_POINT('Ctrl Pts',(0.558579940185467,1.,-2.05888537756571));
#30953=CARTESIAN_POINT('Ctrl Pts',(0.554240657464109,1.,-2.05427091604482));
#30954=CARTESIAN_POINT('Ctrl Pts',(0.549938525150342,1.,-2.04963761077974));
#30955=CARTESIAN_POINT('Ctrl Pts',(0.545673903817348,1.,-2.0449854471456));
#30956=CARTESIAN_POINT('Ctrl Pts',(0.54144712061552,1.,-2.0403142269048));
#30957=CARTESIAN_POINT('Ctrl Pts',(0.537258489833134,1.,-2.03562362953993));
#30958=CARTESIAN_POINT('Ctrl Pts',(0.533108355132905,1.,-2.03091336214401));
#30959=CARTESIAN_POINT('Ctrl Pts',(0.52899712724191,1.,-2.02618329083289));
#30960=CARTESIAN_POINT('Ctrl Pts',(0.524925318333518,1.,-2.02143356304712));
#30961=CARTESIAN_POINT('Ctrl Pts',(0.520893590399428,1.,-2.01666477917306));
#30962=CARTESIAN_POINT('Ctrl Pts',(0.516902681728733,1.,-2.01187773939257));
#30963=CARTESIAN_POINT('Ctrl Pts',(0.512953306961813,1.,-2.00707309946955));
#30964=CARTESIAN_POINT('Ctrl Pts',(0.509046069886152,1.,-2.00225107134733));
#30965=CARTESIAN_POINT('Ctrl Pts',(0.505181361323011,1.,-1.99741107463567));
#30966=CARTESIAN_POINT('Ctrl Pts',(0.501359287727129,1.,-1.9925514912615));
#30967=CARTESIAN_POINT('Ctrl Pts',(0.497579909545564,1.,-1.98767044752929));
#30968=CARTESIAN_POINT('Ctrl Pts',(0.493843476541492,1.,-1.9827665876182));
#30969=CARTESIAN_POINT('Ctrl Pts',(0.490150627860955,1.,-1.97783973019229));
#30970=CARTESIAN_POINT('Ctrl Pts',(0.486502692907661,1.,-1.97289186263272));
#30971=CARTESIAN_POINT('Ctrl Pts',(0.482901662120686,1.,-1.96792703422358));
#30972=CARTESIAN_POINT('Ctrl Pts',(0.479349583074846,1.,-1.96294933055938));
#30973=CARTESIAN_POINT('Ctrl Pts',(0.475848034683171,1.,-1.95796111148175));
#30974=CARTESIAN_POINT('Ctrl Pts',(0.472397672264079,1.,-1.95296148278136));
#30975=CARTESIAN_POINT('Ctrl Pts',(0.468997482913158,1.,-1.94794381136524));
#30976=CARTESIAN_POINT('Ctrl Pts',(0.465645462026064,1.,-1.94289794196205));
#30977=CARTESIAN_POINT('Ctrl Pts',(0.462340031009087,1.,-1.93781486640834));
#30978=CARTESIAN_POINT('Ctrl Pts',(0.459081234547931,1.,-1.93269066517936));
#30979=CARTESIAN_POINT('Ctrl Pts',(0.455872005174335,1.,-1.92753067150461));
#30980=CARTESIAN_POINT('Ctrl Pts',(0.452719478359356,1.,-1.9223538064847));
#30981=CARTESIAN_POINT('Ctrl Pts',(0.449632260106572,1.,-1.91718342555717));
#30982=CARTESIAN_POINT('Ctrl Pts',(0.446617343485651,1.,-1.91203699981095));
#30983=CARTESIAN_POINT('Ctrl Pts',(0.44367755684917,1.,-1.90691756144906));
#30984=CARTESIAN_POINT('Ctrl Pts',(0.44080783370416,1.,-1.90180124389137));
#30985=CARTESIAN_POINT('Ctrl Pts',(0.437995003948443,1.,-1.89663648956549));
#30986=CARTESIAN_POINT('Ctrl Pts',(0.43522566096358,1.,-1.89136993975585));
#30987=CARTESIAN_POINT('Ctrl Pts',(0.432493038548833,1.,-1.88596913666828));
#30988=CARTESIAN_POINT('Ctrl Pts',(0.429803062482217,1.,-1.88044229001779));
#30989=CARTESIAN_POINT('Ctrl Pts',(0.427183828518743,1.,-1.87486989291334));
#30990=CARTESIAN_POINT('Ctrl Pts',(0.424678177290876,1.,-1.8693780394412));
#30991=CARTESIAN_POINT('Ctrl Pts',(0.422327307417884,1.,-1.86408083333863));
#30992=CARTESIAN_POINT('Ctrl Pts',(0.420157287975583,1.,-1.8590328109667));
#30993=CARTESIAN_POINT('Ctrl Pts',(0.418164129144045,1.,-1.8541763285645));
#30994=CARTESIAN_POINT('Ctrl Pts',(0.416300022039885,1.,-1.84929312930314));
#30995=CARTESIAN_POINT('Ctrl Pts',(0.414487438255542,1.,-1.84405757074218));
#30996=CARTESIAN_POINT('Ctrl Pts',(0.412633125322945,1.,-1.8380895347617));
#30997=CARTESIAN_POINT('Ctrl Pts',(0.410641256301276,1.,-1.83100408895047));
#30998=CARTESIAN_POINT('Ctrl Pts',(0.408428948106227,1.,-1.82247022677562));
#30999=CARTESIAN_POINT('Ctrl Pts',(0.405933518407175,1.,-1.81223801812013));
#31000=CARTESIAN_POINT('Ctrl Pts',(0.403107976163396,1.,-1.80012077173238));
#31001=CARTESIAN_POINT('Ctrl Pts',(0.399919403774155,1.,-1.78598826343754));
#31002=CARTESIAN_POINT('Ctrl Pts',(0.396346196110688,1.,-1.76975560043442));
#31003=CARTESIAN_POINT('Ctrl Pts',(0.392375812285395,1.,-1.75137405310193));
#31004=CARTESIAN_POINT('Ctrl Pts',(0.388877023502615,1.,-1.73493170972829));
#31005=CARTESIAN_POINT('Ctrl Pts',(0.386070790323281,1.,-1.72162022244582));
#31006=CARTESIAN_POINT('Ctrl Pts',(0.384119047314215,1.,-1.71231062891398));
#31007=CARTESIAN_POINT('Ctrl Pts',(0.383122945602004,1.,-1.7075470150345));
#31008=CARTESIAN_POINT('',(0.61342227326009,0.,-2.11275013067528));
#31009=CARTESIAN_POINT('Origin',(0.745574324794401,0.,-2.0698113262342));
#31010=CARTESIAN_POINT('',(0.745574324794401,1.,-2.0698113262342));
#31011=CARTESIAN_POINT('',(0.61342227326009,1.,-2.11275013067528));
#31012=CARTESIAN_POINT('',(0.745574324794401,0.,-2.0698113262342));
#31013=CARTESIAN_POINT('Ctrl Pts',(0.693717979106306,-1.,-1.60662857109684));
#31014=CARTESIAN_POINT('Ctrl Pts',(0.693717979106306,1.,-1.60662857109684));
#31015=CARTESIAN_POINT('Ctrl Pts',(0.695712097881194,-1.,-1.61106790958151));
#31016=CARTESIAN_POINT('Ctrl Pts',(0.695712097881194,1.,-1.61106790958151));
#31017=CARTESIAN_POINT('Ctrl Pts',(0.699605146405088,-1.,-1.61974673472612));
#31018=CARTESIAN_POINT('Ctrl Pts',(0.699605146405088,1.,-1.61974673472612));
#31019=CARTESIAN_POINT('Ctrl Pts',(0.705159151988319,-1.,-1.63216541664676));
#31020=CARTESIAN_POINT('Ctrl Pts',(0.705159151988319,1.,-1.63216541664676));
#31021=CARTESIAN_POINT('Ctrl Pts',(0.711993139355394,-1.,-1.64752408832016));
#31022=CARTESIAN_POINT('Ctrl Pts',(0.711993139355394,1.,-1.64752408832016));
#31023=CARTESIAN_POINT('Ctrl Pts',(0.719585433804282,-1.,-1.6647288055568));
#31024=CARTESIAN_POINT('Ctrl Pts',(0.719585433804282,1.,-1.6647288055568));
#31025=CARTESIAN_POINT('Ctrl Pts',(0.726235967997433,-1.,-1.67996158455503));
#31026=CARTESIAN_POINT('Ctrl Pts',(0.726235967997433,1.,-1.67996158455503));
#31027=CARTESIAN_POINT('Ctrl Pts',(0.731963238697195,-1.,-1.69326921975743));
#31028=CARTESIAN_POINT('Ctrl Pts',(0.731963238697195,1.,-1.69326921975743));
#31029=CARTESIAN_POINT('Ctrl Pts',(0.736799665724771,-1.,-1.70473309006121));
#31030=CARTESIAN_POINT('Ctrl Pts',(0.736799665724771,1.,-1.70473309006121));
#31031=CARTESIAN_POINT('Ctrl Pts',(0.740795162032087,-1.,-1.71447789751927));
#31032=CARTESIAN_POINT('Ctrl Pts',(0.740795162032087,1.,-1.71447789751927));
#31033=CARTESIAN_POINT('Ctrl Pts',(0.744021445433764,-1.,-1.7226822991693));
#31034=CARTESIAN_POINT('Ctrl Pts',(0.744021445433764,1.,-1.7226822991693));
#31035=CARTESIAN_POINT('Ctrl Pts',(0.746574710096436,-1.,-1.72958533647399));
#31036=CARTESIAN_POINT('Ctrl Pts',(0.746574710096436,1.,-1.72958533647399));
#31037=CARTESIAN_POINT('Ctrl Pts',(0.748582462954854,-1.,-1.73550351679848));
#31038=CARTESIAN_POINT('Ctrl Pts',(0.748582462954854,1.,-1.73550351679848));
#31039=CARTESIAN_POINT('Ctrl Pts',(0.75019343597954,-1.,-1.74080458266705));
#31040=CARTESIAN_POINT('Ctrl Pts',(0.75019343597954,1.,-1.74080458266705));
#31041=CARTESIAN_POINT('Ctrl Pts',(0.751555614163629,-1.,-1.74585086852298));
#31042=CARTESIAN_POINT('Ctrl Pts',(0.751555614163629,1.,-1.74585086852298));
#31043=CARTESIAN_POINT('Ctrl Pts',(0.752797683531377,-1.,-1.75095139468809));
#31044=CARTESIAN_POINT('Ctrl Pts',(0.752797683531377,1.,-1.75095139468809));
#31045=CARTESIAN_POINT('Ctrl Pts',(0.75400925402848,-1.,-1.75631083600175));
#31046=CARTESIAN_POINT('Ctrl Pts',(0.75400925402848,1.,-1.75631083600175));
#31047=CARTESIAN_POINT('Ctrl Pts',(0.755220979975262,-1.,-1.7619781724032));
#31048=CARTESIAN_POINT('Ctrl Pts',(0.755220979975262,1.,-1.7619781724032));
#31049=CARTESIAN_POINT('Ctrl Pts',(0.756421896028403,-1.,-1.76789396003141));
#31050=CARTESIAN_POINT('Ctrl Pts',(0.756421896028403,1.,-1.76789396003141));
#31051=CARTESIAN_POINT('Ctrl Pts',(0.757578264077238,-1.,-1.77394167108342));
#31052=CARTESIAN_POINT('Ctrl Pts',(0.757578264077238,1.,-1.77394167108342));
#31053=CARTESIAN_POINT('Ctrl Pts',(0.75865062667738,-1.,-1.77999411220912));
#31054=CARTESIAN_POINT('Ctrl Pts',(0.75865062667738,1.,-1.77999411220912));
#31055=CARTESIAN_POINT('Ctrl Pts',(0.759614401109868,-1.,-1.78596964884527));
#31056=CARTESIAN_POINT('Ctrl Pts',(0.759614401109868,1.,-1.78596964884527));
#31057=CARTESIAN_POINT('Ctrl Pts',(0.760469555880425,-1.,-1.79185815610802));
#31058=CARTESIAN_POINT('Ctrl Pts',(0.760469555880425,1.,-1.79185815610802));
#31059=CARTESIAN_POINT('Ctrl Pts',(0.761229695230359,-1.,-1.79768986997735));
#31060=CARTESIAN_POINT('Ctrl Pts',(0.761229695230359,1.,-1.79768986997735));
#31061=CARTESIAN_POINT('Ctrl Pts',(0.761915336443515,-1.,-1.80351583877334));
#31062=CARTESIAN_POINT('Ctrl Pts',(0.761915336443515,1.,-1.80351583877334));
#31063=CARTESIAN_POINT('Ctrl Pts',(0.762546129464036,-1.,-1.80938551463989));
#31064=CARTESIAN_POINT('Ctrl Pts',(0.762546129464036,1.,-1.80938551463989));
#31065=CARTESIAN_POINT('Ctrl Pts',(0.763132003836783,-1.,-1.81532118405566));
#31066=CARTESIAN_POINT('Ctrl Pts',(0.763132003836783,1.,-1.81532118405566));
#31067=CARTESIAN_POINT('Ctrl Pts',(0.763673465462854,-1.,-1.82131873145297));
#31068=CARTESIAN_POINT('Ctrl Pts',(0.763673465462854,1.,-1.82131873145297));
#31069=CARTESIAN_POINT('Ctrl Pts',(0.764165902606055,-1.,-1.8273599120008));
#31070=CARTESIAN_POINT('Ctrl Pts',(0.764165902606055,1.,-1.8273599120008));
#31071=CARTESIAN_POINT('Ctrl Pts',(0.764602549687845,-1.,-1.8334207722714));
#31072=CARTESIAN_POINT('Ctrl Pts',(0.764602549687845,1.,-1.8334207722714));
#31073=CARTESIAN_POINT('Ctrl Pts',(0.764978057881687,-1.,-1.83948181064823));
#31074=CARTESIAN_POINT('Ctrl Pts',(0.764978057881687,1.,-1.83948181064823));
#31075=CARTESIAN_POINT('Ctrl Pts',(0.765291664861971,-1.,-1.84553698875911));
#31076=CARTESIAN_POINT('Ctrl Pts',(0.765291664861971,1.,-1.84553698875911));
#31077=CARTESIAN_POINT('Ctrl Pts',(0.765545710619023,-1.,-1.85158945130054));
#31078=CARTESIAN_POINT('Ctrl Pts',(0.765545710619023,1.,-1.85158945130054));
#31079=CARTESIAN_POINT('Ctrl Pts',(0.765744212909305,-1.,-1.85764741390391));
#31080=CARTESIAN_POINT('Ctrl Pts',(0.765744212909305,1.,-1.85764741390391));
#31081=CARTESIAN_POINT('Ctrl Pts',(0.765891519092557,-1.,-1.86372027063315));
#31082=CARTESIAN_POINT('Ctrl Pts',(0.765891519092557,1.,-1.86372027063315));
#31083=CARTESIAN_POINT('Ctrl Pts',(0.765990708546111,-1.,-1.86981398314345));
#31084=CARTESIAN_POINT('Ctrl Pts',(0.765990708546111,1.,-1.86981398314345));
#31085=CARTESIAN_POINT('Ctrl Pts',(0.766042837036759,-1.,-1.87592888967886));
#31086=CARTESIAN_POINT('Ctrl Pts',(0.766042837036759,1.,-1.87592888967886));
#31087=CARTESIAN_POINT('Ctrl Pts',(0.766047794851868,-1.,-1.88206215302561));
#31088=CARTESIAN_POINT('Ctrl Pts',(0.766047794851868,1.,-1.88206215302561));
#31089=CARTESIAN_POINT('Ctrl Pts',(0.76600483706209,-1.,-1.88820926433409));
#31090=CARTESIAN_POINT('Ctrl Pts',(0.76600483706209,1.,-1.88820926433409));
#31091=CARTESIAN_POINT('Ctrl Pts',(0.765913193856979,-1.,-1.89436577771389));
#31092=CARTESIAN_POINT('Ctrl Pts',(0.765913193856979,1.,-1.89436577771389));
#31093=CARTESIAN_POINT('Ctrl Pts',(0.765772772593395,-1.,-1.90052930393599));
#31094=CARTESIAN_POINT('Ctrl Pts',(0.765772772593395,1.,-1.90052930393599));
#31095=CARTESIAN_POINT('Ctrl Pts',(0.765584196937936,-1.,-1.90669961402362));
#31096=CARTESIAN_POINT('Ctrl Pts',(0.765584196937936,1.,-1.90669961402362));
#31097=CARTESIAN_POINT('Ctrl Pts',(0.765348465884739,-1.,-1.91287765805174));
#31098=CARTESIAN_POINT('Ctrl Pts',(0.765348465884739,1.,-1.91287765805174));
#31099=CARTESIAN_POINT('Ctrl Pts',(0.765066729667095,-1.,-1.91906491634197));
#31100=CARTESIAN_POINT('Ctrl Pts',(0.765066729667095,1.,-1.91906491634197));
#31101=CARTESIAN_POINT('Ctrl Pts',(0.764740025488189,-1.,-1.92526263537041));
#31102=CARTESIAN_POINT('Ctrl Pts',(0.764740025488189,1.,-1.92526263537041));
#31103=CARTESIAN_POINT('Ctrl Pts',(0.764369010673889,-1.,-1.93147105496367));
#31104=CARTESIAN_POINT('Ctrl Pts',(0.764369010673889,1.,-1.93147105496367));
#31105=CARTESIAN_POINT('Ctrl Pts',(0.763954049121393,-1.,-1.93768964875867));
#31106=CARTESIAN_POINT('Ctrl Pts',(0.763954049121393,1.,-1.93768964875867));
#31107=CARTESIAN_POINT('Ctrl Pts',(0.76349533353858,-1.,-1.94391746617626));
#31108=CARTESIAN_POINT('Ctrl Pts',(0.76349533353858,1.,-1.94391746617626));
#31109=CARTESIAN_POINT('Ctrl Pts',(0.762992990878774,-1.,-1.95015342590025));
#31110=CARTESIAN_POINT('Ctrl Pts',(0.762992990878774,1.,-1.95015342590025));
#31111=CARTESIAN_POINT('Ctrl Pts',(0.762447203806263,-1.,-1.95639665309893));
#31112=CARTESIAN_POINT('Ctrl Pts',(0.762447203806263,1.,-1.95639665309893));
#31113=CARTESIAN_POINT('Ctrl Pts',(0.761858300014575,-1.,-1.96264672744229));
#31114=CARTESIAN_POINT('Ctrl Pts',(0.761858300014575,1.,-1.96264672744229));
#31115=CARTESIAN_POINT('Ctrl Pts',(0.761226690483986,-1.,-1.96890351582545));
#31116=CARTESIAN_POINT('Ctrl Pts',(0.761226690483986,1.,-1.96890351582545));
#31117=CARTESIAN_POINT('Ctrl Pts',(0.760552825409855,-1.,-1.97516705321521));
#31118=CARTESIAN_POINT('Ctrl Pts',(0.760552825409855,1.,-1.97516705321521));
#31119=CARTESIAN_POINT('Ctrl Pts',(0.759837147452135,-1.,-1.98143741418156));
#31120=CARTESIAN_POINT('Ctrl Pts',(0.759837147452135,1.,-1.98143741418156));
#31121=CARTESIAN_POINT('Ctrl Pts',(0.759080037802242,-1.,-1.98771456680806));
#31122=CARTESIAN_POINT('Ctrl Pts',(0.759080037802242,1.,-1.98771456680806));
#31123=CARTESIAN_POINT('Ctrl Pts',(0.758281796766377,-1.,-1.9939983109871));
#31124=CARTESIAN_POINT('Ctrl Pts',(0.758281796766377,1.,-1.9939983109871));
#31125=CARTESIAN_POINT('Ctrl Pts',(0.757442676862341,-1.,-2.00028834739072));
#31126=CARTESIAN_POINT('Ctrl Pts',(0.757442676862341,1.,-2.00028834739072));
#31127=CARTESIAN_POINT('Ctrl Pts',(0.756562904646496,-1.,-2.00658431587682));
#31128=CARTESIAN_POINT('Ctrl Pts',(0.756562904646496,1.,-2.00658431587682));
#31129=CARTESIAN_POINT('Ctrl Pts',(0.7556427049581,-1.,-2.01288584328149));
#31130=CARTESIAN_POINT('Ctrl Pts',(0.7556427049581,1.,-2.01288584328149));
#31131=CARTESIAN_POINT('Ctrl Pts',(0.75468233072352,-1.,-2.01919259406003));
#31132=CARTESIAN_POINT('Ctrl Pts',(0.75468233072352,1.,-2.01919259406003));
#31133=CARTESIAN_POINT('Ctrl Pts',(0.753682061113765,-1.,-2.02550428623587));
#31134=CARTESIAN_POINT('Ctrl Pts',(0.753682061113765,1.,-2.02550428623587));
#31135=CARTESIAN_POINT('Ctrl Pts',(0.752642180488104,-1.,-2.03182068456467));
#31136=CARTESIAN_POINT('Ctrl Pts',(0.752642180488104,1.,-2.03182068456467));
#31137=CARTESIAN_POINT('Ctrl Pts',(0.751562963361383,-1.,-2.03814160092173));
#31138=CARTESIAN_POINT('Ctrl Pts',(0.751562963361383,1.,-2.03814160092173));
#31139=CARTESIAN_POINT('Ctrl Pts',(0.750444657874758,-1.,-2.04446689147754));
#31140=CARTESIAN_POINT('Ctrl Pts',(0.750444657874758,1.,-2.04446689147754));
#31141=CARTESIAN_POINT('Ctrl Pts',(0.749287468663053,-1.,-2.05079645591606));
#31142=CARTESIAN_POINT('Ctrl Pts',(0.749287468663053,1.,-2.05079645591606));
#31143=CARTESIAN_POINT('Ctrl Pts',(0.748091554181101,-1.,-2.05713023030263));
#31144=CARTESIAN_POINT('Ctrl Pts',(0.748091554181101,1.,-2.05713023030263));
#31145=CARTESIAN_POINT('Ctrl Pts',(0.747103932785504,-1.,-2.06220058927162));
#31146=CARTESIAN_POINT('Ctrl Pts',(0.747103932785504,1.,-2.06220058927162));
#31147=CARTESIAN_POINT('Ctrl Pts',(0.746345871542695,-1.,-2.06600523016401));
#31148=CARTESIAN_POINT('Ctrl Pts',(0.746345871542695,1.,-2.06600523016401));
#31149=CARTESIAN_POINT('Ctrl Pts',(0.74583279137781,-1.,-2.06854248895575));
#31150=CARTESIAN_POINT('Ctrl Pts',(0.74583279137781,1.,-2.06854248895575));
#31151=CARTESIAN_POINT('Ctrl Pts',(0.745574324794401,-1.,-2.0698113262342));
#31152=CARTESIAN_POINT('Ctrl Pts',(0.745574324794401,1.,-2.0698113262342));
#31153=CARTESIAN_POINT('',(0.693717979106306,1.,-1.60662857109684));
#31154=CARTESIAN_POINT('Ctrl Pts',(0.693717979106306,1.,-1.60662857109684));
#31155=CARTESIAN_POINT('Ctrl Pts',(0.695712097881194,1.,-1.61106790958151));
#31156=CARTESIAN_POINT('Ctrl Pts',(0.699605146405088,1.,-1.61974673472612));
#31157=CARTESIAN_POINT('Ctrl Pts',(0.705159151988319,1.,-1.63216541664676));
#31158=CARTESIAN_POINT('Ctrl Pts',(0.711993139355394,1.,-1.64752408832016));
#31159=CARTESIAN_POINT('Ctrl Pts',(0.719585433804282,1.,-1.6647288055568));
#31160=CARTESIAN_POINT('Ctrl Pts',(0.726235967997433,1.,-1.67996158455503));
#31161=CARTESIAN_POINT('Ctrl Pts',(0.731963238697195,1.,-1.69326921975743));
#31162=CARTESIAN_POINT('Ctrl Pts',(0.736799665724771,1.,-1.70473309006121));
#31163=CARTESIAN_POINT('Ctrl Pts',(0.740795162032087,1.,-1.71447789751927));
#31164=CARTESIAN_POINT('Ctrl Pts',(0.744021445433764,1.,-1.7226822991693));
#31165=CARTESIAN_POINT('Ctrl Pts',(0.746574710096436,1.,-1.72958533647399));
#31166=CARTESIAN_POINT('Ctrl Pts',(0.748582462954854,1.,-1.73550351679848));
#31167=CARTESIAN_POINT('Ctrl Pts',(0.75019343597954,1.,-1.74080458266705));
#31168=CARTESIAN_POINT('Ctrl Pts',(0.751555614163629,1.,-1.74585086852298));
#31169=CARTESIAN_POINT('Ctrl Pts',(0.752797683531377,1.,-1.75095139468809));
#31170=CARTESIAN_POINT('Ctrl Pts',(0.75400925402848,1.,-1.75631083600175));
#31171=CARTESIAN_POINT('Ctrl Pts',(0.755220979975262,1.,-1.7619781724032));
#31172=CARTESIAN_POINT('Ctrl Pts',(0.756421896028403,1.,-1.76789396003141));
#31173=CARTESIAN_POINT('Ctrl Pts',(0.757578264077238,1.,-1.77394167108342));
#31174=CARTESIAN_POINT('Ctrl Pts',(0.75865062667738,1.,-1.77999411220912));
#31175=CARTESIAN_POINT('Ctrl Pts',(0.759614401109868,1.,-1.78596964884527));
#31176=CARTESIAN_POINT('Ctrl Pts',(0.760469555880425,1.,-1.79185815610802));
#31177=CARTESIAN_POINT('Ctrl Pts',(0.761229695230359,1.,-1.79768986997735));
#31178=CARTESIAN_POINT('Ctrl Pts',(0.761915336443515,1.,-1.80351583877334));
#31179=CARTESIAN_POINT('Ctrl Pts',(0.762546129464036,1.,-1.80938551463989));
#31180=CARTESIAN_POINT('Ctrl Pts',(0.763132003836783,1.,-1.81532118405566));
#31181=CARTESIAN_POINT('Ctrl Pts',(0.763673465462854,1.,-1.82131873145297));
#31182=CARTESIAN_POINT('Ctrl Pts',(0.764165902606055,1.,-1.8273599120008));
#31183=CARTESIAN_POINT('Ctrl Pts',(0.764602549687845,1.,-1.8334207722714));
#31184=CARTESIAN_POINT('Ctrl Pts',(0.764978057881687,1.,-1.83948181064823));
#31185=CARTESIAN_POINT('Ctrl Pts',(0.765291664861971,1.,-1.84553698875911));
#31186=CARTESIAN_POINT('Ctrl Pts',(0.765545710619023,1.,-1.85158945130054));
#31187=CARTESIAN_POINT('Ctrl Pts',(0.765744212909305,1.,-1.85764741390391));
#31188=CARTESIAN_POINT('Ctrl Pts',(0.765891519092557,1.,-1.86372027063315));
#31189=CARTESIAN_POINT('Ctrl Pts',(0.765990708546111,1.,-1.86981398314345));
#31190=CARTESIAN_POINT('Ctrl Pts',(0.766042837036759,1.,-1.87592888967886));
#31191=CARTESIAN_POINT('Ctrl Pts',(0.766047794851868,1.,-1.88206215302561));
#31192=CARTESIAN_POINT('Ctrl Pts',(0.76600483706209,1.,-1.88820926433409));
#31193=CARTESIAN_POINT('Ctrl Pts',(0.765913193856979,1.,-1.89436577771389));
#31194=CARTESIAN_POINT('Ctrl Pts',(0.765772772593395,1.,-1.90052930393599));
#31195=CARTESIAN_POINT('Ctrl Pts',(0.765584196937936,1.,-1.90669961402362));
#31196=CARTESIAN_POINT('Ctrl Pts',(0.765348465884739,1.,-1.91287765805174));
#31197=CARTESIAN_POINT('Ctrl Pts',(0.765066729667095,1.,-1.91906491634197));
#31198=CARTESIAN_POINT('Ctrl Pts',(0.764740025488189,1.,-1.92526263537041));
#31199=CARTESIAN_POINT('Ctrl Pts',(0.764369010673889,1.,-1.93147105496367));
#31200=CARTESIAN_POINT('Ctrl Pts',(0.763954049121393,1.,-1.93768964875867));
#31201=CARTESIAN_POINT('Ctrl Pts',(0.76349533353858,1.,-1.94391746617626));
#31202=CARTESIAN_POINT('Ctrl Pts',(0.762992990878774,1.,-1.95015342590025));
#31203=CARTESIAN_POINT('Ctrl Pts',(0.762447203806263,1.,-1.95639665309893));
#31204=CARTESIAN_POINT('Ctrl Pts',(0.761858300014575,1.,-1.96264672744229));
#31205=CARTESIAN_POINT('Ctrl Pts',(0.761226690483986,1.,-1.96890351582545));
#31206=CARTESIAN_POINT('Ctrl Pts',(0.760552825409855,1.,-1.97516705321521));
#31207=CARTESIAN_POINT('Ctrl Pts',(0.759837147452135,1.,-1.98143741418156));
#31208=CARTESIAN_POINT('Ctrl Pts',(0.759080037802242,1.,-1.98771456680806));
#31209=CARTESIAN_POINT('Ctrl Pts',(0.758281796766377,1.,-1.9939983109871));
#31210=CARTESIAN_POINT('Ctrl Pts',(0.757442676862341,1.,-2.00028834739072));
#31211=CARTESIAN_POINT('Ctrl Pts',(0.756562904646496,1.,-2.00658431587682));
#31212=CARTESIAN_POINT('Ctrl Pts',(0.7556427049581,1.,-2.01288584328149));
#31213=CARTESIAN_POINT('Ctrl Pts',(0.75468233072352,1.,-2.01919259406003));
#31214=CARTESIAN_POINT('Ctrl Pts',(0.753682061113765,1.,-2.02550428623587));
#31215=CARTESIAN_POINT('Ctrl Pts',(0.752642180488104,1.,-2.03182068456467));
#31216=CARTESIAN_POINT('Ctrl Pts',(0.751562963361383,1.,-2.03814160092173));
#31217=CARTESIAN_POINT('Ctrl Pts',(0.750444657874758,1.,-2.04446689147754));
#31218=CARTESIAN_POINT('Ctrl Pts',(0.749287468663053,1.,-2.05079645591606));
#31219=CARTESIAN_POINT('Ctrl Pts',(0.748091554181101,1.,-2.05713023030263));
#31220=CARTESIAN_POINT('Ctrl Pts',(0.747103932785504,1.,-2.06220058927162));
#31221=CARTESIAN_POINT('Ctrl Pts',(0.746345871542695,1.,-2.06600523016401));
#31222=CARTESIAN_POINT('Ctrl Pts',(0.74583279137781,1.,-2.06854248895575));
#31223=CARTESIAN_POINT('Ctrl Pts',(0.745574324794401,1.,-2.0698113262342));
#31224=CARTESIAN_POINT('',(0.693717979106306,0.,-1.60662857109684));
#31225=CARTESIAN_POINT('Origin',(0.,0.,0.));
#31226=CARTESIAN_POINT('',(0.892032620296855,1.,-1.5055822144029));
#31227=CARTESIAN_POINT('Origin',(0.,1.,0.));
#31228=CARTESIAN_POINT('',(0.892032620296855,0.,-1.5055822144029));
#31229=CARTESIAN_POINT('Ctrl Pts',(1.23627494547115,-1.,-1.81978687191668));
#31230=CARTESIAN_POINT('Ctrl Pts',(1.23627494547115,1.,-1.81978687191668));
#31231=CARTESIAN_POINT('Ctrl Pts',(1.23509651170476,-1.,-1.81925017193666));
#31232=CARTESIAN_POINT('Ctrl Pts',(1.23509651170476,1.,-1.81925017193666));
#31233=CARTESIAN_POINT('Ctrl Pts',(1.2327422452705,-1.,-1.81817389921279));
#31234=CARTESIAN_POINT('Ctrl Pts',(1.2327422452705,1.,-1.81817389921279));
#31235=CARTESIAN_POINT('Ctrl Pts',(1.2292186489137,-1.,-1.8165508718364));
#31236=CARTESIAN_POINT('Ctrl Pts',(1.2292186489137,1.,-1.8165508718364));
#31237=CARTESIAN_POINT('Ctrl Pts',(1.2245361330495,-1.,-1.81436959210434));
#31238=CARTESIAN_POINT('Ctrl Pts',(1.2245361330495,1.,-1.81436959210434));
#31239=CARTESIAN_POINT('Ctrl Pts',(1.21870906103557,-1.,-1.81161420806656));
#31240=CARTESIAN_POINT('Ctrl Pts',(1.21870906103557,1.,-1.81161420806656));
#31241=CARTESIAN_POINT('Ctrl Pts',(1.21290815708314,-1.,-1.80882996917129));
#31242=CARTESIAN_POINT('Ctrl Pts',(1.21290815708314,1.,-1.80882996917129));
#31243=CARTESIAN_POINT('Ctrl Pts',(1.20713356605475,-1.,-1.80601678480707));
#31244=CARTESIAN_POINT('Ctrl Pts',(1.20713356605475,1.,-1.80601678480707));
#31245=CARTESIAN_POINT('Ctrl Pts',(1.20138548938974,-1.,-1.80317454838603));
#31246=CARTESIAN_POINT('Ctrl Pts',(1.20138548938974,1.,-1.80317454838603));
#31247=CARTESIAN_POINT('Ctrl Pts',(1.19566418930242,-1.,-1.80030314369879));
#31248=CARTESIAN_POINT('Ctrl Pts',(1.19566418930242,1.,-1.80030314369879));
#31249=CARTESIAN_POINT('Ctrl Pts',(1.18996997934445,-1.,-1.79740245923478));
#31250=CARTESIAN_POINT('Ctrl Pts',(1.18996997934445,1.,-1.79740245923478));
#31251=CARTESIAN_POINT('Ctrl Pts',(1.18430321697432,-1.,-1.79447240321515));
#31252=CARTESIAN_POINT('Ctrl Pts',(1.18430321697432,1.,-1.79447240321515));
#31253=CARTESIAN_POINT('Ctrl Pts',(1.17866429440809,-1.,-1.79151291552689));
#31254=CARTESIAN_POINT('Ctrl Pts',(1.17866429440809,1.,-1.79151291552689));
#31255=CARTESIAN_POINT('Ctrl Pts',(1.17305363177328,-1.,-1.78852398877617));
#31256=CARTESIAN_POINT('Ctrl Pts',(1.17305363177328,1.,-1.78852398877617));
#31257=CARTESIAN_POINT('Ctrl Pts',(1.16747166312303,-1.,-1.78550566040443));
#31258=CARTESIAN_POINT('Ctrl Pts',(1.16747166312303,1.,-1.78550566040443));
#31259=CARTESIAN_POINT('Ctrl Pts',(1.16191881298499,-1.,-1.78245795881009));
#31260=CARTESIAN_POINT('Ctrl Pts',(1.16191881298499,1.,-1.78245795881009));
#31261=CARTESIAN_POINT('Ctrl Pts',(1.15639547194698,-1.,-1.77938085564275));
#31262=CARTESIAN_POINT('Ctrl Pts',(1.15639547194698,1.,-1.77938085564275));
#31263=CARTESIAN_POINT('Ctrl Pts',(1.15090197841514,-1.,-1.7762742255701));
#31264=CARTESIAN_POINT('Ctrl Pts',(1.15090197841514,1.,-1.7762742255701));
#31265=CARTESIAN_POINT('Ctrl Pts',(1.1454385822692,-1.,-1.77313777896194));
#31266=CARTESIAN_POINT('Ctrl Pts',(1.1454385822692,1.,-1.77313777896194));
#31267=CARTESIAN_POINT('Ctrl Pts',(1.14000548336975,-1.,-1.76997111386769));
#31268=CARTESIAN_POINT('Ctrl Pts',(1.14000548336975,1.,-1.76997111386769));
#31269=CARTESIAN_POINT('Ctrl Pts',(1.1346029180462,-1.,-1.76677384551862));
#31270=CARTESIAN_POINT('Ctrl Pts',(1.1346029180462,1.,-1.76677384551862));
#31271=CARTESIAN_POINT('Ctrl Pts',(1.12923123555075,-1.,-1.7635457196617));
#31272=CARTESIAN_POINT('Ctrl Pts',(1.12923123555075,1.,-1.7635457196617));
#31273=CARTESIAN_POINT('Ctrl Pts',(1.12389096855086,-1.,-1.76028671825096));
#31274=CARTESIAN_POINT('Ctrl Pts',(1.12389096855086,1.,-1.76028671825096));
#31275=CARTESIAN_POINT('Ctrl Pts',(1.11858293216763,-1.,-1.75699720772105));
#31276=CARTESIAN_POINT('Ctrl Pts',(1.11858293216763,1.,-1.75699720772105));
#31277=CARTESIAN_POINT('Ctrl Pts',(1.11330807582551,-1.,-1.7536777209463));
#31278=CARTESIAN_POINT('Ctrl Pts',(1.11330807582551,1.,-1.7536777209463));
#31279=CARTESIAN_POINT('Ctrl Pts',(1.10806728183007,-1.,-1.7503286607592));
#31280=CARTESIAN_POINT('Ctrl Pts',(1.10806728183007,1.,-1.7503286607592));
#31281=CARTESIAN_POINT('Ctrl Pts',(1.10286118991143,-1.,-1.74695004214923));
#31282=CARTESIAN_POINT('Ctrl Pts',(1.10286118991143,1.,-1.74695004214923));
#31283=CARTESIAN_POINT('Ctrl Pts',(1.09768999241225,-1.,-1.74354119236208));
#31284=CARTESIAN_POINT('Ctrl Pts',(1.09768999241225,1.,-1.74354119236208));
#31285=CARTESIAN_POINT('Ctrl Pts',(1.09255329056493,-1.,-1.74010053962247));
#31286=CARTESIAN_POINT('Ctrl Pts',(1.09255329056493,1.,-1.74010053962247));
#31287=CARTESIAN_POINT('Ctrl Pts',(1.08745056285427,-1.,-1.73662628326091));
#31288=CARTESIAN_POINT('Ctrl Pts',(1.08745056285427,1.,-1.73662628326091));
#31289=CARTESIAN_POINT('Ctrl Pts',(1.08238162784749,-1.,-1.73311705663407));
#31290=CARTESIAN_POINT('Ctrl Pts',(1.08238162784749,1.,-1.73311705663407));
#31291=CARTESIAN_POINT('Ctrl Pts',(1.0773470373727,-1.,-1.72957248977424));
#31292=CARTESIAN_POINT('Ctrl Pts',(1.0773470373727,1.,-1.72957248977424));
#31293=CARTESIAN_POINT('Ctrl Pts',(1.07234866990252,-1.,-1.72599406198488));
#31294=CARTESIAN_POINT('Ctrl Pts',(1.07234866990252,1.,-1.72599406198488));
#31295=CARTESIAN_POINT('Ctrl Pts',(1.06738966975462,-1.,-1.72238500928453));
#31296=CARTESIAN_POINT('Ctrl Pts',(1.06738966975462,1.,-1.72238500928453));
#31297=CARTESIAN_POINT('Ctrl Pts',(1.06247324680647,-1.,-1.71874858456904));
#31298=CARTESIAN_POINT('Ctrl Pts',(1.06247324680647,1.,-1.71874858456904));
#31299=CARTESIAN_POINT('Ctrl Pts',(1.05760163192479,-1.,-1.7150865442702));
#31300=CARTESIAN_POINT('Ctrl Pts',(1.05760163192479,1.,-1.7150865442702));
#31301=CARTESIAN_POINT('Ctrl Pts',(1.05277517202855,-1.,-1.71139783543989));
#31302=CARTESIAN_POINT('Ctrl Pts',(1.05277517202855,1.,-1.71139783543989));
#31303=CARTESIAN_POINT('Ctrl Pts',(1.04799085404995,-1.,-1.70767646263649));
#31304=CARTESIAN_POINT('Ctrl Pts',(1.04799085404995,1.,-1.70767646263649));
#31305=CARTESIAN_POINT('Ctrl Pts',(1.04324363334554,-1.,-1.70391338707982));
#31306=CARTESIAN_POINT('Ctrl Pts',(1.04324363334554,1.,-1.70391338707982));
#31307=CARTESIAN_POINT('Ctrl Pts',(1.03852922490789,-1.,-1.70010052930962));
#31308=CARTESIAN_POINT('Ctrl Pts',(1.03852922490789,1.,-1.70010052930962));
#31309=CARTESIAN_POINT('Ctrl Pts',(1.03384646003588,-1.,-1.69623414782771));
#31310=CARTESIAN_POINT('Ctrl Pts',(1.03384646003588,1.,-1.69623414782771));
#31311=CARTESIAN_POINT('Ctrl Pts',(1.02919977579147,-1.,-1.69231840863458));
#31312=CARTESIAN_POINT('Ctrl Pts',(1.02919977579147,1.,-1.69231840863458));
#31313=CARTESIAN_POINT('Ctrl Pts',(1.02460180535255,-1.,-1.68836910178447));
#31314=CARTESIAN_POINT('Ctrl Pts',(1.02460180535255,1.,-1.68836910178447));
#31315=CARTESIAN_POINT('Ctrl Pts',(1.02006795074201,-1.,-1.68440578021706));
#31316=CARTESIAN_POINT('Ctrl Pts',(1.02006795074201,1.,-1.68440578021706));
#31317=CARTESIAN_POINT('Ctrl Pts',(1.01561026162773,-1.,-1.68044289894798));
#31318=CARTESIAN_POINT('Ctrl Pts',(1.01561026162773,1.,-1.68044289894798));
#31319=CARTESIAN_POINT('Ctrl Pts',(1.01123236493511,-1.,-1.67648246776464));
#31320=CARTESIAN_POINT('Ctrl Pts',(1.01123236493511,1.,-1.67648246776464));
#31321=CARTESIAN_POINT('Ctrl Pts',(1.00692206696414,-1.,-1.67250335383293));
#31322=CARTESIAN_POINT('Ctrl Pts',(1.00692206696414,1.,-1.67250335383293));
#31323=CARTESIAN_POINT('Ctrl Pts',(1.00265091003727,-1.,-1.66846059277303));
#31324=CARTESIAN_POINT('Ctrl Pts',(1.00265091003727,1.,-1.66846059277303));
#31325=CARTESIAN_POINT('Ctrl Pts',(0.998389654952757,-1.,-1.66430758030376));
#31326=CARTESIAN_POINT('Ctrl Pts',(0.998389654952757,1.,-1.66430758030376));
#31327=CARTESIAN_POINT('Ctrl Pts',(0.994121836661305,-1.,-1.66001553809947));
#31328=CARTESIAN_POINT('Ctrl Pts',(0.994121836661305,1.,-1.66001553809947));
#31329=CARTESIAN_POINT('Ctrl Pts',(0.989855627854164,-1.,-1.65559044289699));
#31330=CARTESIAN_POINT('Ctrl Pts',(0.989855627854164,1.,-1.65559044289699));
#31331=CARTESIAN_POINT('Ctrl Pts',(0.98564262292082,-1.,-1.65110016612638));
#31332=CARTESIAN_POINT('Ctrl Pts',(0.98564262292082,1.,-1.65110016612638));
#31333=CARTESIAN_POINT('Ctrl Pts',(0.981562530939489,-1.,-1.64665139190656));
#31334=CARTESIAN_POINT('Ctrl Pts',(0.981562530939489,1.,-1.64665139190656));
#31335=CARTESIAN_POINT('Ctrl Pts',(0.977689794119416,-1.,-1.64233990826687));
#31336=CARTESIAN_POINT('Ctrl Pts',(0.977689794119416,1.,-1.64233990826687));
#31337=CARTESIAN_POINT('Ctrl Pts',(0.974066058287418,-1.,-1.63820952658144));
#31338=CARTESIAN_POINT('Ctrl Pts',(0.974066058287418,1.,-1.63820952658144));
#31339=CARTESIAN_POINT('Ctrl Pts',(0.970669715997509,-1.,-1.63420665729798));
#31340=CARTESIAN_POINT('Ctrl Pts',(0.970669715997509,1.,-1.63420665729798));
#31341=CARTESIAN_POINT('Ctrl Pts',(0.967387853230345,-1.,-1.63013849959462));
#31342=CARTESIAN_POINT('Ctrl Pts',(0.967387853230345,1.,-1.63013849959462));
#31343=CARTESIAN_POINT('Ctrl Pts',(0.964046107040535,-1.,-1.62571930670187));
#31344=CARTESIAN_POINT('Ctrl Pts',(0.964046107040535,1.,-1.62571930670187));
#31345=CARTESIAN_POINT('Ctrl Pts',(0.960438326101728,-1.,-1.62061638140221));
#31346=CARTESIAN_POINT('Ctrl Pts',(0.960438326101728,1.,-1.62061638140221));
#31347=CARTESIAN_POINT('Ctrl Pts',(0.95635442292067,-1.,-1.61449324337085));
#31348=CARTESIAN_POINT('Ctrl Pts',(0.95635442292067,1.,-1.61449324337085));
#31349=CARTESIAN_POINT('Ctrl Pts',(0.951613284356035,-1.,-1.60706069896936));
#31350=CARTESIAN_POINT('Ctrl Pts',(0.951613284356035,1.,-1.60706069896936));
#31351=CARTESIAN_POINT('Ctrl Pts',(0.946078063315257,-1.,-1.59810042043673));
#31352=CARTESIAN_POINT('Ctrl Pts',(0.946078063315257,1.,-1.59810042043673));
#31353=CARTESIAN_POINT('Ctrl Pts',(0.939646377893399,-1.,-1.58744937487176));
#31354=CARTESIAN_POINT('Ctrl Pts',(0.939646377893399,1.,-1.58744937487176));
#31355=CARTESIAN_POINT('Ctrl Pts',(0.932246680108685,-1.,-1.57499388382243));
#31356=CARTESIAN_POINT('Ctrl Pts',(0.932246680108685,1.,-1.57499388382243));
#31357=CARTESIAN_POINT('Ctrl Pts',(0.923832188944341,-1.,-1.56065988578893));
#31358=CARTESIAN_POINT('Ctrl Pts',(0.923832188944341,1.,-1.56065988578893));
#31359=CARTESIAN_POINT('Ctrl Pts',(0.914375919026456,-1.,-1.54440491149498));
#31360=CARTESIAN_POINT('Ctrl Pts',(0.914375919026456,1.,-1.54440491149498));
#31361=CARTESIAN_POINT('Ctrl Pts',(0.905967409625651,-1.,-1.52984849887993));
#31362=CARTESIAN_POINT('Ctrl Pts',(0.905967409625651,1.,-1.52984849887993));
#31363=CARTESIAN_POINT('Ctrl Pts',(0.89918504748351,-1.,-1.51805569590094));
#31364=CARTESIAN_POINT('Ctrl Pts',(0.89918504748351,1.,-1.51805569590094));
#31365=CARTESIAN_POINT('Ctrl Pts',(0.894452006964543,-1.,-1.50980486806688));
#31366=CARTESIAN_POINT('Ctrl Pts',(0.894452006964543,1.,-1.50980486806688));
#31367=CARTESIAN_POINT('Ctrl Pts',(0.892032620296855,-1.,-1.5055822144029));
#31368=CARTESIAN_POINT('Ctrl Pts',(0.892032620296855,1.,-1.5055822144029));
#31369=CARTESIAN_POINT('',(1.23627494547115,1.,-1.81978687191668));
#31370=CARTESIAN_POINT('Ctrl Pts',(1.23627494547115,1.,-1.81978687191668));
#31371=CARTESIAN_POINT('Ctrl Pts',(1.23509651170476,1.,-1.81925017193666));
#31372=CARTESIAN_POINT('Ctrl Pts',(1.2327422452705,1.,-1.81817389921279));
#31373=CARTESIAN_POINT('Ctrl Pts',(1.2292186489137,1.,-1.8165508718364));
#31374=CARTESIAN_POINT('Ctrl Pts',(1.2245361330495,1.,-1.81436959210434));
#31375=CARTESIAN_POINT('Ctrl Pts',(1.21870906103557,1.,-1.81161420806656));
#31376=CARTESIAN_POINT('Ctrl Pts',(1.21290815708314,1.,-1.80882996917129));
#31377=CARTESIAN_POINT('Ctrl Pts',(1.20713356605475,1.,-1.80601678480707));
#31378=CARTESIAN_POINT('Ctrl Pts',(1.20138548938974,1.,-1.80317454838603));
#31379=CARTESIAN_POINT('Ctrl Pts',(1.19566418930242,1.,-1.80030314369879));
#31380=CARTESIAN_POINT('Ctrl Pts',(1.18996997934445,1.,-1.79740245923478));
#31381=CARTESIAN_POINT('Ctrl Pts',(1.18430321697432,1.,-1.79447240321515));
#31382=CARTESIAN_POINT('Ctrl Pts',(1.17866429440809,1.,-1.79151291552689));
#31383=CARTESIAN_POINT('Ctrl Pts',(1.17305363177328,1.,-1.78852398877617));
#31384=CARTESIAN_POINT('Ctrl Pts',(1.16747166312303,1.,-1.78550566040443));
#31385=CARTESIAN_POINT('Ctrl Pts',(1.16191881298499,1.,-1.78245795881009));
#31386=CARTESIAN_POINT('Ctrl Pts',(1.15639547194698,1.,-1.77938085564275));
#31387=CARTESIAN_POINT('Ctrl Pts',(1.15090197841514,1.,-1.7762742255701));
#31388=CARTESIAN_POINT('Ctrl Pts',(1.1454385822692,1.,-1.77313777896194));
#31389=CARTESIAN_POINT('Ctrl Pts',(1.14000548336975,1.,-1.76997111386769));
#31390=CARTESIAN_POINT('Ctrl Pts',(1.1346029180462,1.,-1.76677384551862));
#31391=CARTESIAN_POINT('Ctrl Pts',(1.12923123555075,1.,-1.7635457196617));
#31392=CARTESIAN_POINT('Ctrl Pts',(1.12389096855086,1.,-1.76028671825096));
#31393=CARTESIAN_POINT('Ctrl Pts',(1.11858293216763,1.,-1.75699720772105));
#31394=CARTESIAN_POINT('Ctrl Pts',(1.11330807582551,1.,-1.7536777209463));
#31395=CARTESIAN_POINT('Ctrl Pts',(1.10806728183007,1.,-1.7503286607592));
#31396=CARTESIAN_POINT('Ctrl Pts',(1.10286118991143,1.,-1.74695004214923));
#31397=CARTESIAN_POINT('Ctrl Pts',(1.09768999241225,1.,-1.74354119236208));
#31398=CARTESIAN_POINT('Ctrl Pts',(1.09255329056493,1.,-1.74010053962247));
#31399=CARTESIAN_POINT('Ctrl Pts',(1.08745056285427,1.,-1.73662628326091));
#31400=CARTESIAN_POINT('Ctrl Pts',(1.08238162784749,1.,-1.73311705663407));
#31401=CARTESIAN_POINT('Ctrl Pts',(1.0773470373727,1.,-1.72957248977424));
#31402=CARTESIAN_POINT('Ctrl Pts',(1.07234866990252,1.,-1.72599406198488));
#31403=CARTESIAN_POINT('Ctrl Pts',(1.06738966975462,1.,-1.72238500928453));
#31404=CARTESIAN_POINT('Ctrl Pts',(1.06247324680647,1.,-1.71874858456904));
#31405=CARTESIAN_POINT('Ctrl Pts',(1.05760163192479,1.,-1.7150865442702));
#31406=CARTESIAN_POINT('Ctrl Pts',(1.05277517202855,1.,-1.71139783543989));
#31407=CARTESIAN_POINT('Ctrl Pts',(1.04799085404995,1.,-1.70767646263649));
#31408=CARTESIAN_POINT('Ctrl Pts',(1.04324363334554,1.,-1.70391338707982));
#31409=CARTESIAN_POINT('Ctrl Pts',(1.03852922490789,1.,-1.70010052930962));
#31410=CARTESIAN_POINT('Ctrl Pts',(1.03384646003588,1.,-1.69623414782771));
#31411=CARTESIAN_POINT('Ctrl Pts',(1.02919977579147,1.,-1.69231840863458));
#31412=CARTESIAN_POINT('Ctrl Pts',(1.02460180535255,1.,-1.68836910178447));
#31413=CARTESIAN_POINT('Ctrl Pts',(1.02006795074201,1.,-1.68440578021706));
#31414=CARTESIAN_POINT('Ctrl Pts',(1.01561026162773,1.,-1.68044289894798));
#31415=CARTESIAN_POINT('Ctrl Pts',(1.01123236493511,1.,-1.67648246776464));
#31416=CARTESIAN_POINT('Ctrl Pts',(1.00692206696414,1.,-1.67250335383293));
#31417=CARTESIAN_POINT('Ctrl Pts',(1.00265091003727,1.,-1.66846059277303));
#31418=CARTESIAN_POINT('Ctrl Pts',(0.998389654952757,1.,-1.66430758030376));
#31419=CARTESIAN_POINT('Ctrl Pts',(0.994121836661305,1.,-1.66001553809947));
#31420=CARTESIAN_POINT('Ctrl Pts',(0.989855627854164,1.,-1.65559044289699));
#31421=CARTESIAN_POINT('Ctrl Pts',(0.98564262292082,1.,-1.65110016612638));
#31422=CARTESIAN_POINT('Ctrl Pts',(0.981562530939489,1.,-1.64665139190656));
#31423=CARTESIAN_POINT('Ctrl Pts',(0.977689794119416,1.,-1.64233990826687));
#31424=CARTESIAN_POINT('Ctrl Pts',(0.974066058287418,1.,-1.63820952658144));
#31425=CARTESIAN_POINT('Ctrl Pts',(0.970669715997509,1.,-1.63420665729798));
#31426=CARTESIAN_POINT('Ctrl Pts',(0.967387853230345,1.,-1.63013849959462));
#31427=CARTESIAN_POINT('Ctrl Pts',(0.964046107040535,1.,-1.62571930670187));
#31428=CARTESIAN_POINT('Ctrl Pts',(0.960438326101728,1.,-1.62061638140221));
#31429=CARTESIAN_POINT('Ctrl Pts',(0.95635442292067,1.,-1.61449324337085));
#31430=CARTESIAN_POINT('Ctrl Pts',(0.951613284356035,1.,-1.60706069896936));
#31431=CARTESIAN_POINT('Ctrl Pts',(0.946078063315257,1.,-1.59810042043673));
#31432=CARTESIAN_POINT('Ctrl Pts',(0.939646377893399,1.,-1.58744937487176));
#31433=CARTESIAN_POINT('Ctrl Pts',(0.932246680108685,1.,-1.57499388382243));
#31434=CARTESIAN_POINT('Ctrl Pts',(0.923832188944341,1.,-1.56065988578893));
#31435=CARTESIAN_POINT('Ctrl Pts',(0.914375919026456,1.,-1.54440491149498));
#31436=CARTESIAN_POINT('Ctrl Pts',(0.905967409625651,1.,-1.52984849887993));
#31437=CARTESIAN_POINT('Ctrl Pts',(0.89918504748351,1.,-1.51805569590094));
#31438=CARTESIAN_POINT('Ctrl Pts',(0.894452006964543,1.,-1.50980486806688));
#31439=CARTESIAN_POINT('Ctrl Pts',(0.892032620296855,1.,-1.5055822144029));
#31440=CARTESIAN_POINT('',(1.23627494547115,0.,-1.81978687191668));
#31441=CARTESIAN_POINT('Origin',(1.34869019493419,0.,-1.73811241238545));
#31442=CARTESIAN_POINT('',(1.34869019493419,1.,-1.73811241238545));
#31443=CARTESIAN_POINT('',(1.23627494547115,1.,-1.81978687191668));
#31444=CARTESIAN_POINT('',(1.34869019493419,0.,-1.73811241238545));
#31445=CARTESIAN_POINT('Ctrl Pts',(1.15624053661742,-1.,-1.31362392696032));
#31446=CARTESIAN_POINT('Ctrl Pts',(1.15624053661742,1.,-1.31362392696032));
#31447=CARTESIAN_POINT('Ctrl Pts',(1.15950888730809,-1.,-1.31722977216397));
#31448=CARTESIAN_POINT('Ctrl Pts',(1.15950888730809,1.,-1.31722977216397));
#31449=CARTESIAN_POINT('Ctrl Pts',(1.16589330093588,-1.,-1.32428080721772));
#31450=CARTESIAN_POINT('Ctrl Pts',(1.16589330093588,1.,-1.32428080721772));
#31451=CARTESIAN_POINT('Ctrl Pts',(1.17501305789857,-1.,-1.33437539347008));
#31452=CARTESIAN_POINT('Ctrl Pts',(1.17501305789857,1.,-1.33437539347008));
#31453=CARTESIAN_POINT('Ctrl Pts',(1.18625865667441,-1.,-1.34687054001093));
#31454=CARTESIAN_POINT('Ctrl Pts',(1.18625865667441,1.,-1.34687054001093));
#31455=CARTESIAN_POINT('Ctrl Pts',(1.1987959077932,-1.,-1.36088705043885));
#31456=CARTESIAN_POINT('Ctrl Pts',(1.1987959077932,1.,-1.36088705043885));
#31457=CARTESIAN_POINT('Ctrl Pts',(1.20982812925645,-1.,-1.37331915607905));
#31458=CARTESIAN_POINT('Ctrl Pts',(1.20982812925645,1.,-1.37331915607905));
#31459=CARTESIAN_POINT('Ctrl Pts',(1.21938737280852,-1.,-1.38420564527715));
#31460=CARTESIAN_POINT('Ctrl Pts',(1.21938737280852,1.,-1.38420564527715));
#31461=CARTESIAN_POINT('Ctrl Pts',(1.22752961899387,-1.,-1.39361389568796));
#31462=CARTESIAN_POINT('Ctrl Pts',(1.22752961899387,1.,-1.39361389568796));
#31463=CARTESIAN_POINT('Ctrl Pts',(1.23434087290423,-1.,-1.40164708206106));
#31464=CARTESIAN_POINT('Ctrl Pts',(1.23434087290423,1.,-1.40164708206106));
#31465=CARTESIAN_POINT('Ctrl Pts',(1.23994455029534,-1.,-1.40845295531283));
#31466=CARTESIAN_POINT('Ctrl Pts',(1.23994455029534,1.,-1.40845295531283));
#31467=CARTESIAN_POINT('Ctrl Pts',(1.24450600513056,-1.,-1.41422913175179));
#31468=CARTESIAN_POINT('Ctrl Pts',(1.24450600513056,1.,-1.41422913175179));
#31469=CARTESIAN_POINT('Ctrl Pts',(1.24824430986571,-1.,-1.41923722596025));
#31470=CARTESIAN_POINT('Ctrl Pts',(1.24824430986571,1.,-1.41923722596025));
#31471=CARTESIAN_POINT('Ctrl Pts',(1.2514145557001,-1.,-1.42378102115575));
#31472=CARTESIAN_POINT('Ctrl Pts',(1.2514145557001,1.,-1.42378102115575));
#31473=CARTESIAN_POINT('Ctrl Pts',(1.25426945222639,-1.,-1.42815938799387));
#31474=CARTESIAN_POINT('Ctrl Pts',(1.25426945222639,1.,-1.42815938799387));
#31475=CARTESIAN_POINT('Ctrl Pts',(1.25702687965755,-1.,-1.43262645609691));
#31476=CARTESIAN_POINT('Ctrl Pts',(1.25702687965755,1.,-1.43262645609691));
#31477=CARTESIAN_POINT('Ctrl Pts',(1.25983531012005,-1.,-1.43734919180848));
#31478=CARTESIAN_POINT('Ctrl Pts',(1.25983531012005,1.,-1.43734919180848));
#31479=CARTESIAN_POINT('Ctrl Pts',(1.26273903323858,-1.,-1.44236470511303));
#31480=CARTESIAN_POINT('Ctrl Pts',(1.26273903323858,1.,-1.44236470511303));
#31481=CARTESIAN_POINT('Ctrl Pts',(1.26570925118868,-1.,-1.44761985001662));
#31482=CARTESIAN_POINT('Ctrl Pts',(1.26570925118868,1.,-1.44761985001662));
#31483=CARTESIAN_POINT('Ctrl Pts',(1.2686778680489,-1.,-1.45301422764247));
#31484=CARTESIAN_POINT('Ctrl Pts',(1.2686778680489,1.,-1.45301422764247));
#31485=CARTESIAN_POINT('Ctrl Pts',(1.27156805265289,-1.,-1.45843906294697));
#31486=CARTESIAN_POINT('Ctrl Pts',(1.27156805265289,1.,-1.45843906294697));
#31487=CARTESIAN_POINT('Ctrl Pts',(1.27433119897822,-1.,-1.46382431332476));
#31488=CARTESIAN_POINT('Ctrl Pts',(1.27433119897822,1.,-1.46382431332476));
#31489=CARTESIAN_POINT('Ctrl Pts',(1.27696414831089,-1.,-1.46916035917133));
#31490=CARTESIAN_POINT('Ctrl Pts',(1.27696414831089,1.,-1.46916035917133));
#31491=CARTESIAN_POINT('Ctrl Pts',(1.2794891824849,-1.,-1.4744717526707));
#31492=CARTESIAN_POINT('Ctrl Pts',(1.2794891824849,1.,-1.4744717526707));
#31493=CARTESIAN_POINT('Ctrl Pts',(1.28194158939517,-1.,-1.47980070347096));
#31494=CARTESIAN_POINT('Ctrl Pts',(1.28194158939517,1.,-1.47980070347096));
#31495=CARTESIAN_POINT('Ctrl Pts',(1.28435533880201,-1.,-1.4851881711891));
#31496=CARTESIAN_POINT('Ctrl Pts',(1.28435533880201,1.,-1.4851881711891));
#31497=CARTESIAN_POINT('Ctrl Pts',(1.2867467611644,-1.,-1.4906522831278));
#31498=CARTESIAN_POINT('Ctrl Pts',(1.2867467611644,1.,-1.4906522831278));
#31499=CARTESIAN_POINT('Ctrl Pts',(1.28911506584254,-1.,-1.49618896881754));
#31500=CARTESIAN_POINT('Ctrl Pts',(1.28911506584254,1.,-1.49618896881754));
#31501=CARTESIAN_POINT('Ctrl Pts',(1.29145022885181,-1.,-1.50178230149776));
#31502=CARTESIAN_POINT('Ctrl Pts',(1.29145022885181,1.,-1.50178230149776));
#31503=CARTESIAN_POINT('Ctrl Pts',(1.29373841372842,-1.,-1.50741159078365));
#31504=CARTESIAN_POINT('Ctrl Pts',(1.29373841372842,1.,-1.50741159078365));
#31505=CARTESIAN_POINT('Ctrl Pts',(1.29596850710509,-1.,-1.51305994241402));
#31506=CARTESIAN_POINT('Ctrl Pts',(1.29596850710509,1.,-1.51305994241402));
#31507=CARTESIAN_POINT('Ctrl Pts',(1.29813791800747,-1.,-1.51872184912724));
#31508=CARTESIAN_POINT('Ctrl Pts',(1.29813791800747,1.,-1.51872184912724));
#31509=CARTESIAN_POINT('Ctrl Pts',(1.30024984366328,-1.,-1.52439957861062));
#31510=CARTESIAN_POINT('Ctrl Pts',(1.30024984366328,1.,-1.52439957861062));
#31511=CARTESIAN_POINT('Ctrl Pts',(1.30231064395568,-1.,-1.53009970283891));
#31512=CARTESIAN_POINT('Ctrl Pts',(1.30231064395568,1.,-1.53009970283891));
#31513=CARTESIAN_POINT('Ctrl Pts',(1.30432735639489,-1.,-1.53582981268977));
#31514=CARTESIAN_POINT('Ctrl Pts',(1.30432735639489,1.,-1.53582981268977));
#31515=CARTESIAN_POINT('Ctrl Pts',(1.30630475189556,-1.,-1.54159462645432));
#31516=CARTESIAN_POINT('Ctrl Pts',(1.30630475189556,1.,-1.54159462645432));
#31517=CARTESIAN_POINT('Ctrl Pts',(1.30824393907473,-1.,-1.54739413957185));
#31518=CARTESIAN_POINT('Ctrl Pts',(1.30824393907473,1.,-1.54739413957185));
#31519=CARTESIAN_POINT('Ctrl Pts',(1.31014393684222,-1.,-1.55322568759481));
#31520=CARTESIAN_POINT('Ctrl Pts',(1.31014393684222,1.,-1.55322568759481));
#31521=CARTESIAN_POINT('Ctrl Pts',(1.31200264341696,-1.,-1.55908521254821));
#31522=CARTESIAN_POINT('Ctrl Pts',(1.31200264341696,1.,-1.55908521254821));
#31523=CARTESIAN_POINT('Ctrl Pts',(1.31381795281002,-1.,-1.56496872402353));
#31524=CARTESIAN_POINT('Ctrl Pts',(1.31381795281002,1.,-1.56496872402353));
#31525=CARTESIAN_POINT('Ctrl Pts',(1.31558903860016,-1.,-1.57087397835723));
#31526=CARTESIAN_POINT('Ctrl Pts',(1.31558903860016,1.,-1.57087397835723));
#31527=CARTESIAN_POINT('Ctrl Pts',(1.31731642317187,-1.,-1.5768005650559));
#31528=CARTESIAN_POINT('Ctrl Pts',(1.31731642317187,1.,-1.5768005650559));
#31529=CARTESIAN_POINT('Ctrl Pts',(1.31900135021432,-1.,-1.58274907898834));
#31530=CARTESIAN_POINT('Ctrl Pts',(1.31900135021432,1.,-1.58274907898834));
#31531=CARTESIAN_POINT('Ctrl Pts',(1.32064537110892,-1.,-1.58872057258245));
#31532=CARTESIAN_POINT('Ctrl Pts',(1.32064537110892,1.,-1.58872057258245));
#31533=CARTESIAN_POINT('Ctrl Pts',(1.32224985747682,-1.,-1.59471591079403));
#31534=CARTESIAN_POINT('Ctrl Pts',(1.32224985747682,1.,-1.59471591079403));
#31535=CARTESIAN_POINT('Ctrl Pts',(1.32381550858256,-1.,-1.60073511858687));
#31536=CARTESIAN_POINT('Ctrl Pts',(1.32381550858256,1.,-1.60073511858687));
#31537=CARTESIAN_POINT('Ctrl Pts',(1.32534250785782,-1.,-1.60677758290954));
#31538=CARTESIAN_POINT('Ctrl Pts',(1.32534250785782,1.,-1.60677758290954));
#31539=CARTESIAN_POINT('Ctrl Pts',(1.32683074483356,-1.,-1.6128423401575));
#31540=CARTESIAN_POINT('Ctrl Pts',(1.32683074483356,1.,-1.6128423401575));
#31541=CARTESIAN_POINT('Ctrl Pts',(1.32828000610449,-1.,-1.61892832270724));
#31542=CARTESIAN_POINT('Ctrl Pts',(1.32828000610449,1.,-1.61892832270724));
#31543=CARTESIAN_POINT('Ctrl Pts',(1.3296901950568,-1.,-1.62503464209797));
#31544=CARTESIAN_POINT('Ctrl Pts',(1.3296901950568,1.,-1.62503464209797));
#31545=CARTESIAN_POINT('Ctrl Pts',(1.33106149345645,-1.,-1.63116079730923));
#31546=CARTESIAN_POINT('Ctrl Pts',(1.33106149345645,1.,-1.63116079730923));
#31547=CARTESIAN_POINT('Ctrl Pts',(1.33239425103724,-1.,-1.63730653475089));
#31548=CARTESIAN_POINT('Ctrl Pts',(1.33239425103724,1.,-1.63730653475089));
#31549=CARTESIAN_POINT('Ctrl Pts',(1.33368890676572,-1.,-1.6434717485603));
#31550=CARTESIAN_POINT('Ctrl Pts',(1.33368890676572,1.,-1.6434717485603));
#31551=CARTESIAN_POINT('Ctrl Pts',(1.33494590467993,-1.,-1.6496563728683));
#31552=CARTESIAN_POINT('Ctrl Pts',(1.33494590467993,1.,-1.6496563728683));
#31553=CARTESIAN_POINT('Ctrl Pts',(1.33616559745172,-1.,-1.65586025952593));
#31554=CARTESIAN_POINT('Ctrl Pts',(1.33616559745172,1.,-1.65586025952593));
#31555=CARTESIAN_POINT('Ctrl Pts',(1.33734820885262,-1.,-1.66208312541983));
#31556=CARTESIAN_POINT('Ctrl Pts',(1.33734820885262,1.,-1.66208312541983));
#31557=CARTESIAN_POINT('Ctrl Pts',(1.33849388654388,-1.,-1.66832460783989));
#31558=CARTESIAN_POINT('Ctrl Pts',(1.33849388654388,1.,-1.66832460783989));
#31559=CARTESIAN_POINT('Ctrl Pts',(1.3396027347034,-1.,-1.67458429426086));
#31560=CARTESIAN_POINT('Ctrl Pts',(1.3396027347034,1.,-1.67458429426086));
#31561=CARTESIAN_POINT('Ctrl Pts',(1.34067485185203,-1.,-1.68086176030362));
#31562=CARTESIAN_POINT('Ctrl Pts',(1.34067485185203,1.,-1.68086176030362));
#31563=CARTESIAN_POINT('Ctrl Pts',(1.341710374848,-1.,-1.68715660868764));
#31564=CARTESIAN_POINT('Ctrl Pts',(1.341710374848,1.,-1.68715660868764));
#31565=CARTESIAN_POINT('Ctrl Pts',(1.34270948206319,-1.,-1.6934684849687));
#31566=CARTESIAN_POINT('Ctrl Pts',(1.34270948206319,1.,-1.6934684849687));
#31567=CARTESIAN_POINT('Ctrl Pts',(1.34367237124483,-1.,-1.69979707754427));
#31568=CARTESIAN_POINT('Ctrl Pts',(1.34367237124483,1.,-1.69979707754427));
#31569=CARTESIAN_POINT('Ctrl Pts',(1.34459924533831,-1.,-1.70614212266738));
#31570=CARTESIAN_POINT('Ctrl Pts',(1.34459924533831,1.,-1.70614212266738));
#31571=CARTESIAN_POINT('Ctrl Pts',(1.34549029589416,-1.,-1.71250340686822));
#31572=CARTESIAN_POINT('Ctrl Pts',(1.34549029589416,1.,-1.71250340686822));
#31573=CARTESIAN_POINT('Ctrl Pts',(1.34634568653227,-1.,-1.7188807715049));
#31574=CARTESIAN_POINT('Ctrl Pts',(1.34634568653227,1.,-1.7188807715049));
#31575=CARTESIAN_POINT('Ctrl Pts',(1.34716554819527,-1.,-1.72527410680674));
#31576=CARTESIAN_POINT('Ctrl Pts',(1.34716554819527,1.,-1.72527410680674));
#31577=CARTESIAN_POINT('Ctrl Pts',(1.34779309152035,-1.,-1.7304014965394));
#31578=CARTESIAN_POINT('Ctrl Pts',(1.34779309152035,1.,-1.7304014965394));
#31579=CARTESIAN_POINT('Ctrl Pts',(1.34824783112887,-1.,-1.73425417885907));
#31580=CARTESIAN_POINT('Ctrl Pts',(1.34824783112887,1.,-1.73425417885907));
#31581=CARTESIAN_POINT('Ctrl Pts',(1.34854391898045,-1.,-1.73682580585691));
#31582=CARTESIAN_POINT('Ctrl Pts',(1.34854391898045,1.,-1.73682580585691));
#31583=CARTESIAN_POINT('Ctrl Pts',(1.34869019493419,-1.,-1.73811241238545));
#31584=CARTESIAN_POINT('Ctrl Pts',(1.34869019493419,1.,-1.73811241238545));
#31585=CARTESIAN_POINT('',(1.15624053661742,1.,-1.31362392696032));
#31586=CARTESIAN_POINT('Ctrl Pts',(1.15624053661742,1.,-1.31362392696032));
#31587=CARTESIAN_POINT('Ctrl Pts',(1.15950888730809,1.,-1.31722977216397));
#31588=CARTESIAN_POINT('Ctrl Pts',(1.16589330093588,1.,-1.32428080721772));
#31589=CARTESIAN_POINT('Ctrl Pts',(1.17501305789857,1.,-1.33437539347008));
#31590=CARTESIAN_POINT('Ctrl Pts',(1.18625865667441,1.,-1.34687054001093));
#31591=CARTESIAN_POINT('Ctrl Pts',(1.1987959077932,1.,-1.36088705043885));
#31592=CARTESIAN_POINT('Ctrl Pts',(1.20982812925645,1.,-1.37331915607905));
#31593=CARTESIAN_POINT('Ctrl Pts',(1.21938737280852,1.,-1.38420564527715));
#31594=CARTESIAN_POINT('Ctrl Pts',(1.22752961899387,1.,-1.39361389568796));
#31595=CARTESIAN_POINT('Ctrl Pts',(1.23434087290423,1.,-1.40164708206106));
#31596=CARTESIAN_POINT('Ctrl Pts',(1.23994455029534,1.,-1.40845295531283));
#31597=CARTESIAN_POINT('Ctrl Pts',(1.24450600513056,1.,-1.41422913175179));
#31598=CARTESIAN_POINT('Ctrl Pts',(1.24824430986571,1.,-1.41923722596025));
#31599=CARTESIAN_POINT('Ctrl Pts',(1.2514145557001,1.,-1.42378102115575));
#31600=CARTESIAN_POINT('Ctrl Pts',(1.25426945222639,1.,-1.42815938799387));
#31601=CARTESIAN_POINT('Ctrl Pts',(1.25702687965755,1.,-1.43262645609691));
#31602=CARTESIAN_POINT('Ctrl Pts',(1.25983531012005,1.,-1.43734919180848));
#31603=CARTESIAN_POINT('Ctrl Pts',(1.26273903323858,1.,-1.44236470511303));
#31604=CARTESIAN_POINT('Ctrl Pts',(1.26570925118868,1.,-1.44761985001662));
#31605=CARTESIAN_POINT('Ctrl Pts',(1.2686778680489,1.,-1.45301422764247));
#31606=CARTESIAN_POINT('Ctrl Pts',(1.27156805265289,1.,-1.45843906294697));
#31607=CARTESIAN_POINT('Ctrl Pts',(1.27433119897822,1.,-1.46382431332476));
#31608=CARTESIAN_POINT('Ctrl Pts',(1.27696414831089,1.,-1.46916035917133));
#31609=CARTESIAN_POINT('Ctrl Pts',(1.2794891824849,1.,-1.4744717526707));
#31610=CARTESIAN_POINT('Ctrl Pts',(1.28194158939517,1.,-1.47980070347096));
#31611=CARTESIAN_POINT('Ctrl Pts',(1.28435533880201,1.,-1.4851881711891));
#31612=CARTESIAN_POINT('Ctrl Pts',(1.2867467611644,1.,-1.4906522831278));
#31613=CARTESIAN_POINT('Ctrl Pts',(1.28911506584254,1.,-1.49618896881754));
#31614=CARTESIAN_POINT('Ctrl Pts',(1.29145022885181,1.,-1.50178230149776));
#31615=CARTESIAN_POINT('Ctrl Pts',(1.29373841372842,1.,-1.50741159078365));
#31616=CARTESIAN_POINT('Ctrl Pts',(1.29596850710509,1.,-1.51305994241402));
#31617=CARTESIAN_POINT('Ctrl Pts',(1.29813791800747,1.,-1.51872184912724));
#31618=CARTESIAN_POINT('Ctrl Pts',(1.30024984366328,1.,-1.52439957861062));
#31619=CARTESIAN_POINT('Ctrl Pts',(1.30231064395568,1.,-1.53009970283891));
#31620=CARTESIAN_POINT('Ctrl Pts',(1.30432735639489,1.,-1.53582981268977));
#31621=CARTESIAN_POINT('Ctrl Pts',(1.30630475189556,1.,-1.54159462645432));
#31622=CARTESIAN_POINT('Ctrl Pts',(1.30824393907473,1.,-1.54739413957185));
#31623=CARTESIAN_POINT('Ctrl Pts',(1.31014393684222,1.,-1.55322568759481));
#31624=CARTESIAN_POINT('Ctrl Pts',(1.31200264341696,1.,-1.55908521254821));
#31625=CARTESIAN_POINT('Ctrl Pts',(1.31381795281002,1.,-1.56496872402353));
#31626=CARTESIAN_POINT('Ctrl Pts',(1.31558903860016,1.,-1.57087397835723));
#31627=CARTESIAN_POINT('Ctrl Pts',(1.31731642317187,1.,-1.5768005650559));
#31628=CARTESIAN_POINT('Ctrl Pts',(1.31900135021432,1.,-1.58274907898834));
#31629=CARTESIAN_POINT('Ctrl Pts',(1.32064537110892,1.,-1.58872057258245));
#31630=CARTESIAN_POINT('Ctrl Pts',(1.32224985747682,1.,-1.59471591079403));
#31631=CARTESIAN_POINT('Ctrl Pts',(1.32381550858256,1.,-1.60073511858687));
#31632=CARTESIAN_POINT('Ctrl Pts',(1.32534250785782,1.,-1.60677758290954));
#31633=CARTESIAN_POINT('Ctrl Pts',(1.32683074483356,1.,-1.6128423401575));
#31634=CARTESIAN_POINT('Ctrl Pts',(1.32828000610449,1.,-1.61892832270724));
#31635=CARTESIAN_POINT('Ctrl Pts',(1.3296901950568,1.,-1.62503464209797));
#31636=CARTESIAN_POINT('Ctrl Pts',(1.33106149345645,1.,-1.63116079730923));
#31637=CARTESIAN_POINT('Ctrl Pts',(1.33239425103724,1.,-1.63730653475089));
#31638=CARTESIAN_POINT('Ctrl Pts',(1.33368890676572,1.,-1.6434717485603));
#31639=CARTESIAN_POINT('Ctrl Pts',(1.33494590467993,1.,-1.6496563728683));
#31640=CARTESIAN_POINT('Ctrl Pts',(1.33616559745172,1.,-1.65586025952593));
#31641=CARTESIAN_POINT('Ctrl Pts',(1.33734820885262,1.,-1.66208312541983));
#31642=CARTESIAN_POINT('Ctrl Pts',(1.33849388654388,1.,-1.66832460783989));
#31643=CARTESIAN_POINT('Ctrl Pts',(1.3396027347034,1.,-1.67458429426086));
#31644=CARTESIAN_POINT('Ctrl Pts',(1.34067485185203,1.,-1.68086176030362));
#31645=CARTESIAN_POINT('Ctrl Pts',(1.341710374848,1.,-1.68715660868764));
#31646=CARTESIAN_POINT('Ctrl Pts',(1.34270948206319,1.,-1.6934684849687));
#31647=CARTESIAN_POINT('Ctrl Pts',(1.34367237124483,1.,-1.69979707754427));
#31648=CARTESIAN_POINT('Ctrl Pts',(1.34459924533831,1.,-1.70614212266738));
#31649=CARTESIAN_POINT('Ctrl Pts',(1.34549029589416,1.,-1.71250340686822));
#31650=CARTESIAN_POINT('Ctrl Pts',(1.34634568653227,1.,-1.7188807715049));
#31651=CARTESIAN_POINT('Ctrl Pts',(1.34716554819527,1.,-1.72527410680674));
#31652=CARTESIAN_POINT('Ctrl Pts',(1.34779309152035,1.,-1.7304014965394));
#31653=CARTESIAN_POINT('Ctrl Pts',(1.34824783112887,1.,-1.73425417885907));
#31654=CARTESIAN_POINT('Ctrl Pts',(1.34854391898045,1.,-1.73682580585691));
#31655=CARTESIAN_POINT('Ctrl Pts',(1.34869019493419,1.,-1.73811241238545));
#31656=CARTESIAN_POINT('',(1.15624053661742,0.,-1.31362392696032));
#31657=CARTESIAN_POINT('Origin',(0.,0.,0.));
#31658=CARTESIAN_POINT('',(1.31362392696032,1.,-1.15624053661742));
#31659=CARTESIAN_POINT('Origin',(0.,1.,0.));
#31660=CARTESIAN_POINT('',(1.31362392696032,0.,-1.15624053661742));
#31661=CARTESIAN_POINT('Ctrl Pts',(1.73811241238545,-1.,-1.34869019493419));
#31662=CARTESIAN_POINT('Ctrl Pts',(1.73811241238545,1.,-1.34869019493419));
#31663=CARTESIAN_POINT('Ctrl Pts',(1.73682580585819,-1.,-1.34854391898145));
#31664=CARTESIAN_POINT('Ctrl Pts',(1.73682580585819,1.,-1.34854391898145));
#31665=CARTESIAN_POINT('Ctrl Pts',(1.73425417886254,-1.,-1.34824783113158));
#31666=CARTESIAN_POINT('Ctrl Pts',(1.73425417886254,1.,-1.34824783113158));
#31667=CARTESIAN_POINT('Ctrl Pts',(1.73040149654497,-1.,-1.3477930915247));
#31668=CARTESIAN_POINT('Ctrl Pts',(1.73040149654497,1.,-1.3477930915247));
#31669=CARTESIAN_POINT('Ctrl Pts',(1.72527410681298,-1.,-1.34716554820013));
#31670=CARTESIAN_POINT('Ctrl Pts',(1.72527410681298,1.,-1.34716554820013));
#31671=CARTESIAN_POINT('Ctrl Pts',(1.7188807715095,-1.,-1.34634568653586));
#31672=CARTESIAN_POINT('Ctrl Pts',(1.7188807715095,1.,-1.34634568653586));
#31673=CARTESIAN_POINT('Ctrl Pts',(1.71250340687011,-1.,-1.34549029589563));
#31674=CARTESIAN_POINT('Ctrl Pts',(1.71250340687011,1.,-1.34549029589563));
#31675=CARTESIAN_POINT('Ctrl Pts',(1.70614212266676,-1.,-1.34459924533783));
#31676=CARTESIAN_POINT('Ctrl Pts',(1.70614212266676,1.,-1.34459924533783));
#31677=CARTESIAN_POINT('Ctrl Pts',(1.69979707754221,-1.,-1.34367237124322));
#31678=CARTESIAN_POINT('Ctrl Pts',(1.69979707754221,1.,-1.34367237124322));
#31679=CARTESIAN_POINT('Ctrl Pts',(1.6934684849664,-1.,-1.34270948206139));
#31680=CARTESIAN_POINT('Ctrl Pts',(1.6934684849664,1.,-1.34270948206139));
#31681=CARTESIAN_POINT('Ctrl Pts',(1.68715660868602,-1.,-1.34171037484673));
#31682=CARTESIAN_POINT('Ctrl Pts',(1.68715660868602,1.,-1.34171037484673));
#31683=CARTESIAN_POINT('Ctrl Pts',(1.68086176030308,-1.,-1.3406748518516));
#31684=CARTESIAN_POINT('Ctrl Pts',(1.68086176030308,1.,-1.3406748518516));
#31685=CARTESIAN_POINT('Ctrl Pts',(1.67458429426126,-1.,-1.33960273470372));
#31686=CARTESIAN_POINT('Ctrl Pts',(1.67458429426126,1.,-1.33960273470372));
#31687=CARTESIAN_POINT('Ctrl Pts',(1.66832460784078,-1.,-1.33849388654458));
#31688=CARTESIAN_POINT('Ctrl Pts',(1.66832460784078,1.,-1.33849388654458));
#31689=CARTESIAN_POINT('Ctrl Pts',(1.66208312542073,-1.,-1.33734820885331));
#31690=CARTESIAN_POINT('Ctrl Pts',(1.66208312542073,1.,-1.33734820885331));
#31691=CARTESIAN_POINT('Ctrl Pts',(1.65586025952651,-1.,-1.33616559745217));
#31692=CARTESIAN_POINT('Ctrl Pts',(1.65586025952651,1.,-1.33616559745217));
#31693=CARTESIAN_POINT('Ctrl Pts',(1.64965637286843,-1.,-1.33494590468003));
#31694=CARTESIAN_POINT('Ctrl Pts',(1.64965637286843,1.,-1.33494590468003));
#31695=CARTESIAN_POINT('Ctrl Pts',(1.64347174856007,-1.,-1.33368890676554));
#31696=CARTESIAN_POINT('Ctrl Pts',(1.64347174856007,1.,-1.33368890676554));
#31697=CARTESIAN_POINT('Ctrl Pts',(1.63730653475049,-1.,-1.33239425103694));
#31698=CARTESIAN_POINT('Ctrl Pts',(1.63730653475049,1.,-1.33239425103694));
#31699=CARTESIAN_POINT('Ctrl Pts',(1.63116079730887,-1.,-1.33106149345618));
#31700=CARTESIAN_POINT('Ctrl Pts',(1.63116079730887,1.,-1.33106149345618));
#31701=CARTESIAN_POINT('Ctrl Pts',(1.62503464209777,-1.,-1.32969019505665));
#31702=CARTESIAN_POINT('Ctrl Pts',(1.62503464209777,1.,-1.32969019505665));
#31703=CARTESIAN_POINT('Ctrl Pts',(1.61892832270723,-1.,-1.32828000610448));
#31704=CARTESIAN_POINT('Ctrl Pts',(1.61892832270723,1.,-1.32828000610448));
#31705=CARTESIAN_POINT('Ctrl Pts',(1.61284234015762,-1.,-1.32683074483365));
#31706=CARTESIAN_POINT('Ctrl Pts',(1.61284234015762,1.,-1.32683074483365));
#31707=CARTESIAN_POINT('Ctrl Pts',(1.6067775829097,-1.,-1.32534250785794));
#31708=CARTESIAN_POINT('Ctrl Pts',(1.6067775829097,1.,-1.32534250785794));
#31709=CARTESIAN_POINT('Ctrl Pts',(1.600735118587,-1.,-1.32381550858266));
#31710=CARTESIAN_POINT('Ctrl Pts',(1.600735118587,1.,-1.32381550858266));
#31711=CARTESIAN_POINT('Ctrl Pts',(1.59471591079408,-1.,-1.32224985747686));
#31712=CARTESIAN_POINT('Ctrl Pts',(1.59471591079408,1.,-1.32224985747686));
#31713=CARTESIAN_POINT('Ctrl Pts',(1.58872057258244,-1.,-1.32064537110891));
#31714=CARTESIAN_POINT('Ctrl Pts',(1.58872057258244,1.,-1.32064537110891));
#31715=CARTESIAN_POINT('Ctrl Pts',(1.58274907898829,-1.,-1.31900135021428));
#31716=CARTESIAN_POINT('Ctrl Pts',(1.58274907898829,1.,-1.31900135021428));
#31717=CARTESIAN_POINT('Ctrl Pts',(1.57680056505585,-1.,-1.31731642317183));
#31718=CARTESIAN_POINT('Ctrl Pts',(1.57680056505585,1.,-1.31731642317183));
#31719=CARTESIAN_POINT('Ctrl Pts',(1.57087397835721,-1.,-1.31558903860015));
#31720=CARTESIAN_POINT('Ctrl Pts',(1.57087397835721,1.,-1.31558903860015));
#31721=CARTESIAN_POINT('Ctrl Pts',(1.56496872402352,-1.,-1.31381795281002));
#31722=CARTESIAN_POINT('Ctrl Pts',(1.56496872402352,1.,-1.31381795281002));
#31723=CARTESIAN_POINT('Ctrl Pts',(1.55908521254822,-1.,-1.31200264341696));
#31724=CARTESIAN_POINT('Ctrl Pts',(1.55908521254822,1.,-1.31200264341696));
#31725=CARTESIAN_POINT('Ctrl Pts',(1.55322568759481,-1.,-1.31014393684221));
#31726=CARTESIAN_POINT('Ctrl Pts',(1.55322568759481,1.,-1.31014393684221));
#31727=CARTESIAN_POINT('Ctrl Pts',(1.54739413957183,-1.,-1.30824393907471));
#31728=CARTESIAN_POINT('Ctrl Pts',(1.54739413957183,1.,-1.30824393907471));
#31729=CARTESIAN_POINT('Ctrl Pts',(1.54159462645428,-1.,-1.30630475189553));
#31730=CARTESIAN_POINT('Ctrl Pts',(1.54159462645428,1.,-1.30630475189553));
#31731=CARTESIAN_POINT('Ctrl Pts',(1.53582981268976,-1.,-1.30432735639487));
#31732=CARTESIAN_POINT('Ctrl Pts',(1.53582981268976,1.,-1.30432735639487));
#31733=CARTESIAN_POINT('Ctrl Pts',(1.53009970283893,-1.,-1.3023106439557));
#31734=CARTESIAN_POINT('Ctrl Pts',(1.53009970283893,1.,-1.3023106439557));
#31735=CARTESIAN_POINT('Ctrl Pts',(1.5243995786107,-1.,-1.30024984366334));
#31736=CARTESIAN_POINT('Ctrl Pts',(1.5243995786107,1.,-1.30024984366334));
#31737=CARTESIAN_POINT('Ctrl Pts',(1.51872184912735,-1.,-1.29813791800757));
#31738=CARTESIAN_POINT('Ctrl Pts',(1.51872184912735,1.,-1.29813791800757));
#31739=CARTESIAN_POINT('Ctrl Pts',(1.51305994241412,-1.,-1.29596850710518));
#31740=CARTESIAN_POINT('Ctrl Pts',(1.51305994241412,1.,-1.29596850710518));
#31741=CARTESIAN_POINT('Ctrl Pts',(1.50741159078367,-1.,-1.29373841372843));
#31742=CARTESIAN_POINT('Ctrl Pts',(1.50741159078367,1.,-1.29373841372843));
#31743=CARTESIAN_POINT('Ctrl Pts',(1.50178230149764,-1.,-1.29145022885171));
#31744=CARTESIAN_POINT('Ctrl Pts',(1.50178230149764,1.,-1.29145022885171));
#31745=CARTESIAN_POINT('Ctrl Pts',(1.49618896881729,-1.,-1.28911506584232));
#31746=CARTESIAN_POINT('Ctrl Pts',(1.49618896881729,1.,-1.28911506584232));
#31747=CARTESIAN_POINT('Ctrl Pts',(1.4906522831275,-1.,-1.28674676116415));
#31748=CARTESIAN_POINT('Ctrl Pts',(1.4906522831275,1.,-1.28674676116415));
#31749=CARTESIAN_POINT('Ctrl Pts',(1.48518817118891,-1.,-1.28435533880184));
#31750=CARTESIAN_POINT('Ctrl Pts',(1.48518817118891,1.,-1.28435533880184));
#31751=CARTESIAN_POINT('Ctrl Pts',(1.47980070347102,-1.,-1.28194158939522));
#31752=CARTESIAN_POINT('Ctrl Pts',(1.47980070347102,1.,-1.28194158939522));
#31753=CARTESIAN_POINT('Ctrl Pts',(1.4744717526711,-1.,-1.27948918248524));
#31754=CARTESIAN_POINT('Ctrl Pts',(1.4744717526711,1.,-1.27948918248524));
#31755=CARTESIAN_POINT('Ctrl Pts',(1.46916035917197,-1.,-1.27696414831144));
#31756=CARTESIAN_POINT('Ctrl Pts',(1.46916035917197,1.,-1.27696414831144));
#31757=CARTESIAN_POINT('Ctrl Pts',(1.4638243133254,-1.,-1.27433119897877));
#31758=CARTESIAN_POINT('Ctrl Pts',(1.4638243133254,1.,-1.27433119897877));
#31759=CARTESIAN_POINT('Ctrl Pts',(1.45843906294725,-1.,-1.27156805265312));
#31760=CARTESIAN_POINT('Ctrl Pts',(1.45843906294725,1.,-1.27156805265312));
#31761=CARTESIAN_POINT('Ctrl Pts',(1.45301422764205,-1.,-1.26867786804854));
#31762=CARTESIAN_POINT('Ctrl Pts',(1.45301422764205,1.,-1.26867786804854));
#31763=CARTESIAN_POINT('Ctrl Pts',(1.44761985001544,-1.,-1.26570925118767));
#31764=CARTESIAN_POINT('Ctrl Pts',(1.44761985001544,1.,-1.26570925118767));
#31765=CARTESIAN_POINT('Ctrl Pts',(1.44236470511145,-1.,-1.26273903323723));
#31766=CARTESIAN_POINT('Ctrl Pts',(1.44236470511145,1.,-1.26273903323723));
#31767=CARTESIAN_POINT('Ctrl Pts',(1.43734919180719,-1.,-1.25983531011894));
#31768=CARTESIAN_POINT('Ctrl Pts',(1.43734919180719,1.,-1.25983531011894));
#31769=CARTESIAN_POINT('Ctrl Pts',(1.43262645609679,-1.,-1.25702687965744));
#31770=CARTESIAN_POINT('Ctrl Pts',(1.43262645609679,1.,-1.25702687965744));
#31771=CARTESIAN_POINT('Ctrl Pts',(1.42815938799555,-1.,-1.25426945222783));
#31772=CARTESIAN_POINT('Ctrl Pts',(1.42815938799555,1.,-1.25426945222783));
#31773=CARTESIAN_POINT('Ctrl Pts',(1.42378102115911,-1.,-1.25141455570299));
#31774=CARTESIAN_POINT('Ctrl Pts',(1.42378102115911,1.,-1.25141455570299));
#31775=CARTESIAN_POINT('Ctrl Pts',(1.41923722596421,-1.,-1.24824430986911));
#31776=CARTESIAN_POINT('Ctrl Pts',(1.41923722596421,1.,-1.24824430986911));
#31777=CARTESIAN_POINT('Ctrl Pts',(1.41422913175437,-1.,-1.24450600513278));
#31778=CARTESIAN_POINT('Ctrl Pts',(1.41422913175437,1.,-1.24450600513278));
#31779=CARTESIAN_POINT('Ctrl Pts',(1.40845295531151,-1.,-1.23994455029421));
#31780=CARTESIAN_POINT('Ctrl Pts',(1.40845295531151,1.,-1.23994455029421));
#31781=CARTESIAN_POINT('Ctrl Pts',(1.40164708205345,-1.,-1.23434087289768));
#31782=CARTESIAN_POINT('Ctrl Pts',(1.40164708205345,1.,-1.23434087289768));
#31783=CARTESIAN_POINT('Ctrl Pts',(1.39361389567257,-1.,-1.22752961898063));
#31784=CARTESIAN_POINT('Ctrl Pts',(1.39361389567257,1.,-1.22752961898063));
#31785=CARTESIAN_POINT('Ctrl Pts',(1.38420564525391,-1.,-1.21938737278853));
#31786=CARTESIAN_POINT('Ctrl Pts',(1.38420564525391,1.,-1.21938737278853));
#31787=CARTESIAN_POINT('Ctrl Pts',(1.37331915604962,-1.,-1.20982812923113));
#31788=CARTESIAN_POINT('Ctrl Pts',(1.37331915604962,1.,-1.20982812923113));
#31789=CARTESIAN_POINT('Ctrl Pts',(1.36088705040677,-1.,-1.1987959077656));
#31790=CARTESIAN_POINT('Ctrl Pts',(1.36088705040677,1.,-1.1987959077656));
#31791=CARTESIAN_POINT('Ctrl Pts',(1.34687053998157,-1.,-1.18625865664915));
#31792=CARTESIAN_POINT('Ctrl Pts',(1.34687053998157,1.,-1.18625865664915));
#31793=CARTESIAN_POINT('Ctrl Pts',(1.33437539344842,-1.,-1.17501305787994));
#31794=CARTESIAN_POINT('Ctrl Pts',(1.33437539344842,1.,-1.17501305787994));
#31795=CARTESIAN_POINT('Ctrl Pts',(1.32428080720544,-1.,-1.16589330092532));
#31796=CARTESIAN_POINT('Ctrl Pts',(1.32428080720544,1.,-1.16589330092532));
#31797=CARTESIAN_POINT('Ctrl Pts',(1.3172297721596,-1.,-1.15950888730433));
#31798=CARTESIAN_POINT('Ctrl Pts',(1.3172297721596,1.,-1.15950888730433));
#31799=CARTESIAN_POINT('Ctrl Pts',(1.31362392696032,-1.,-1.15624053661742));
#31800=CARTESIAN_POINT('Ctrl Pts',(1.31362392696032,1.,-1.15624053661742));
#31801=CARTESIAN_POINT('',(1.73811241238545,1.,-1.34869019493419));
#31802=CARTESIAN_POINT('Ctrl Pts',(1.73811241238545,1.,-1.34869019493419));
#31803=CARTESIAN_POINT('Ctrl Pts',(1.73682580585819,1.,-1.34854391898145));
#31804=CARTESIAN_POINT('Ctrl Pts',(1.73425417886254,1.,-1.34824783113158));
#31805=CARTESIAN_POINT('Ctrl Pts',(1.73040149654497,1.,-1.3477930915247));
#31806=CARTESIAN_POINT('Ctrl Pts',(1.72527410681298,1.,-1.34716554820013));
#31807=CARTESIAN_POINT('Ctrl Pts',(1.7188807715095,1.,-1.34634568653586));
#31808=CARTESIAN_POINT('Ctrl Pts',(1.71250340687011,1.,-1.34549029589563));
#31809=CARTESIAN_POINT('Ctrl Pts',(1.70614212266676,1.,-1.34459924533783));
#31810=CARTESIAN_POINT('Ctrl Pts',(1.69979707754221,1.,-1.34367237124322));
#31811=CARTESIAN_POINT('Ctrl Pts',(1.6934684849664,1.,-1.34270948206139));
#31812=CARTESIAN_POINT('Ctrl Pts',(1.68715660868602,1.,-1.34171037484673));
#31813=CARTESIAN_POINT('Ctrl Pts',(1.68086176030308,1.,-1.3406748518516));
#31814=CARTESIAN_POINT('Ctrl Pts',(1.67458429426126,1.,-1.33960273470372));
#31815=CARTESIAN_POINT('Ctrl Pts',(1.66832460784078,1.,-1.33849388654458));
#31816=CARTESIAN_POINT('Ctrl Pts',(1.66208312542073,1.,-1.33734820885331));
#31817=CARTESIAN_POINT('Ctrl Pts',(1.65586025952651,1.,-1.33616559745217));
#31818=CARTESIAN_POINT('Ctrl Pts',(1.64965637286843,1.,-1.33494590468003));
#31819=CARTESIAN_POINT('Ctrl Pts',(1.64347174856007,1.,-1.33368890676554));
#31820=CARTESIAN_POINT('Ctrl Pts',(1.63730653475049,1.,-1.33239425103694));
#31821=CARTESIAN_POINT('Ctrl Pts',(1.63116079730887,1.,-1.33106149345618));
#31822=CARTESIAN_POINT('Ctrl Pts',(1.62503464209777,1.,-1.32969019505665));
#31823=CARTESIAN_POINT('Ctrl Pts',(1.61892832270723,1.,-1.32828000610448));
#31824=CARTESIAN_POINT('Ctrl Pts',(1.61284234015762,1.,-1.32683074483365));
#31825=CARTESIAN_POINT('Ctrl Pts',(1.6067775829097,1.,-1.32534250785794));
#31826=CARTESIAN_POINT('Ctrl Pts',(1.600735118587,1.,-1.32381550858266));
#31827=CARTESIAN_POINT('Ctrl Pts',(1.59471591079408,1.,-1.32224985747686));
#31828=CARTESIAN_POINT('Ctrl Pts',(1.58872057258244,1.,-1.32064537110891));
#31829=CARTESIAN_POINT('Ctrl Pts',(1.58274907898829,1.,-1.31900135021428));
#31830=CARTESIAN_POINT('Ctrl Pts',(1.57680056505585,1.,-1.31731642317183));
#31831=CARTESIAN_POINT('Ctrl Pts',(1.57087397835721,1.,-1.31558903860015));
#31832=CARTESIAN_POINT('Ctrl Pts',(1.56496872402352,1.,-1.31381795281002));
#31833=CARTESIAN_POINT('Ctrl Pts',(1.55908521254822,1.,-1.31200264341696));
#31834=CARTESIAN_POINT('Ctrl Pts',(1.55322568759481,1.,-1.31014393684221));
#31835=CARTESIAN_POINT('Ctrl Pts',(1.54739413957183,1.,-1.30824393907471));
#31836=CARTESIAN_POINT('Ctrl Pts',(1.54159462645428,1.,-1.30630475189553));
#31837=CARTESIAN_POINT('Ctrl Pts',(1.53582981268976,1.,-1.30432735639487));
#31838=CARTESIAN_POINT('Ctrl Pts',(1.53009970283893,1.,-1.3023106439557));
#31839=CARTESIAN_POINT('Ctrl Pts',(1.5243995786107,1.,-1.30024984366334));
#31840=CARTESIAN_POINT('Ctrl Pts',(1.51872184912735,1.,-1.29813791800757));
#31841=CARTESIAN_POINT('Ctrl Pts',(1.51305994241412,1.,-1.29596850710518));
#31842=CARTESIAN_POINT('Ctrl Pts',(1.50741159078367,1.,-1.29373841372843));
#31843=CARTESIAN_POINT('Ctrl Pts',(1.50178230149764,1.,-1.29145022885171));
#31844=CARTESIAN_POINT('Ctrl Pts',(1.49618896881729,1.,-1.28911506584232));
#31845=CARTESIAN_POINT('Ctrl Pts',(1.4906522831275,1.,-1.28674676116415));
#31846=CARTESIAN_POINT('Ctrl Pts',(1.48518817118891,1.,-1.28435533880184));
#31847=CARTESIAN_POINT('Ctrl Pts',(1.47980070347102,1.,-1.28194158939522));
#31848=CARTESIAN_POINT('Ctrl Pts',(1.4744717526711,1.,-1.27948918248524));
#31849=CARTESIAN_POINT('Ctrl Pts',(1.46916035917197,1.,-1.27696414831144));
#31850=CARTESIAN_POINT('Ctrl Pts',(1.4638243133254,1.,-1.27433119897877));
#31851=CARTESIAN_POINT('Ctrl Pts',(1.45843906294725,1.,-1.27156805265312));
#31852=CARTESIAN_POINT('Ctrl Pts',(1.45301422764205,1.,-1.26867786804854));
#31853=CARTESIAN_POINT('Ctrl Pts',(1.44761985001544,1.,-1.26570925118767));
#31854=CARTESIAN_POINT('Ctrl Pts',(1.44236470511145,1.,-1.26273903323723));
#31855=CARTESIAN_POINT('Ctrl Pts',(1.43734919180719,1.,-1.25983531011894));
#31856=CARTESIAN_POINT('Ctrl Pts',(1.43262645609679,1.,-1.25702687965744));
#31857=CARTESIAN_POINT('Ctrl Pts',(1.42815938799555,1.,-1.25426945222783));
#31858=CARTESIAN_POINT('Ctrl Pts',(1.42378102115911,1.,-1.25141455570299));
#31859=CARTESIAN_POINT('Ctrl Pts',(1.41923722596421,1.,-1.24824430986911));
#31860=CARTESIAN_POINT('Ctrl Pts',(1.41422913175437,1.,-1.24450600513278));
#31861=CARTESIAN_POINT('Ctrl Pts',(1.40845295531151,1.,-1.23994455029421));
#31862=CARTESIAN_POINT('Ctrl Pts',(1.40164708205345,1.,-1.23434087289768));
#31863=CARTESIAN_POINT('Ctrl Pts',(1.39361389567257,1.,-1.22752961898063));
#31864=CARTESIAN_POINT('Ctrl Pts',(1.38420564525391,1.,-1.21938737278853));
#31865=CARTESIAN_POINT('Ctrl Pts',(1.37331915604962,1.,-1.20982812923113));
#31866=CARTESIAN_POINT('Ctrl Pts',(1.36088705040677,1.,-1.1987959077656));
#31867=CARTESIAN_POINT('Ctrl Pts',(1.34687053998157,1.,-1.18625865664915));
#31868=CARTESIAN_POINT('Ctrl Pts',(1.33437539344842,1.,-1.17501305787994));
#31869=CARTESIAN_POINT('Ctrl Pts',(1.32428080720544,1.,-1.16589330092532));
#31870=CARTESIAN_POINT('Ctrl Pts',(1.3172297721596,1.,-1.15950888730433));
#31871=CARTESIAN_POINT('Ctrl Pts',(1.31362392696032,1.,-1.15624053661742));
#31872=CARTESIAN_POINT('',(1.73811241238545,0.,-1.34869019493419));
#31873=CARTESIAN_POINT('Origin',(1.81978687191668,0.,-1.23627494547115));
#31874=CARTESIAN_POINT('',(1.81978687191668,1.,-1.23627494547115));
#31875=CARTESIAN_POINT('',(1.73811241238545,1.,-1.34869019493419));
#31876=CARTESIAN_POINT('',(1.81978687191668,0.,-1.23627494547115));
#31877=CARTESIAN_POINT('Ctrl Pts',(1.5055822144029,-1.,-0.892032620296855));
#31878=CARTESIAN_POINT('Ctrl Pts',(1.5055822144029,1.,-0.892032620296855));
#31879=CARTESIAN_POINT('Ctrl Pts',(1.50980486807181,-1.,-0.894452006967538));
#31880=CARTESIAN_POINT('Ctrl Pts',(1.50980486807181,1.,-0.894452006967538));
#31881=CARTESIAN_POINT('Ctrl Pts',(1.51805569591479,-1.,-0.89918504749193));
#31882=CARTESIAN_POINT('Ctrl Pts',(1.51805569591479,1.,-0.89918504749193));
#31883=CARTESIAN_POINT('Ctrl Pts',(1.52984849890434,-1.,-0.905967409640499));
#31884=CARTESIAN_POINT('Ctrl Pts',(1.52984849890434,1.,-0.905967409640499));
#31885=CARTESIAN_POINT('Ctrl Pts',(1.54440491152807,-1.,-0.91437591904658));
#31886=CARTESIAN_POINT('Ctrl Pts',(1.54440491152807,1.,-0.91437591904658));
#31887=CARTESIAN_POINT('Ctrl Pts',(1.56065988582509,-1.,-0.923832188966322));
#31888=CARTESIAN_POINT('Ctrl Pts',(1.56065988582509,1.,-0.923832188966322));
#31889=CARTESIAN_POINT('Ctrl Pts',(1.57499388385561,-1.,-0.932246680128849));
#31890=CARTESIAN_POINT('Ctrl Pts',(1.57499388385561,1.,-0.932246680128849));
#31891=CARTESIAN_POINT('Ctrl Pts',(1.58744937489796,-1.,-0.939646377909319));
#31892=CARTESIAN_POINT('Ctrl Pts',(1.58744937489796,1.,-0.939646377909319));
#31893=CARTESIAN_POINT('Ctrl Pts',(1.59810042045408,-1.,-0.946078063325796));
#31894=CARTESIAN_POINT('Ctrl Pts',(1.59810042045408,1.,-0.946078063325796));
#31895=CARTESIAN_POINT('Ctrl Pts',(1.60706069897794,-1.,-0.951613284361248));
#31896=CARTESIAN_POINT('Ctrl Pts',(1.60706069897794,1.,-0.951613284361248));
#31897=CARTESIAN_POINT('Ctrl Pts',(1.61449324337233,-1.,-0.956354422921573));
#31898=CARTESIAN_POINT('Ctrl Pts',(1.61449324337233,1.,-0.956354422921573));
#31899=CARTESIAN_POINT('Ctrl Pts',(1.62061638139929,-1.,-0.960438326099958));
#31900=CARTESIAN_POINT('Ctrl Pts',(1.62061638139929,1.,-0.960438326099958));
#31901=CARTESIAN_POINT('Ctrl Pts',(1.6257193066974,-1.,-0.964046107037821));
#31902=CARTESIAN_POINT('Ctrl Pts',(1.6257193066974,1.,-0.964046107037821));
#31903=CARTESIAN_POINT('Ctrl Pts',(1.63013849959083,-1.,-0.967387853228041));
#31904=CARTESIAN_POINT('Ctrl Pts',(1.63013849959083,1.,-0.967387853228041));
#31905=CARTESIAN_POINT('Ctrl Pts',(1.63420665729609,-1.,-0.970669715996356));
#31906=CARTESIAN_POINT('Ctrl Pts',(1.63420665729609,1.,-0.970669715996356));
#31907=CARTESIAN_POINT('Ctrl Pts',(1.63820952658157,-1.,-0.974066058287501));
#31908=CARTESIAN_POINT('Ctrl Pts',(1.63820952658157,1.,-0.974066058287501));
#31909=CARTESIAN_POINT('Ctrl Pts',(1.64233990826831,-1.,-0.977689794120297));
#31910=CARTESIAN_POINT('Ctrl Pts',(1.64233990826831,1.,-0.977689794120297));
#31911=CARTESIAN_POINT('Ctrl Pts',(1.64665139190834,-1.,-0.981562530940574));
#31912=CARTESIAN_POINT('Ctrl Pts',(1.64665139190834,1.,-0.981562530940574));
#31913=CARTESIAN_POINT('Ctrl Pts',(1.6511001661277,-1.,-0.985642622921626));
#31914=CARTESIAN_POINT('Ctrl Pts',(1.6511001661277,1.,-0.985642622921626));
#31915=CARTESIAN_POINT('Ctrl Pts',(1.65559044289746,-1.,-0.98985562785445));
#31916=CARTESIAN_POINT('Ctrl Pts',(1.65559044289746,1.,-0.98985562785445));
#31917=CARTESIAN_POINT('Ctrl Pts',(1.66001553809916,-1.,-0.994121836661116));
#31918=CARTESIAN_POINT('Ctrl Pts',(1.66001553809916,1.,-0.994121836661116));
#31919=CARTESIAN_POINT('Ctrl Pts',(1.66430758030304,-1.,-0.998389654952317));
#31920=CARTESIAN_POINT('Ctrl Pts',(1.66430758030304,1.,-0.998389654952317));
#31921=CARTESIAN_POINT('Ctrl Pts',(1.66846059277231,-1.,-1.00265091003682));
#31922=CARTESIAN_POINT('Ctrl Pts',(1.66846059277231,1.,-1.00265091003682));
#31923=CARTESIAN_POINT('Ctrl Pts',(1.67250335383248,-1.,-1.00692206696387));
#31924=CARTESIAN_POINT('Ctrl Pts',(1.67250335383248,1.,-1.00692206696387));
#31925=CARTESIAN_POINT('Ctrl Pts',(1.67648246776457,-1.,-1.01123236493507));
#31926=CARTESIAN_POINT('Ctrl Pts',(1.67648246776457,1.,-1.01123236493507));
#31927=CARTESIAN_POINT('Ctrl Pts',(1.6804428989482,-1.,-1.01561026162787));
#31928=CARTESIAN_POINT('Ctrl Pts',(1.6804428989482,1.,-1.01561026162787));
#31929=CARTESIAN_POINT('Ctrl Pts',(1.68440578021739,-1.,-1.02006795074222));
#31930=CARTESIAN_POINT('Ctrl Pts',(1.68440578021739,1.,-1.02006795074222));
#31931=CARTESIAN_POINT('Ctrl Pts',(1.68836910178475,-1.,-1.02460180535272));
#31932=CARTESIAN_POINT('Ctrl Pts',(1.68836910178475,1.,-1.02460180535272));
#31933=CARTESIAN_POINT('Ctrl Pts',(1.69231840863471,-1.,-1.02919977579155));
#31934=CARTESIAN_POINT('Ctrl Pts',(1.69231840863471,1.,-1.02919977579155));
#31935=CARTESIAN_POINT('Ctrl Pts',(1.69623414782769,-1.,-1.03384646003587));
#31936=CARTESIAN_POINT('Ctrl Pts',(1.69623414782769,1.,-1.03384646003587));
#31937=CARTESIAN_POINT('Ctrl Pts',(1.70010052930951,-1.,-1.03852922490782));
#31938=CARTESIAN_POINT('Ctrl Pts',(1.70010052930951,1.,-1.03852922490782));
#31939=CARTESIAN_POINT('Ctrl Pts',(1.70391338707969,-1.,-1.04324363334546));
#31940=CARTESIAN_POINT('Ctrl Pts',(1.70391338707969,1.,-1.04324363334546));
#31941=CARTESIAN_POINT('Ctrl Pts',(1.70767646263641,-1.,-1.0479908540499));
#31942=CARTESIAN_POINT('Ctrl Pts',(1.70767646263641,1.,-1.0479908540499));
#31943=CARTESIAN_POINT('Ctrl Pts',(1.71139783543986,-1.,-1.05277517202854));
#31944=CARTESIAN_POINT('Ctrl Pts',(1.71139783543986,1.,-1.05277517202854));
#31945=CARTESIAN_POINT('Ctrl Pts',(1.71508654427022,-1.,-1.05760163192481));
#31946=CARTESIAN_POINT('Ctrl Pts',(1.71508654427022,1.,-1.05760163192481));
#31947=CARTESIAN_POINT('Ctrl Pts',(1.71874858456908,-1.,-1.0624732468065));
#31948=CARTESIAN_POINT('Ctrl Pts',(1.71874858456908,1.,-1.0624732468065));
#31949=CARTESIAN_POINT('Ctrl Pts',(1.72238500928456,-1.,-1.06738966975463));
#31950=CARTESIAN_POINT('Ctrl Pts',(1.72238500928456,1.,-1.06738966975463));
#31951=CARTESIAN_POINT('Ctrl Pts',(1.72599406198489,-1.,-1.07234866990252));
#31952=CARTESIAN_POINT('Ctrl Pts',(1.72599406198489,1.,-1.07234866990252));
#31953=CARTESIAN_POINT('Ctrl Pts',(1.72957248977424,-1.,-1.0773470373727));
#31954=CARTESIAN_POINT('Ctrl Pts',(1.72957248977424,1.,-1.0773470373727));
#31955=CARTESIAN_POINT('Ctrl Pts',(1.73311705663407,-1.,-1.08238162784749));
#31956=CARTESIAN_POINT('Ctrl Pts',(1.73311705663407,1.,-1.08238162784749));
#31957=CARTESIAN_POINT('Ctrl Pts',(1.73662628326093,-1.,-1.08745056285429));
#31958=CARTESIAN_POINT('Ctrl Pts',(1.73662628326093,1.,-1.08745056285429));
#31959=CARTESIAN_POINT('Ctrl Pts',(1.74010053962252,-1.,-1.09255329056496));
#31960=CARTESIAN_POINT('Ctrl Pts',(1.74010053962252,1.,-1.09255329056496));
#31961=CARTESIAN_POINT('Ctrl Pts',(1.74354119236212,-1.,-1.09768999241229));
#31962=CARTESIAN_POINT('Ctrl Pts',(1.74354119236212,1.,-1.09768999241229));
#31963=CARTESIAN_POINT('Ctrl Pts',(1.74695004214924,-1.,-1.10286118991144));
#31964=CARTESIAN_POINT('Ctrl Pts',(1.74695004214924,1.,-1.10286118991144));
#31965=CARTESIAN_POINT('Ctrl Pts',(1.75032866075914,-1.,-1.10806728183003));
#31966=CARTESIAN_POINT('Ctrl Pts',(1.75032866075914,1.,-1.10806728183003));
#31967=CARTESIAN_POINT('Ctrl Pts',(1.75367772094617,-1.,-1.11330807582542));
#31968=CARTESIAN_POINT('Ctrl Pts',(1.75367772094617,1.,-1.11330807582542));
#31969=CARTESIAN_POINT('Ctrl Pts',(1.75699720772089,-1.,-1.11858293216752));
#31970=CARTESIAN_POINT('Ctrl Pts',(1.75699720772089,1.,-1.11858293216752));
#31971=CARTESIAN_POINT('Ctrl Pts',(1.76028671825084,-1.,-1.12389096855078));
#31972=CARTESIAN_POINT('Ctrl Pts',(1.76028671825084,1.,-1.12389096855078));
#31973=CARTESIAN_POINT('Ctrl Pts',(1.76354571966171,-1.,-1.12923123555076));
#31974=CARTESIAN_POINT('Ctrl Pts',(1.76354571966171,1.,-1.12923123555076));
#31975=CARTESIAN_POINT('Ctrl Pts',(1.76677384551883,-1.,-1.13460291804635));
#31976=CARTESIAN_POINT('Ctrl Pts',(1.76677384551883,1.,-1.13460291804635));
#31977=CARTESIAN_POINT('Ctrl Pts',(1.76997111386806,-1.,-1.14000548337));
#31978=CARTESIAN_POINT('Ctrl Pts',(1.76997111386806,1.,-1.14000548337));
#31979=CARTESIAN_POINT('Ctrl Pts',(1.77313777896234,-1.,-1.14543858226948));
#31980=CARTESIAN_POINT('Ctrl Pts',(1.77313777896234,1.,-1.14543858226948));
#31981=CARTESIAN_POINT('Ctrl Pts',(1.77627422557034,-1.,-1.15090197841531));
#31982=CARTESIAN_POINT('Ctrl Pts',(1.77627422557034,1.,-1.15090197841531));
#31983=CARTESIAN_POINT('Ctrl Pts',(1.77938085564261,-1.,-1.15639547194689));
#31984=CARTESIAN_POINT('Ctrl Pts',(1.77938085564261,1.,-1.15639547194689));
#31985=CARTESIAN_POINT('Ctrl Pts',(1.78245795880949,-1.,-1.16191881298458));
#31986=CARTESIAN_POINT('Ctrl Pts',(1.78245795880949,1.,-1.16191881298458));
#31987=CARTESIAN_POINT('Ctrl Pts',(1.78550566040349,-1.,-1.16747166312239));
#31988=CARTESIAN_POINT('Ctrl Pts',(1.78550566040349,1.,-1.16747166312239));
#31989=CARTESIAN_POINT('Ctrl Pts',(1.78852398877523,-1.,-1.17305363177265));
#31990=CARTESIAN_POINT('Ctrl Pts',(1.78852398877523,1.,-1.17305363177265));
#31991=CARTESIAN_POINT('Ctrl Pts',(1.79151291552646,-1.,-1.17866429440781));
#31992=CARTESIAN_POINT('Ctrl Pts',(1.79151291552646,1.,-1.17866429440781));
#31993=CARTESIAN_POINT('Ctrl Pts',(1.79447240321572,-1.,-1.18430321697471));
#31994=CARTESIAN_POINT('Ctrl Pts',(1.79447240321572,1.,-1.18430321697471));
#31995=CARTESIAN_POINT('Ctrl Pts',(1.79740245923649,-1.,-1.1899699793456));
#31996=CARTESIAN_POINT('Ctrl Pts',(1.79740245923649,1.,-1.1899699793456));
#31997=CARTESIAN_POINT('Ctrl Pts',(1.80030314370121,-1.,-1.19566418930405));
#31998=CARTESIAN_POINT('Ctrl Pts',(1.80030314370121,1.,-1.19566418930405));
#31999=CARTESIAN_POINT('Ctrl Pts',(1.8031745483882,-1.,-1.2013854893912));
#32000=CARTESIAN_POINT('Ctrl Pts',(1.8031745483882,1.,-1.2013854893912));
#32001=CARTESIAN_POINT('Ctrl Pts',(1.80601678480772,-1.,-1.20713356605519));
#32002=CARTESIAN_POINT('Ctrl Pts',(1.80601678480772,1.,-1.20713356605519));
#32003=CARTESIAN_POINT('Ctrl Pts',(1.80882996916931,-1.,-1.2129081570818));
#32004=CARTESIAN_POINT('Ctrl Pts',(1.80882996916931,1.,-1.2129081570818));
#32005=CARTESIAN_POINT('Ctrl Pts',(1.81161420806172,-1.,-1.2187090610323));
#32006=CARTESIAN_POINT('Ctrl Pts',(1.81161420806172,1.,-1.2187090610323));
#32007=CARTESIAN_POINT('Ctrl Pts',(1.81436959209778,-1.,-1.22453613304507));
#32008=CARTESIAN_POINT('Ctrl Pts',(1.81436959209778,1.,-1.22453613304507));
#32009=CARTESIAN_POINT('Ctrl Pts',(1.81655087183054,-1.,-1.22921864890975));
#32010=CARTESIAN_POINT('Ctrl Pts',(1.81655087183054,1.,-1.22921864890975));
#32011=CARTESIAN_POINT('Ctrl Pts',(1.81817389920914,-1.,-1.23274224526804));
#32012=CARTESIAN_POINT('Ctrl Pts',(1.81817389920914,1.,-1.23274224526804));
#32013=CARTESIAN_POINT('Ctrl Pts',(1.81925017193531,-1.,-1.23509651170384));
#32014=CARTESIAN_POINT('Ctrl Pts',(1.81925017193531,1.,-1.23509651170384));
#32015=CARTESIAN_POINT('Ctrl Pts',(1.81978687191668,-1.,-1.23627494547115));
#32016=CARTESIAN_POINT('Ctrl Pts',(1.81978687191668,1.,-1.23627494547115));
#32017=CARTESIAN_POINT('',(1.5055822144029,1.,-0.892032620296855));
#32018=CARTESIAN_POINT('Ctrl Pts',(1.5055822144029,1.,-0.892032620296855));
#32019=CARTESIAN_POINT('Ctrl Pts',(1.50980486807181,1.,-0.894452006967538));
#32020=CARTESIAN_POINT('Ctrl Pts',(1.51805569591479,1.,-0.89918504749193));
#32021=CARTESIAN_POINT('Ctrl Pts',(1.52984849890434,1.,-0.905967409640499));
#32022=CARTESIAN_POINT('Ctrl Pts',(1.54440491152807,1.,-0.91437591904658));
#32023=CARTESIAN_POINT('Ctrl Pts',(1.56065988582509,1.,-0.923832188966322));
#32024=CARTESIAN_POINT('Ctrl Pts',(1.57499388385561,1.,-0.932246680128849));
#32025=CARTESIAN_POINT('Ctrl Pts',(1.58744937489796,1.,-0.939646377909319));
#32026=CARTESIAN_POINT('Ctrl Pts',(1.59810042045408,1.,-0.946078063325796));
#32027=CARTESIAN_POINT('Ctrl Pts',(1.60706069897794,1.,-0.951613284361248));
#32028=CARTESIAN_POINT('Ctrl Pts',(1.61449324337233,1.,-0.956354422921573));
#32029=CARTESIAN_POINT('Ctrl Pts',(1.62061638139929,1.,-0.960438326099958));
#32030=CARTESIAN_POINT('Ctrl Pts',(1.6257193066974,1.,-0.964046107037821));
#32031=CARTESIAN_POINT('Ctrl Pts',(1.63013849959083,1.,-0.967387853228041));
#32032=CARTESIAN_POINT('Ctrl Pts',(1.63420665729609,1.,-0.970669715996356));
#32033=CARTESIAN_POINT('Ctrl Pts',(1.63820952658157,1.,-0.974066058287501));
#32034=CARTESIAN_POINT('Ctrl Pts',(1.64233990826831,1.,-0.977689794120297));
#32035=CARTESIAN_POINT('Ctrl Pts',(1.64665139190834,1.,-0.981562530940574));
#32036=CARTESIAN_POINT('Ctrl Pts',(1.6511001661277,1.,-0.985642622921626));
#32037=CARTESIAN_POINT('Ctrl Pts',(1.65559044289746,1.,-0.98985562785445));
#32038=CARTESIAN_POINT('Ctrl Pts',(1.66001553809916,1.,-0.994121836661116));
#32039=CARTESIAN_POINT('Ctrl Pts',(1.66430758030304,1.,-0.998389654952317));
#32040=CARTESIAN_POINT('Ctrl Pts',(1.66846059277231,1.,-1.00265091003682));
#32041=CARTESIAN_POINT('Ctrl Pts',(1.67250335383248,1.,-1.00692206696387));
#32042=CARTESIAN_POINT('Ctrl Pts',(1.67648246776457,1.,-1.01123236493507));
#32043=CARTESIAN_POINT('Ctrl Pts',(1.6804428989482,1.,-1.01561026162787));
#32044=CARTESIAN_POINT('Ctrl Pts',(1.68440578021739,1.,-1.02006795074222));
#32045=CARTESIAN_POINT('Ctrl Pts',(1.68836910178475,1.,-1.02460180535272));
#32046=CARTESIAN_POINT('Ctrl Pts',(1.69231840863471,1.,-1.02919977579155));
#32047=CARTESIAN_POINT('Ctrl Pts',(1.69623414782769,1.,-1.03384646003587));
#32048=CARTESIAN_POINT('Ctrl Pts',(1.70010052930951,1.,-1.03852922490782));
#32049=CARTESIAN_POINT('Ctrl Pts',(1.70391338707969,1.,-1.04324363334546));
#32050=CARTESIAN_POINT('Ctrl Pts',(1.70767646263641,1.,-1.0479908540499));
#32051=CARTESIAN_POINT('Ctrl Pts',(1.71139783543986,1.,-1.05277517202854));
#32052=CARTESIAN_POINT('Ctrl Pts',(1.71508654427022,1.,-1.05760163192481));
#32053=CARTESIAN_POINT('Ctrl Pts',(1.71874858456908,1.,-1.0624732468065));
#32054=CARTESIAN_POINT('Ctrl Pts',(1.72238500928456,1.,-1.06738966975463));
#32055=CARTESIAN_POINT('Ctrl Pts',(1.72599406198489,1.,-1.07234866990252));
#32056=CARTESIAN_POINT('Ctrl Pts',(1.72957248977424,1.,-1.0773470373727));
#32057=CARTESIAN_POINT('Ctrl Pts',(1.73311705663407,1.,-1.08238162784749));
#32058=CARTESIAN_POINT('Ctrl Pts',(1.73662628326093,1.,-1.08745056285429));
#32059=CARTESIAN_POINT('Ctrl Pts',(1.74010053962252,1.,-1.09255329056496));
#32060=CARTESIAN_POINT('Ctrl Pts',(1.74354119236212,1.,-1.09768999241229));
#32061=CARTESIAN_POINT('Ctrl Pts',(1.74695004214924,1.,-1.10286118991144));
#32062=CARTESIAN_POINT('Ctrl Pts',(1.75032866075914,1.,-1.10806728183003));
#32063=CARTESIAN_POINT('Ctrl Pts',(1.75367772094617,1.,-1.11330807582542));
#32064=CARTESIAN_POINT('Ctrl Pts',(1.75699720772089,1.,-1.11858293216752));
#32065=CARTESIAN_POINT('Ctrl Pts',(1.76028671825084,1.,-1.12389096855078));
#32066=CARTESIAN_POINT('Ctrl Pts',(1.76354571966171,1.,-1.12923123555076));
#32067=CARTESIAN_POINT('Ctrl Pts',(1.76677384551883,1.,-1.13460291804635));
#32068=CARTESIAN_POINT('Ctrl Pts',(1.76997111386806,1.,-1.14000548337));
#32069=CARTESIAN_POINT('Ctrl Pts',(1.77313777896234,1.,-1.14543858226948));
#32070=CARTESIAN_POINT('Ctrl Pts',(1.77627422557034,1.,-1.15090197841531));
#32071=CARTESIAN_POINT('Ctrl Pts',(1.77938085564261,1.,-1.15639547194689));
#32072=CARTESIAN_POINT('Ctrl Pts',(1.78245795880949,1.,-1.16191881298458));
#32073=CARTESIAN_POINT('Ctrl Pts',(1.78550566040349,1.,-1.16747166312239));
#32074=CARTESIAN_POINT('Ctrl Pts',(1.78852398877523,1.,-1.17305363177265));
#32075=CARTESIAN_POINT('Ctrl Pts',(1.79151291552646,1.,-1.17866429440781));
#32076=CARTESIAN_POINT('Ctrl Pts',(1.79447240321572,1.,-1.18430321697471));
#32077=CARTESIAN_POINT('Ctrl Pts',(1.79740245923649,1.,-1.1899699793456));
#32078=CARTESIAN_POINT('Ctrl Pts',(1.80030314370121,1.,-1.19566418930405));
#32079=CARTESIAN_POINT('Ctrl Pts',(1.8031745483882,1.,-1.2013854893912));
#32080=CARTESIAN_POINT('Ctrl Pts',(1.80601678480772,1.,-1.20713356605519));
#32081=CARTESIAN_POINT('Ctrl Pts',(1.80882996916931,1.,-1.2129081570818));
#32082=CARTESIAN_POINT('Ctrl Pts',(1.81161420806172,1.,-1.2187090610323));
#32083=CARTESIAN_POINT('Ctrl Pts',(1.81436959209778,1.,-1.22453613304507));
#32084=CARTESIAN_POINT('Ctrl Pts',(1.81655087183054,1.,-1.22921864890975));
#32085=CARTESIAN_POINT('Ctrl Pts',(1.81817389920914,1.,-1.23274224526804));
#32086=CARTESIAN_POINT('Ctrl Pts',(1.81925017193531,1.,-1.23509651170384));
#32087=CARTESIAN_POINT('Ctrl Pts',(1.81978687191668,1.,-1.23627494547115));
#32088=CARTESIAN_POINT('',(1.5055822144029,0.,-0.892032620296855));
#32089=CARTESIAN_POINT('Origin',(0.,0.,0.));
#32090=CARTESIAN_POINT('',(1.60662857109684,1.,-0.693717979106306));
#32091=CARTESIAN_POINT('Origin',(0.,1.,0.));
#32092=CARTESIAN_POINT('',(1.60662857109684,0.,-0.693717979106308));
#32093=CARTESIAN_POINT('Ctrl Pts',(2.0698113262342,-1.,-0.745574324794401));
#32094=CARTESIAN_POINT('Ctrl Pts',(2.0698113262342,1.,-0.745574324794401));
#32095=CARTESIAN_POINT('Ctrl Pts',(2.06854248895728,-1.,-0.745832791378367));
#32096=CARTESIAN_POINT('Ctrl Pts',(2.06854248895728,1.,-0.745832791378367));
#32097=CARTESIAN_POINT('Ctrl Pts',(2.06600523016815,-1.,-0.746345871544201));
#32098=CARTESIAN_POINT('Ctrl Pts',(2.06600523016815,1.,-0.746345871544201));
#32099=CARTESIAN_POINT('Ctrl Pts',(2.06220058927826,-1.,-0.74710393278792));
#32100=CARTESIAN_POINT('Ctrl Pts',(2.06220058927826,1.,-0.74710393278792));
#32101=CARTESIAN_POINT('Ctrl Pts',(2.05713023031006,-1.,-0.748091554183803));
#32102=CARTESIAN_POINT('Ctrl Pts',(2.05713023031006,1.,-0.748091554183803));
#32103=CARTESIAN_POINT('Ctrl Pts',(2.05079645592154,-1.,-0.749287468665046));
#32104=CARTESIAN_POINT('Ctrl Pts',(2.05079645592154,1.,-0.749287468665046));
#32105=CARTESIAN_POINT('Ctrl Pts',(2.04446689147979,-1.,-0.750444657875576));
#32106=CARTESIAN_POINT('Ctrl Pts',(2.04446689147979,1.,-0.750444657875576));
#32107=CARTESIAN_POINT('Ctrl Pts',(2.03814160092099,-1.,-0.751562963361115));
#32108=CARTESIAN_POINT('Ctrl Pts',(2.03814160092099,1.,-0.751562963361115));
#32109=CARTESIAN_POINT('Ctrl Pts',(2.03182068456221,-1.,-0.752642180487211));
#32110=CARTESIAN_POINT('Ctrl Pts',(2.03182068456221,1.,-0.752642180487211));
#32111=CARTESIAN_POINT('Ctrl Pts',(2.02550428623313,-1.,-0.753682061112768));
#32112=CARTESIAN_POINT('Ctrl Pts',(2.02550428623313,1.,-0.753682061112768));
#32113=CARTESIAN_POINT('Ctrl Pts',(2.01919259405809,-1.,-0.754682330722816));
#32114=CARTESIAN_POINT('Ctrl Pts',(2.01919259405809,1.,-0.754682330722816));
#32115=CARTESIAN_POINT('Ctrl Pts',(2.01288584328084,-1.,-0.755642704957865));
#32116=CARTESIAN_POINT('Ctrl Pts',(2.01288584328084,1.,-0.755642704957865));
#32117=CARTESIAN_POINT('Ctrl Pts',(2.0065843158773,-1.,-0.756562904646671));
#32118=CARTESIAN_POINT('Ctrl Pts',(2.0065843158773,1.,-0.756562904646671));
#32119=CARTESIAN_POINT('Ctrl Pts',(2.00028834739178,-1.,-0.757442676862724));
#32120=CARTESIAN_POINT('Ctrl Pts',(2.00028834739178,1.,-0.757442676862724));
#32121=CARTESIAN_POINT('Ctrl Pts',(1.99399831098817,-1.,-0.758281796766761));
#32122=CARTESIAN_POINT('Ctrl Pts',(1.99399831098817,1.,-0.758281796766761));
#32123=CARTESIAN_POINT('Ctrl Pts',(1.98771456680874,-1.,-0.759080037802488));
#32124=CARTESIAN_POINT('Ctrl Pts',(1.98771456680874,1.,-0.759080037802488));
#32125=CARTESIAN_POINT('Ctrl Pts',(1.98143741418172,-1.,-0.75983714745219));
#32126=CARTESIAN_POINT('Ctrl Pts',(1.98143741418172,1.,-0.75983714745219));
#32127=CARTESIAN_POINT('Ctrl Pts',(1.97516705321494,-1.,-0.760552825409757));
#32128=CARTESIAN_POINT('Ctrl Pts',(1.97516705321494,1.,-0.760552825409757));
#32129=CARTESIAN_POINT('Ctrl Pts',(1.96890351582499,-1.,-0.761226690483821));
#32130=CARTESIAN_POINT('Ctrl Pts',(1.96890351582499,1.,-0.761226690483821));
#32131=CARTESIAN_POINT('Ctrl Pts',(1.96264672744186,-1.,-0.761858300014424));
#32132=CARTESIAN_POINT('Ctrl Pts',(1.96264672744186,1.,-0.761858300014424));
#32133=CARTESIAN_POINT('Ctrl Pts',(1.95639665309869,-1.,-0.762447203806179));
#32134=CARTESIAN_POINT('Ctrl Pts',(1.95639665309869,1.,-0.762447203806179));
#32135=CARTESIAN_POINT('Ctrl Pts',(1.95015342590024,-1.,-0.762992990878769));
#32136=CARTESIAN_POINT('Ctrl Pts',(1.95015342590024,1.,-0.762992990878769));
#32137=CARTESIAN_POINT('Ctrl Pts',(1.9439174661764,-1.,-0.763495333538629));
#32138=CARTESIAN_POINT('Ctrl Pts',(1.9439174661764,1.,-0.763495333538629));
#32139=CARTESIAN_POINT('Ctrl Pts',(1.93768964875886,-1.,-0.763954049121459));
#32140=CARTESIAN_POINT('Ctrl Pts',(1.93768964875886,1.,-0.763954049121459));
#32141=CARTESIAN_POINT('Ctrl Pts',(1.93147105496382,-1.,-0.764369010673941));
#32142=CARTESIAN_POINT('Ctrl Pts',(1.93147105496382,1.,-0.764369010673941));
#32143=CARTESIAN_POINT('Ctrl Pts',(1.92526263537048,-1.,-0.764740025488212));
#32144=CARTESIAN_POINT('Ctrl Pts',(1.92526263537048,1.,-0.764740025488212));
#32145=CARTESIAN_POINT('Ctrl Pts',(1.91906491634196,-1.,-0.765066729667089));
#32146=CARTESIAN_POINT('Ctrl Pts',(1.91906491634196,1.,-0.765066729667089));
#32147=CARTESIAN_POINT('Ctrl Pts',(1.91287765805169,-1.,-0.765348465884722));
#32148=CARTESIAN_POINT('Ctrl Pts',(1.91287765805169,1.,-0.765348465884722));
#32149=CARTESIAN_POINT('Ctrl Pts',(1.90669961402356,-1.,-0.765584196937919));
#32150=CARTESIAN_POINT('Ctrl Pts',(1.90669961402356,1.,-0.765584196937919));
#32151=CARTESIAN_POINT('Ctrl Pts',(1.90052930393596,-1.,-0.765772772593386));
#32152=CARTESIAN_POINT('Ctrl Pts',(1.90052930393596,1.,-0.765772772593386));
#32153=CARTESIAN_POINT('Ctrl Pts',(1.89436577771388,-1.,-0.765913193856978));
#32154=CARTESIAN_POINT('Ctrl Pts',(1.89436577771388,1.,-0.765913193856978));
#32155=CARTESIAN_POINT('Ctrl Pts',(1.88820926433409,-1.,-0.766004837062091));
#32156=CARTESIAN_POINT('Ctrl Pts',(1.88820926433409,1.,-0.766004837062091));
#32157=CARTESIAN_POINT('Ctrl Pts',(1.88206215302561,-1.,-0.766047794851865));
#32158=CARTESIAN_POINT('Ctrl Pts',(1.88206215302561,1.,-0.766047794851865));
#32159=CARTESIAN_POINT('Ctrl Pts',(1.87592888967883,-1.,-0.766042837036744));
#32160=CARTESIAN_POINT('Ctrl Pts',(1.87592888967883,1.,-0.766042837036744));
#32161=CARTESIAN_POINT('Ctrl Pts',(1.86981398314341,-1.,-0.765990708546091));
#32162=CARTESIAN_POINT('Ctrl Pts',(1.86981398314341,1.,-0.765990708546091));
#32163=CARTESIAN_POINT('Ctrl Pts',(1.86372027063312,-1.,-0.765891519092547));
#32164=CARTESIAN_POINT('Ctrl Pts',(1.86372027063312,1.,-0.765891519092547));
#32165=CARTESIAN_POINT('Ctrl Pts',(1.85764741390394,-1.,-0.765744212909319));
#32166=CARTESIAN_POINT('Ctrl Pts',(1.85764741390394,1.,-0.765744212909319));
#32167=CARTESIAN_POINT('Ctrl Pts',(1.85158945130063,-1.,-0.765545710619063));
#32168=CARTESIAN_POINT('Ctrl Pts',(1.85158945130063,1.,-0.765545710619063));
#32169=CARTESIAN_POINT('Ctrl Pts',(1.84553698875924,-1.,-0.765291664862029));
#32170=CARTESIAN_POINT('Ctrl Pts',(1.84553698875924,1.,-0.765291664862029));
#32171=CARTESIAN_POINT('Ctrl Pts',(1.83948181064835,-1.,-0.764978057881738));
#32172=CARTESIAN_POINT('Ctrl Pts',(1.83948181064835,1.,-0.764978057881738));
#32173=CARTESIAN_POINT('Ctrl Pts',(1.83342077227142,-1.,-0.764602549687853));
#32174=CARTESIAN_POINT('Ctrl Pts',(1.83342077227142,1.,-0.764602549687853));
#32175=CARTESIAN_POINT('Ctrl Pts',(1.82735991200065,-1.,-0.764165902605995));
#32176=CARTESIAN_POINT('Ctrl Pts',(1.82735991200065,1.,-0.764165902605995));
#32177=CARTESIAN_POINT('Ctrl Pts',(1.82131873145266,-1.,-0.763673465462727));
#32178=CARTESIAN_POINT('Ctrl Pts',(1.82131873145266,1.,-0.763673465462727));
#32179=CARTESIAN_POINT('Ctrl Pts',(1.8153211840553,-1.,-0.763132003836634));
#32180=CARTESIAN_POINT('Ctrl Pts',(1.8153211840553,1.,-0.763132003836634));
#32181=CARTESIAN_POINT('Ctrl Pts',(1.80938551463965,-1.,-0.762546129463938));
#32182=CARTESIAN_POINT('Ctrl Pts',(1.80938551463965,1.,-0.762546129463938));
#32183=CARTESIAN_POINT('Ctrl Pts',(1.80351583877342,-1.,-0.761915336443547));
#32184=CARTESIAN_POINT('Ctrl Pts',(1.80351583877342,1.,-0.761915336443547));
#32185=CARTESIAN_POINT('Ctrl Pts',(1.79768986997783,-1.,-0.761229695230558));
#32186=CARTESIAN_POINT('Ctrl Pts',(1.79768986997783,1.,-0.761229695230558));
#32187=CARTESIAN_POINT('Ctrl Pts',(1.7918581561088,-1.,-0.760469555880749));
#32188=CARTESIAN_POINT('Ctrl Pts',(1.7918581561088,1.,-0.760469555880749));
#32189=CARTESIAN_POINT('Ctrl Pts',(1.78596964884604,-1.,-0.75961440111019));
#32190=CARTESIAN_POINT('Ctrl Pts',(1.78596964884604,1.,-0.75961440111019));
#32191=CARTESIAN_POINT('Ctrl Pts',(1.77999411220945,-1.,-0.758650626677519));
#32192=CARTESIAN_POINT('Ctrl Pts',(1.77999411220945,1.,-0.758650626677519));
#32193=CARTESIAN_POINT('Ctrl Pts',(1.77394167108292,-1.,-0.757578264077029));
#32194=CARTESIAN_POINT('Ctrl Pts',(1.77394167108292,1.,-0.757578264077029));
#32195=CARTESIAN_POINT('Ctrl Pts',(1.76789396002998,-1.,-0.75642189602781));
#32196=CARTESIAN_POINT('Ctrl Pts',(1.76789396002998,1.,-0.75642189602781));
#32197=CARTESIAN_POINT('Ctrl Pts',(1.76197817240128,-1.,-0.755220979974462));
#32198=CARTESIAN_POINT('Ctrl Pts',(1.76197817240128,1.,-0.755220979974462));
#32199=CARTESIAN_POINT('Ctrl Pts',(1.75631083600019,-1.,-0.754009254027829));
#32200=CARTESIAN_POINT('Ctrl Pts',(1.75631083600019,1.,-0.754009254027829));
#32201=CARTESIAN_POINT('Ctrl Pts',(1.75095139468794,-1.,-0.752797683531314));
#32202=CARTESIAN_POINT('Ctrl Pts',(1.75095139468794,1.,-0.752797683531314));
#32203=CARTESIAN_POINT('Ctrl Pts',(1.74585086852502,-1.,-0.751555614164483));
#32204=CARTESIAN_POINT('Ctrl Pts',(1.74585086852502,1.,-0.751555614164483));
#32205=CARTESIAN_POINT('Ctrl Pts',(1.74080458267114,-1.,-0.75019343598125));
#32206=CARTESIAN_POINT('Ctrl Pts',(1.74080458267114,1.,-0.75019343598125));
#32207=CARTESIAN_POINT('Ctrl Pts',(1.7355035168033,-1.,-0.74858246295687));
#32208=CARTESIAN_POINT('Ctrl Pts',(1.7355035168033,1.,-0.74858246295687));
#32209=CARTESIAN_POINT('Ctrl Pts',(1.72958533647714,-1.,-0.746574710097752));
#32210=CARTESIAN_POINT('Ctrl Pts',(1.72958533647714,1.,-0.746574710097752));
#32211=CARTESIAN_POINT('Ctrl Pts',(1.72268229916769,-1.,-0.744021445433094));
#32212=CARTESIAN_POINT('Ctrl Pts',(1.72268229916769,1.,-0.744021445433094));
#32213=CARTESIAN_POINT('Ctrl Pts',(1.71447789751001,-1.,-0.74079516202821));
#32214=CARTESIAN_POINT('Ctrl Pts',(1.71447789751001,1.,-0.74079516202821));
#32215=CARTESIAN_POINT('Ctrl Pts',(1.70473309004249,-1.,-0.736799665716932));
#32216=CARTESIAN_POINT('Ctrl Pts',(1.70473309004249,1.,-0.736799665716932));
#32217=CARTESIAN_POINT('Ctrl Pts',(1.69326921972915,-1.,-0.731963238685357));
#32218=CARTESIAN_POINT('Ctrl Pts',(1.69326921972915,1.,-0.731963238685357));
#32219=CARTESIAN_POINT('Ctrl Pts',(1.67996158451922,-1.,-0.726235967982445));
#32220=CARTESIAN_POINT('Ctrl Pts',(1.67996158451922,1.,-0.726235967982445));
#32221=CARTESIAN_POINT('Ctrl Pts',(1.66472880551777,-1.,-0.71958543378795));
#32222=CARTESIAN_POINT('Ctrl Pts',(1.66472880551777,1.,-0.71958543378795));
#32223=CARTESIAN_POINT('Ctrl Pts',(1.64752408828442,-1.,-0.711993139340448));
#32224=CARTESIAN_POINT('Ctrl Pts',(1.64752408828442,1.,-0.711993139340448));
#32225=CARTESIAN_POINT('Ctrl Pts',(1.6321654166204,-1.,-0.705159151977294));
#32226=CARTESIAN_POINT('Ctrl Pts',(1.6321654166204,1.,-0.705159151977294));
#32227=CARTESIAN_POINT('Ctrl Pts',(1.61974673471117,-1.,-0.699605146398837));
#32228=CARTESIAN_POINT('Ctrl Pts',(1.61974673471117,1.,-0.699605146398837));
#32229=CARTESIAN_POINT('Ctrl Pts',(1.61106790957619,-1.,-0.69571209787897));
#32230=CARTESIAN_POINT('Ctrl Pts',(1.61106790957619,1.,-0.69571209787897));
#32231=CARTESIAN_POINT('Ctrl Pts',(1.60662857109684,-1.,-0.693717979106306));
#32232=CARTESIAN_POINT('Ctrl Pts',(1.60662857109684,1.,-0.693717979106306));
#32233=CARTESIAN_POINT('',(2.0698113262342,1.,-0.745574324794401));
#32234=CARTESIAN_POINT('Ctrl Pts',(2.0698113262342,1.,-0.745574324794401));
#32235=CARTESIAN_POINT('Ctrl Pts',(2.06854248895728,1.,-0.745832791378367));
#32236=CARTESIAN_POINT('Ctrl Pts',(2.06600523016815,1.,-0.746345871544201));
#32237=CARTESIAN_POINT('Ctrl Pts',(2.06220058927826,1.,-0.74710393278792));
#32238=CARTESIAN_POINT('Ctrl Pts',(2.05713023031006,1.,-0.748091554183803));
#32239=CARTESIAN_POINT('Ctrl Pts',(2.05079645592154,1.,-0.749287468665046));
#32240=CARTESIAN_POINT('Ctrl Pts',(2.04446689147979,1.,-0.750444657875576));
#32241=CARTESIAN_POINT('Ctrl Pts',(2.03814160092099,1.,-0.751562963361115));
#32242=CARTESIAN_POINT('Ctrl Pts',(2.03182068456221,1.,-0.752642180487211));
#32243=CARTESIAN_POINT('Ctrl Pts',(2.02550428623313,1.,-0.753682061112768));
#32244=CARTESIAN_POINT('Ctrl Pts',(2.01919259405809,1.,-0.754682330722816));
#32245=CARTESIAN_POINT('Ctrl Pts',(2.01288584328084,1.,-0.755642704957865));
#32246=CARTESIAN_POINT('Ctrl Pts',(2.0065843158773,1.,-0.756562904646671));
#32247=CARTESIAN_POINT('Ctrl Pts',(2.00028834739178,1.,-0.757442676862724));
#32248=CARTESIAN_POINT('Ctrl Pts',(1.99399831098817,1.,-0.758281796766761));
#32249=CARTESIAN_POINT('Ctrl Pts',(1.98771456680874,1.,-0.759080037802488));
#32250=CARTESIAN_POINT('Ctrl Pts',(1.98143741418172,1.,-0.75983714745219));
#32251=CARTESIAN_POINT('Ctrl Pts',(1.97516705321494,1.,-0.760552825409757));
#32252=CARTESIAN_POINT('Ctrl Pts',(1.96890351582499,1.,-0.761226690483821));
#32253=CARTESIAN_POINT('Ctrl Pts',(1.96264672744186,1.,-0.761858300014424));
#32254=CARTESIAN_POINT('Ctrl Pts',(1.95639665309869,1.,-0.762447203806179));
#32255=CARTESIAN_POINT('Ctrl Pts',(1.95015342590024,1.,-0.762992990878769));
#32256=CARTESIAN_POINT('Ctrl Pts',(1.9439174661764,1.,-0.763495333538629));
#32257=CARTESIAN_POINT('Ctrl Pts',(1.93768964875886,1.,-0.763954049121459));
#32258=CARTESIAN_POINT('Ctrl Pts',(1.93147105496382,1.,-0.764369010673941));
#32259=CARTESIAN_POINT('Ctrl Pts',(1.92526263537048,1.,-0.764740025488212));
#32260=CARTESIAN_POINT('Ctrl Pts',(1.91906491634196,1.,-0.765066729667089));
#32261=CARTESIAN_POINT('Ctrl Pts',(1.91287765805169,1.,-0.765348465884722));
#32262=CARTESIAN_POINT('Ctrl Pts',(1.90669961402356,1.,-0.765584196937919));
#32263=CARTESIAN_POINT('Ctrl Pts',(1.90052930393596,1.,-0.765772772593386));
#32264=CARTESIAN_POINT('Ctrl Pts',(1.89436577771388,1.,-0.765913193856978));
#32265=CARTESIAN_POINT('Ctrl Pts',(1.88820926433409,1.,-0.766004837062091));
#32266=CARTESIAN_POINT('Ctrl Pts',(1.88206215302561,1.,-0.766047794851865));
#32267=CARTESIAN_POINT('Ctrl Pts',(1.87592888967883,1.,-0.766042837036744));
#32268=CARTESIAN_POINT('Ctrl Pts',(1.86981398314341,1.,-0.765990708546091));
#32269=CARTESIAN_POINT('Ctrl Pts',(1.86372027063312,1.,-0.765891519092547));
#32270=CARTESIAN_POINT('Ctrl Pts',(1.85764741390394,1.,-0.765744212909319));
#32271=CARTESIAN_POINT('Ctrl Pts',(1.85158945130063,1.,-0.765545710619063));
#32272=CARTESIAN_POINT('Ctrl Pts',(1.84553698875924,1.,-0.765291664862029));
#32273=CARTESIAN_POINT('Ctrl Pts',(1.83948181064835,1.,-0.764978057881738));
#32274=CARTESIAN_POINT('Ctrl Pts',(1.83342077227142,1.,-0.764602549687853));
#32275=CARTESIAN_POINT('Ctrl Pts',(1.82735991200065,1.,-0.764165902605995));
#32276=CARTESIAN_POINT('Ctrl Pts',(1.82131873145266,1.,-0.763673465462727));
#32277=CARTESIAN_POINT('Ctrl Pts',(1.8153211840553,1.,-0.763132003836634));
#32278=CARTESIAN_POINT('Ctrl Pts',(1.80938551463965,1.,-0.762546129463938));
#32279=CARTESIAN_POINT('Ctrl Pts',(1.80351583877342,1.,-0.761915336443547));
#32280=CARTESIAN_POINT('Ctrl Pts',(1.79768986997783,1.,-0.761229695230558));
#32281=CARTESIAN_POINT('Ctrl Pts',(1.7918581561088,1.,-0.760469555880749));
#32282=CARTESIAN_POINT('Ctrl Pts',(1.78596964884604,1.,-0.75961440111019));
#32283=CARTESIAN_POINT('Ctrl Pts',(1.77999411220945,1.,-0.758650626677519));
#32284=CARTESIAN_POINT('Ctrl Pts',(1.77394167108292,1.,-0.757578264077029));
#32285=CARTESIAN_POINT('Ctrl Pts',(1.76789396002998,1.,-0.75642189602781));
#32286=CARTESIAN_POINT('Ctrl Pts',(1.76197817240128,1.,-0.755220979974462));
#32287=CARTESIAN_POINT('Ctrl Pts',(1.75631083600019,1.,-0.754009254027829));
#32288=CARTESIAN_POINT('Ctrl Pts',(1.75095139468794,1.,-0.752797683531314));
#32289=CARTESIAN_POINT('Ctrl Pts',(1.74585086852502,1.,-0.751555614164483));
#32290=CARTESIAN_POINT('Ctrl Pts',(1.74080458267114,1.,-0.75019343598125));
#32291=CARTESIAN_POINT('Ctrl Pts',(1.7355035168033,1.,-0.74858246295687));
#32292=CARTESIAN_POINT('Ctrl Pts',(1.72958533647714,1.,-0.746574710097752));
#32293=CARTESIAN_POINT('Ctrl Pts',(1.72268229916769,1.,-0.744021445433094));
#32294=CARTESIAN_POINT('Ctrl Pts',(1.71447789751001,1.,-0.74079516202821));
#32295=CARTESIAN_POINT('Ctrl Pts',(1.70473309004249,1.,-0.736799665716932));
#32296=CARTESIAN_POINT('Ctrl Pts',(1.69326921972915,1.,-0.731963238685357));
#32297=CARTESIAN_POINT('Ctrl Pts',(1.67996158451922,1.,-0.726235967982445));
#32298=CARTESIAN_POINT('Ctrl Pts',(1.66472880551777,1.,-0.71958543378795));
#32299=CARTESIAN_POINT('Ctrl Pts',(1.64752408828442,1.,-0.711993139340448));
#32300=CARTESIAN_POINT('Ctrl Pts',(1.6321654166204,1.,-0.705159151977294));
#32301=CARTESIAN_POINT('Ctrl Pts',(1.61974673471117,1.,-0.699605146398837));
#32302=CARTESIAN_POINT('Ctrl Pts',(1.61106790957619,1.,-0.69571209787897));
#32303=CARTESIAN_POINT('Ctrl Pts',(1.60662857109684,1.,-0.693717979106306));
#32304=CARTESIAN_POINT('',(2.0698113262342,0.,-0.745574324794401));
#32305=CARTESIAN_POINT('Origin',(2.11275013067528,0.,-0.61342227326009));
#32306=CARTESIAN_POINT('',(2.11275013067528,1.,-0.61342227326009));
#32307=CARTESIAN_POINT('',(2.0698113262342,1.,-0.745574324794401));
#32308=CARTESIAN_POINT('',(2.11275013067528,0.,-0.61342227326009));
#32309=CARTESIAN_POINT('Ctrl Pts',(1.7075470150345,-1.,-0.383122945602004));
#32310=CARTESIAN_POINT('Ctrl Pts',(1.7075470150345,1.,-0.383122945602004));
#32311=CARTESIAN_POINT('Ctrl Pts',(1.71231062891958,-1.,-0.384119047315542));
#32312=CARTESIAN_POINT('Ctrl Pts',(1.71231062891958,1.,-0.384119047315542));
#32313=CARTESIAN_POINT('Ctrl Pts',(1.72162022246158,-1.,-0.38607079032701));
#32314=CARTESIAN_POINT('Ctrl Pts',(1.72162022246158,1.,-0.38607079032701));
#32315=CARTESIAN_POINT('Ctrl Pts',(1.7349317097561,-1.,-0.388877023509192));
#32316=CARTESIAN_POINT('Ctrl Pts',(1.7349317097561,1.,-0.388877023509192));
#32317=CARTESIAN_POINT('Ctrl Pts',(1.75137405313962,-1.,-0.392375812294307));
#32318=CARTESIAN_POINT('Ctrl Pts',(1.75137405313962,1.,-0.392375812294307));
#32319=CARTESIAN_POINT('Ctrl Pts',(1.7697556004756,-1.,-0.39634619612042));
#32320=CARTESIAN_POINT('Ctrl Pts',(1.7697556004756,1.,-0.39634619612042));
#32321=CARTESIAN_POINT('Ctrl Pts',(1.78598826347533,-1.,-0.399919403783081));
#32322=CARTESIAN_POINT('Ctrl Pts',(1.78598826347533,1.,-0.399919403783081));
#32323=CARTESIAN_POINT('Ctrl Pts',(1.80012077176221,-1.,-0.403107976170441));
#32324=CARTESIAN_POINT('Ctrl Pts',(1.80012077176221,1.,-0.403107976170441));
#32325=CARTESIAN_POINT('Ctrl Pts',(1.81223801813988,-1.,-0.405933518411838));
#32326=CARTESIAN_POINT('Ctrl Pts',(1.81223801813988,1.,-0.405933518411838));
#32327=CARTESIAN_POINT('Ctrl Pts',(1.8224702267854,-1.,-0.408428948108534));
#32328=CARTESIAN_POINT('Ctrl Pts',(1.8224702267854,1.,-0.408428948108534));
#32329=CARTESIAN_POINT('Ctrl Pts',(1.83100408895216,-1.,-0.410641256301675));
#32330=CARTESIAN_POINT('Ctrl Pts',(1.83100408895216,1.,-0.410641256301675));
#32331=CARTESIAN_POINT('Ctrl Pts',(1.83808953475839,-1.,-0.412633125322162));
#32332=CARTESIAN_POINT('Ctrl Pts',(1.83808953475839,1.,-0.412633125322162));
#32333=CARTESIAN_POINT('Ctrl Pts',(1.8440575707371,-1.,-0.41448743825434));
#32334=CARTESIAN_POINT('Ctrl Pts',(1.8440575707371,1.,-0.41448743825434));
#32335=CARTESIAN_POINT('Ctrl Pts',(1.84929312929882,-1.,-0.416300022038864));
#32336=CARTESIAN_POINT('Ctrl Pts',(1.84929312929882,1.,-0.416300022038864));
#32337=CARTESIAN_POINT('Ctrl Pts',(1.85417632856234,-1.,-0.418164129143534));
#32338=CARTESIAN_POINT('Ctrl Pts',(1.85417632856234,1.,-0.418164129143534));
#32339=CARTESIAN_POINT('Ctrl Pts',(1.85903281096686,-1.,-0.42015728797562));
#32340=CARTESIAN_POINT('Ctrl Pts',(1.85903281096686,1.,-0.42015728797562));
#32341=CARTESIAN_POINT('Ctrl Pts',(1.86408083334028,-1.,-0.422327307418275));
#32342=CARTESIAN_POINT('Ctrl Pts',(1.86408083334028,1.,-0.422327307418275));
#32343=CARTESIAN_POINT('Ctrl Pts',(1.86937803944323,-1.,-0.424678177291359));
#32344=CARTESIAN_POINT('Ctrl Pts',(1.86937803944323,1.,-0.424678177291359));
#32345=CARTESIAN_POINT('Ctrl Pts',(1.87486989291484,-1.,-0.427183828519102));
#32346=CARTESIAN_POINT('Ctrl Pts',(1.87486989291484,1.,-0.427183828519102));
#32347=CARTESIAN_POINT('Ctrl Pts',(1.88044229001832,-1.,-0.429803062482345));
#32348=CARTESIAN_POINT('Ctrl Pts',(1.88044229001832,1.,-0.429803062482345));
#32349=CARTESIAN_POINT('Ctrl Pts',(1.88596913666793,-1.,-0.432493038548748));
#32350=CARTESIAN_POINT('Ctrl Pts',(1.88596913666793,1.,-0.432493038548748));
#32351=CARTESIAN_POINT('Ctrl Pts',(1.89136993975504,-1.,-0.435225660963383));
#32352=CARTESIAN_POINT('Ctrl Pts',(1.89136993975504,1.,-0.435225660963383));
#32353=CARTESIAN_POINT('Ctrl Pts',(1.89663648956466,-1.,-0.437995003948244));
#32354=CARTESIAN_POINT('Ctrl Pts',(1.89663648956466,1.,-0.437995003948244));
#32355=CARTESIAN_POINT('Ctrl Pts',(1.90180124389086,-1.,-0.440807833704038));
#32356=CARTESIAN_POINT('Ctrl Pts',(1.90180124389086,1.,-0.440807833704038));
#32357=CARTESIAN_POINT('Ctrl Pts',(1.90691756144898,-1.,-0.443677556849151));
#32358=CARTESIAN_POINT('Ctrl Pts',(1.90691756144898,1.,-0.443677556849151));
#32359=CARTESIAN_POINT('Ctrl Pts',(1.9120369998112,-1.,-0.446617343485711));
#32360=CARTESIAN_POINT('Ctrl Pts',(1.9120369998112,1.,-0.446617343485711));
#32361=CARTESIAN_POINT('Ctrl Pts',(1.91718342555755,-1.,-0.449632260106662));
#32362=CARTESIAN_POINT('Ctrl Pts',(1.91718342555755,1.,-0.449632260106662));
#32363=CARTESIAN_POINT('Ctrl Pts',(1.92235380648502,-1.,-0.452719478359433));
#32364=CARTESIAN_POINT('Ctrl Pts',(1.92235380648502,1.,-0.452719478359433));
#32365=CARTESIAN_POINT('Ctrl Pts',(1.92753067150476,-1.,-0.455872005174371));
#32366=CARTESIAN_POINT('Ctrl Pts',(1.92753067150476,1.,-0.455872005174371));
#32367=CARTESIAN_POINT('Ctrl Pts',(1.93269066517934,-1.,-0.459081234547926));
#32368=CARTESIAN_POINT('Ctrl Pts',(1.93269066517934,1.,-0.459081234547926));
#32369=CARTESIAN_POINT('Ctrl Pts',(1.93781486640821,-1.,-0.462340031009057));
#32370=CARTESIAN_POINT('Ctrl Pts',(1.93781486640821,1.,-0.462340031009057));
#32371=CARTESIAN_POINT('Ctrl Pts',(1.9428979419619,-1.,-0.46564546202603));
#32372=CARTESIAN_POINT('Ctrl Pts',(1.9428979419619,1.,-0.46564546202603));
#32373=CARTESIAN_POINT('Ctrl Pts',(1.94794381136514,-1.,-0.468997482913135));
#32374=CARTESIAN_POINT('Ctrl Pts',(1.94794381136514,1.,-0.468997482913135));
#32375=CARTESIAN_POINT('Ctrl Pts',(1.95296148278133,-1.,-0.472397672264072));
#32376=CARTESIAN_POINT('Ctrl Pts',(1.95296148278133,1.,-0.472397672264072));
#32377=CARTESIAN_POINT('Ctrl Pts',(1.95796111148177,-1.,-0.475848034683176));
#32378=CARTESIAN_POINT('Ctrl Pts',(1.95796111148177,1.,-0.475848034683176));
#32379=CARTESIAN_POINT('Ctrl Pts',(1.96294933055943,-1.,-0.479349583074855));
#32380=CARTESIAN_POINT('Ctrl Pts',(1.96294933055943,1.,-0.479349583074855));
#32381=CARTESIAN_POINT('Ctrl Pts',(1.96792703422362,-1.,-0.482901662120691));
#32382=CARTESIAN_POINT('Ctrl Pts',(1.96792703422362,1.,-0.482901662120691));
#32383=CARTESIAN_POINT('Ctrl Pts',(1.97289186263272,-1.,-0.486502692907659));
#32384=CARTESIAN_POINT('Ctrl Pts',(1.97289186263272,1.,-0.486502692907659));
#32385=CARTESIAN_POINT('Ctrl Pts',(1.97783973019229,-1.,-0.490150627860953));
#32386=CARTESIAN_POINT('Ctrl Pts',(1.97783973019229,1.,-0.490150627860953));
#32387=CARTESIAN_POINT('Ctrl Pts',(1.98276658761821,-1.,-0.493843476541495));
#32388=CARTESIAN_POINT('Ctrl Pts',(1.98276658761821,1.,-0.493843476541495));
#32389=CARTESIAN_POINT('Ctrl Pts',(1.98767044752932,-1.,-0.497579909545574));
#32390=CARTESIAN_POINT('Ctrl Pts',(1.98767044752932,1.,-0.497579909545574));
#32391=CARTESIAN_POINT('Ctrl Pts',(1.99255149126155,-1.,-0.501359287727146));
#32392=CARTESIAN_POINT('Ctrl Pts',(1.99255149126155,1.,-0.501359287727146));
#32393=CARTESIAN_POINT('Ctrl Pts',(1.99741107463572,-1.,-0.505181361323026));
#32394=CARTESIAN_POINT('Ctrl Pts',(1.99741107463572,1.,-0.505181361323026));
#32395=CARTESIAN_POINT('Ctrl Pts',(2.00225107134734,-1.,-0.509046069886157));
#32396=CARTESIAN_POINT('Ctrl Pts',(2.00225107134734,1.,-0.509046069886157));
#32397=CARTESIAN_POINT('Ctrl Pts',(2.00707309946949,-1.,-0.512953306961793));
#32398=CARTESIAN_POINT('Ctrl Pts',(2.00707309946949,1.,-0.512953306961793));
#32399=CARTESIAN_POINT('Ctrl Pts',(2.01187773939242,-1.,-0.516902681728687));
#32400=CARTESIAN_POINT('Ctrl Pts',(2.01187773939242,1.,-0.516902681728687));
#32401=CARTESIAN_POINT('Ctrl Pts',(2.01666477917286,-1.,-0.520893590399371));
#32402=CARTESIAN_POINT('Ctrl Pts',(2.01666477917286,1.,-0.520893590399371));
#32403=CARTESIAN_POINT('Ctrl Pts',(2.02143356304698,-1.,-0.524925318333476));
#32404=CARTESIAN_POINT('Ctrl Pts',(2.02143356304698,1.,-0.524925318333476));
#32405=CARTESIAN_POINT('Ctrl Pts',(2.0261832908329,-1.,-0.528997127241914));
#32406=CARTESIAN_POINT('Ctrl Pts',(2.0261832908329,1.,-0.528997127241914));
#32407=CARTESIAN_POINT('Ctrl Pts',(2.03091336214426,-1.,-0.533108355132977));
#32408=CARTESIAN_POINT('Ctrl Pts',(2.03091336214426,1.,-0.533108355132977));
#32409=CARTESIAN_POINT('Ctrl Pts',(2.03562362954037,-1.,-0.537258489833262));
#32410=CARTESIAN_POINT('Ctrl Pts',(2.03562362954037,1.,-0.537258489833262));
#32411=CARTESIAN_POINT('Ctrl Pts',(2.04031422690527,-1.,-0.541447120615659));
#32412=CARTESIAN_POINT('Ctrl Pts',(2.04031422690527,1.,-0.541447120615659));
#32413=CARTESIAN_POINT('Ctrl Pts',(2.04498544714588,-1.,-0.54567390381743));
#32414=CARTESIAN_POINT('Ctrl Pts',(2.04498544714588,1.,-0.54567390381743));
#32415=CARTESIAN_POINT('Ctrl Pts',(2.04963761077958,-1.,-0.549938525150295));
#32416=CARTESIAN_POINT('Ctrl Pts',(2.04963761077958,1.,-0.549938525150295));
#32417=CARTESIAN_POINT('Ctrl Pts',(2.05427091604413,-1.,-0.554240657463906));
#32418=CARTESIAN_POINT('Ctrl Pts',(2.05427091604413,1.,-0.554240657463906));
#32419=CARTESIAN_POINT('Ctrl Pts',(2.05888537756462,-1.,-0.558579940185152));
#32420=CARTESIAN_POINT('Ctrl Pts',(2.05888537756462,1.,-0.558579940185152));
#32421=CARTESIAN_POINT('Ctrl Pts',(2.06348090160589,-1.,-0.562955993082262));
#32422=CARTESIAN_POINT('Ctrl Pts',(2.06348090160589,1.,-0.562955993082262));
#32423=CARTESIAN_POINT('Ctrl Pts',(2.06805732997334,-1.,-0.567368421181087));
#32424=CARTESIAN_POINT('Ctrl Pts',(2.06805732997334,1.,-0.567368421181087));
#32425=CARTESIAN_POINT('Ctrl Pts',(2.07261449292824,-1.,-0.571816823242603));
#32426=CARTESIAN_POINT('Ctrl Pts',(2.07261449292824,1.,-0.571816823242603));
#32427=CARTESIAN_POINT('Ctrl Pts',(2.07715226767559,-1.,-0.576300797416845));
#32428=CARTESIAN_POINT('Ctrl Pts',(2.07715226767559,1.,-0.576300797416845));
#32429=CARTESIAN_POINT('Ctrl Pts',(2.08167059018418,-1.,-0.580819952108064));
#32430=CARTESIAN_POINT('Ctrl Pts',(2.08167059018418,1.,-0.580819952108064));
#32431=CARTESIAN_POINT('Ctrl Pts',(2.08616943727951,-1.,-0.585373918991617));
#32432=CARTESIAN_POINT('Ctrl Pts',(2.08616943727951,1.,-0.585373918991617));
#32433=CARTESIAN_POINT('Ctrl Pts',(2.09064881812129,-1.,-0.589962365403406));
#32434=CARTESIAN_POINT('Ctrl Pts',(2.09064881812129,1.,-0.589962365403406));
#32435=CARTESIAN_POINT('Ctrl Pts',(2.0951087622027,-1.,-0.594585006052162));
#32436=CARTESIAN_POINT('Ctrl Pts',(2.0951087622027,1.,-0.594585006052162));
#32437=CARTESIAN_POINT('Ctrl Pts',(2.0995493086477,-1.,-0.599241616420534));
#32438=CARTESIAN_POINT('Ctrl Pts',(2.0995493086477,1.,-0.599241616420534));
#32439=CARTESIAN_POINT('Ctrl Pts',(2.10397049886949,-1.,-0.60393203073603));
#32440=CARTESIAN_POINT('Ctrl Pts',(2.10397049886949,1.,-0.60393203073603));
#32441=CARTESIAN_POINT('Ctrl Pts',(2.1074919961518,-1.,-0.607711315454876));
#32442=CARTESIAN_POINT('Ctrl Pts',(2.1074919961518,1.,-0.607711315454876));
#32443=CARTESIAN_POINT('Ctrl Pts',(2.11012443807238,-1.,-0.610560911689899));
#32444=CARTESIAN_POINT('Ctrl Pts',(2.11012443807238,1.,-0.610560911689899));
#32445=CARTESIAN_POINT('Ctrl Pts',(2.11187554259986,-1.,-0.6124673655618));
#32446=CARTESIAN_POINT('Ctrl Pts',(2.11187554259986,1.,-0.6124673655618));
#32447=CARTESIAN_POINT('Ctrl Pts',(2.11275013067528,-1.,-0.61342227326009));
#32448=CARTESIAN_POINT('Ctrl Pts',(2.11275013067528,1.,-0.61342227326009));
#32449=CARTESIAN_POINT('',(1.7075470150345,1.,-0.383122945602004));
#32450=CARTESIAN_POINT('Ctrl Pts',(1.7075470150345,1.,-0.383122945602004));
#32451=CARTESIAN_POINT('Ctrl Pts',(1.71231062891958,1.,-0.384119047315542));
#32452=CARTESIAN_POINT('Ctrl Pts',(1.72162022246158,1.,-0.38607079032701));
#32453=CARTESIAN_POINT('Ctrl Pts',(1.7349317097561,1.,-0.388877023509192));
#32454=CARTESIAN_POINT('Ctrl Pts',(1.75137405313962,1.,-0.392375812294307));
#32455=CARTESIAN_POINT('Ctrl Pts',(1.7697556004756,1.,-0.39634619612042));
#32456=CARTESIAN_POINT('Ctrl Pts',(1.78598826347533,1.,-0.399919403783081));
#32457=CARTESIAN_POINT('Ctrl Pts',(1.80012077176221,1.,-0.403107976170441));
#32458=CARTESIAN_POINT('Ctrl Pts',(1.81223801813988,1.,-0.405933518411838));
#32459=CARTESIAN_POINT('Ctrl Pts',(1.8224702267854,1.,-0.408428948108534));
#32460=CARTESIAN_POINT('Ctrl Pts',(1.83100408895216,1.,-0.410641256301675));
#32461=CARTESIAN_POINT('Ctrl Pts',(1.83808953475839,1.,-0.412633125322162));
#32462=CARTESIAN_POINT('Ctrl Pts',(1.8440575707371,1.,-0.41448743825434));
#32463=CARTESIAN_POINT('Ctrl Pts',(1.84929312929882,1.,-0.416300022038864));
#32464=CARTESIAN_POINT('Ctrl Pts',(1.85417632856234,1.,-0.418164129143534));
#32465=CARTESIAN_POINT('Ctrl Pts',(1.85903281096686,1.,-0.42015728797562));
#32466=CARTESIAN_POINT('Ctrl Pts',(1.86408083334028,1.,-0.422327307418275));
#32467=CARTESIAN_POINT('Ctrl Pts',(1.86937803944323,1.,-0.424678177291359));
#32468=CARTESIAN_POINT('Ctrl Pts',(1.87486989291484,1.,-0.427183828519102));
#32469=CARTESIAN_POINT('Ctrl Pts',(1.88044229001832,1.,-0.429803062482345));
#32470=CARTESIAN_POINT('Ctrl Pts',(1.88596913666793,1.,-0.432493038548748));
#32471=CARTESIAN_POINT('Ctrl Pts',(1.89136993975504,1.,-0.435225660963383));
#32472=CARTESIAN_POINT('Ctrl Pts',(1.89663648956466,1.,-0.437995003948244));
#32473=CARTESIAN_POINT('Ctrl Pts',(1.90180124389086,1.,-0.440807833704038));
#32474=CARTESIAN_POINT('Ctrl Pts',(1.90691756144898,1.,-0.443677556849151));
#32475=CARTESIAN_POINT('Ctrl Pts',(1.9120369998112,1.,-0.446617343485711));
#32476=CARTESIAN_POINT('Ctrl Pts',(1.91718342555755,1.,-0.449632260106662));
#32477=CARTESIAN_POINT('Ctrl Pts',(1.92235380648502,1.,-0.452719478359433));
#32478=CARTESIAN_POINT('Ctrl Pts',(1.92753067150476,1.,-0.455872005174371));
#32479=CARTESIAN_POINT('Ctrl Pts',(1.93269066517934,1.,-0.459081234547926));
#32480=CARTESIAN_POINT('Ctrl Pts',(1.93781486640821,1.,-0.462340031009057));
#32481=CARTESIAN_POINT('Ctrl Pts',(1.9428979419619,1.,-0.46564546202603));
#32482=CARTESIAN_POINT('Ctrl Pts',(1.94794381136514,1.,-0.468997482913135));
#32483=CARTESIAN_POINT('Ctrl Pts',(1.95296148278133,1.,-0.472397672264072));
#32484=CARTESIAN_POINT('Ctrl Pts',(1.95796111148177,1.,-0.475848034683176));
#32485=CARTESIAN_POINT('Ctrl Pts',(1.96294933055943,1.,-0.479349583074855));
#32486=CARTESIAN_POINT('Ctrl Pts',(1.96792703422362,1.,-0.482901662120691));
#32487=CARTESIAN_POINT('Ctrl Pts',(1.97289186263272,1.,-0.486502692907659));
#32488=CARTESIAN_POINT('Ctrl Pts',(1.97783973019229,1.,-0.490150627860953));
#32489=CARTESIAN_POINT('Ctrl Pts',(1.98276658761821,1.,-0.493843476541495));
#32490=CARTESIAN_POINT('Ctrl Pts',(1.98767044752932,1.,-0.497579909545574));
#32491=CARTESIAN_POINT('Ctrl Pts',(1.99255149126155,1.,-0.501359287727146));
#32492=CARTESIAN_POINT('Ctrl Pts',(1.99741107463572,1.,-0.505181361323026));
#32493=CARTESIAN_POINT('Ctrl Pts',(2.00225107134734,1.,-0.509046069886157));
#32494=CARTESIAN_POINT('Ctrl Pts',(2.00707309946949,1.,-0.512953306961793));
#32495=CARTESIAN_POINT('Ctrl Pts',(2.01187773939242,1.,-0.516902681728687));
#32496=CARTESIAN_POINT('Ctrl Pts',(2.01666477917286,1.,-0.520893590399371));
#32497=CARTESIAN_POINT('Ctrl Pts',(2.02143356304698,1.,-0.524925318333476));
#32498=CARTESIAN_POINT('Ctrl Pts',(2.0261832908329,1.,-0.528997127241914));
#32499=CARTESIAN_POINT('Ctrl Pts',(2.03091336214426,1.,-0.533108355132977));
#32500=CARTESIAN_POINT('Ctrl Pts',(2.03562362954037,1.,-0.537258489833262));
#32501=CARTESIAN_POINT('Ctrl Pts',(2.04031422690527,1.,-0.541447120615659));
#32502=CARTESIAN_POINT('Ctrl Pts',(2.04498544714588,1.,-0.54567390381743));
#32503=CARTESIAN_POINT('Ctrl Pts',(2.04963761077958,1.,-0.549938525150295));
#32504=CARTESIAN_POINT('Ctrl Pts',(2.05427091604413,1.,-0.554240657463906));
#32505=CARTESIAN_POINT('Ctrl Pts',(2.05888537756462,1.,-0.558579940185152));
#32506=CARTESIAN_POINT('Ctrl Pts',(2.06348090160589,1.,-0.562955993082262));
#32507=CARTESIAN_POINT('Ctrl Pts',(2.06805732997334,1.,-0.567368421181087));
#32508=CARTESIAN_POINT('Ctrl Pts',(2.07261449292824,1.,-0.571816823242603));
#32509=CARTESIAN_POINT('Ctrl Pts',(2.07715226767559,1.,-0.576300797416845));
#32510=CARTESIAN_POINT('Ctrl Pts',(2.08167059018418,1.,-0.580819952108064));
#32511=CARTESIAN_POINT('Ctrl Pts',(2.08616943727951,1.,-0.585373918991617));
#32512=CARTESIAN_POINT('Ctrl Pts',(2.09064881812129,1.,-0.589962365403406));
#32513=CARTESIAN_POINT('Ctrl Pts',(2.0951087622027,1.,-0.594585006052162));
#32514=CARTESIAN_POINT('Ctrl Pts',(2.0995493086477,1.,-0.599241616420534));
#32515=CARTESIAN_POINT('Ctrl Pts',(2.10397049886949,1.,-0.60393203073603));
#32516=CARTESIAN_POINT('Ctrl Pts',(2.1074919961518,1.,-0.607711315454876));
#32517=CARTESIAN_POINT('Ctrl Pts',(2.11012443807238,1.,-0.610560911689899));
#32518=CARTESIAN_POINT('Ctrl Pts',(2.11187554259986,1.,-0.6124673655618));
#32519=CARTESIAN_POINT('Ctrl Pts',(2.11275013067528,1.,-0.61342227326009));
#32520=CARTESIAN_POINT('',(1.7075470150345,0.,-0.383122945602001));
#32521=CARTESIAN_POINT('Origin',(0.,0.,0.));
#32522=CARTESIAN_POINT('',(1.74236521665491,1.,-0.163289472382896));
#32523=CARTESIAN_POINT('Origin',(0.,1.,0.));
#32524=CARTESIAN_POINT('',(1.74236521665491,0.,-0.163289472382896));
#32525=CARTESIAN_POINT('Ctrl Pts',(2.19890268624765,-1.,-0.0694764450219582));
#32526=CARTESIAN_POINT('Ctrl Pts',(2.19890268624765,1.,-0.0694764450219582));
#32527=CARTESIAN_POINT('Ctrl Pts',(2.19777582085423,-1.,-0.0701143536325491));
#32528=CARTESIAN_POINT('Ctrl Pts',(2.19777582085423,1.,-0.0701143536325491));
#32529=CARTESIAN_POINT('Ctrl Pts',(2.19552129484002,-1.,-0.0713863779526155));
#32530=CARTESIAN_POINT('Ctrl Pts',(2.19552129484002,1.,-0.0713863779526155));
#32531=CARTESIAN_POINT('Ctrl Pts',(2.19213712013662,-1.,-0.0732830357306726));
#32532=CARTESIAN_POINT('Ctrl Pts',(2.19213712013662,1.,-0.0732830357306726));
#32533=CARTESIAN_POINT('Ctrl Pts',(2.1876201139953,-1.,-0.0757891465836149));
#32534=CARTESIAN_POINT('Ctrl Pts',(2.1876201139953,1.,-0.0757891465836149));
#32535=CARTESIAN_POINT('Ctrl Pts',(2.18196589448887,-1.,-0.0788837727685244));
#32536=CARTESIAN_POINT('Ctrl Pts',(2.18196589448887,1.,-0.0788837727685244));
#32537=CARTESIAN_POINT('Ctrl Pts',(2.176303712113,-1.,-0.0819402680872767));
#32538=CARTESIAN_POINT('Ctrl Pts',(2.176303712113,1.,-0.0819402680872767));
#32539=CARTESIAN_POINT('Ctrl Pts',(2.17063357870952,-1.,-0.0849584620835374));
#32540=CARTESIAN_POINT('Ctrl Pts',(2.17063357870952,1.,-0.0849584620835374));
#32541=CARTESIAN_POINT('Ctrl Pts',(2.16495552645014,-1.,-0.0879381291386924));
#32542=CARTESIAN_POINT('Ctrl Pts',(2.16495552645014,1.,-0.0879381291386924));
#32543=CARTESIAN_POINT('Ctrl Pts',(2.15926961544516,-1.,-0.0908789888107267));
#32544=CARTESIAN_POINT('Ctrl Pts',(2.15926961544516,1.,-0.0908789888107267));
#32545=CARTESIAN_POINT('Ctrl Pts',(2.1535759397817,-1.,-0.0937807218867645));
#32546=CARTESIAN_POINT('Ctrl Pts',(2.1535759397817,1.,-0.0937807218867645));
#32547=CARTESIAN_POINT('Ctrl Pts',(2.14787463531795,-1.,-0.096642985230546));
#32548=CARTESIAN_POINT('Ctrl Pts',(2.14787463531795,1.,-0.096642985230546));
#32549=CARTESIAN_POINT('Ctrl Pts',(2.14216588396025,-1.,-0.0994654261990917));
#32550=CARTESIAN_POINT('Ctrl Pts',(2.14216588396025,1.,-0.0994654261990917));
#32551=CARTESIAN_POINT('Ctrl Pts',(2.13644992667165,-1.,-0.102247700556101));
#32552=CARTESIAN_POINT('Ctrl Pts',(2.13644992667165,1.,-0.102247700556101));
#32553=CARTESIAN_POINT('Ctrl Pts',(2.13072704887293,-1.,-0.10498947915274));
#32554=CARTESIAN_POINT('Ctrl Pts',(2.13072704887293,1.,-0.10498947915274));
#32555=CARTESIAN_POINT('Ctrl Pts',(2.12499752307,-1.,-0.10769043523109));
#32556=CARTESIAN_POINT('Ctrl Pts',(2.12499752307,1.,-0.10769043523109));
#32557=CARTESIAN_POINT('Ctrl Pts',(2.11926155590865,-1.,-0.110350236135025));
#32558=CARTESIAN_POINT('Ctrl Pts',(2.11926155590865,1.,-0.110350236135025));
#32559=CARTESIAN_POINT('Ctrl Pts',(2.11351924490306,-1.,-0.112968534419737));
#32560=CARTESIAN_POINT('Ctrl Pts',(2.11351924490306,1.,-0.112968534419737));
#32561=CARTESIAN_POINT('Ctrl Pts',(2.10777050261309,-1.,-0.115544957687927));
#32562=CARTESIAN_POINT('Ctrl Pts',(2.10777050261309,1.,-0.115544957687927));
#32563=CARTESIAN_POINT('Ctrl Pts',(2.102015121329,-1.,-0.118079107988356));
#32564=CARTESIAN_POINT('Ctrl Pts',(2.102015121329,1.,-0.118079107988356));
#32565=CARTESIAN_POINT('Ctrl Pts',(2.0962529286773,-1.,-0.120570567965122));
#32566=CARTESIAN_POINT('Ctrl Pts',(2.0962529286773,1.,-0.120570567965122));
#32567=CARTESIAN_POINT('Ctrl Pts',(2.09048392424825,-1.,-0.123018905621083));
#32568=CARTESIAN_POINT('Ctrl Pts',(2.09048392424825,1.,-0.123018905621083));
#32569=CARTESIAN_POINT('Ctrl Pts',(2.08470840653643,-1.,-0.125423679412062));
#32570=CARTESIAN_POINT('Ctrl Pts',(2.08470840653643,1.,-0.125423679412062));
#32571=CARTESIAN_POINT('Ctrl Pts',(2.07892715110987,-1.,-0.12778444527612));
#32572=CARTESIAN_POINT('Ctrl Pts',(2.07892715110987,1.,-0.12778444527612));
#32573=CARTESIAN_POINT('Ctrl Pts',(2.07314114713063,-1.,-0.130100748328404));
#32574=CARTESIAN_POINT('Ctrl Pts',(2.07314114713063,1.,-0.130100748328404));
#32575=CARTESIAN_POINT('Ctrl Pts',(2.06735123910326,-1.,-0.132372111547711));
#32576=CARTESIAN_POINT('Ctrl Pts',(2.06735123910326,1.,-0.132372111547711));
#32577=CARTESIAN_POINT('Ctrl Pts',(2.06155781517842,-1.,-0.134598026192106));
#32578=CARTESIAN_POINT('Ctrl Pts',(2.06155781517842,1.,-0.134598026192106));
#32579=CARTESIAN_POINT('Ctrl Pts',(2.05576044414264,-1.,-0.136777941218044));
#32580=CARTESIAN_POINT('Ctrl Pts',(2.05576044414264,1.,-0.136777941218044));
#32581=CARTESIAN_POINT('Ctrl Pts',(2.04995762001328,-1.,-0.138911255368966));
#32582=CARTESIAN_POINT('Ctrl Pts',(2.04995762001328,1.,-0.138911255368966));
#32583=CARTESIAN_POINT('Ctrl Pts',(2.04414757947916,-1.,-0.140997332152546));
#32584=CARTESIAN_POINT('Ctrl Pts',(2.04414757947916,1.,-0.140997332152546));
#32585=CARTESIAN_POINT('Ctrl Pts',(2.03832911025912,-1.,-0.143035515058209));
#32586=CARTESIAN_POINT('Ctrl Pts',(2.03832911025912,1.,-0.143035515058209));
#32587=CARTESIAN_POINT('Ctrl Pts',(2.03250223739942,-1.,-0.145025140186058));
#32588=CARTESIAN_POINT('Ctrl Pts',(2.03250223739942,1.,-0.145025140186058));
#32589=CARTESIAN_POINT('Ctrl Pts',(2.02666926182017,-1.,-0.146965557332583));
#32590=CARTESIAN_POINT('Ctrl Pts',(2.02666926182017,1.,-0.146965557332583));
#32591=CARTESIAN_POINT('Ctrl Pts',(2.02083464969894,-1.,-0.148856124775337));
#32592=CARTESIAN_POINT('Ctrl Pts',(2.02083464969894,1.,-0.148856124775337));
#32593=CARTESIAN_POINT('Ctrl Pts',(2.01500291940238,-1.,-0.150696157673078));
#32594=CARTESIAN_POINT('Ctrl Pts',(2.01500291940238,1.,-0.150696157673078));
#32595=CARTESIAN_POINT('Ctrl Pts',(2.00917680318424,-1.,-0.15248488362145));
#32596=CARTESIAN_POINT('Ctrl Pts',(2.00917680318424,1.,-0.15248488362145));
#32597=CARTESIAN_POINT('Ctrl Pts',(2.00335565310543,-1.,-0.154221403049722));
#32598=CARTESIAN_POINT('Ctrl Pts',(2.00335565310543,1.,-0.154221403049722));
#32599=CARTESIAN_POINT('Ctrl Pts',(1.99753284771497,-1.,-0.155904629548784));
#32600=CARTESIAN_POINT('Ctrl Pts',(1.99753284771497,1.,-0.155904629548784));
#32601=CARTESIAN_POINT('Ctrl Pts',(1.99169810931908,-1.,-0.157533331459227));
#32602=CARTESIAN_POINT('Ctrl Pts',(1.99169810931908,1.,-0.157533331459227));
#32603=CARTESIAN_POINT('Ctrl Pts',(1.98584238283292,-1.,-0.159106226437299));
#32604=CARTESIAN_POINT('Ctrl Pts',(1.98584238283292,1.,-0.159106226437299));
#32605=CARTESIAN_POINT('Ctrl Pts',(1.97996195437559,-1.,-0.160622060784611));
#32606=CARTESIAN_POINT('Ctrl Pts',(1.97996195437559,1.,-0.160622060784611));
#32607=CARTESIAN_POINT('Ctrl Pts',(1.97406280235188,-1.,-0.162079693556289));
#32608=CARTESIAN_POINT('Ctrl Pts',(1.97406280235188,1.,-0.162079693556289));
#32609=CARTESIAN_POINT('Ctrl Pts',(1.96816512677967,-1.,-0.163478185457734));
#32610=CARTESIAN_POINT('Ctrl Pts',(1.96816512677967,1.,-0.163478185457734));
#32611=CARTESIAN_POINT('Ctrl Pts',(1.96229379940136,-1.,-0.164816568920269));
#32612=CARTESIAN_POINT('Ctrl Pts',(1.96229379940136,1.,-0.164816568920269));
#32613=CARTESIAN_POINT('Ctrl Pts',(1.9564675971873,-1.,-0.166093592002813));
#32614=CARTESIAN_POINT('Ctrl Pts',(1.9564675971873,1.,-0.166093592002813));
#32615=CARTESIAN_POINT('Ctrl Pts',(1.95069027794294,-1.,-0.167307501784476));
#32616=CARTESIAN_POINT('Ctrl Pts',(1.95069027794294,1.,-0.167307501784476));
#32617=CARTESIAN_POINT('Ctrl Pts',(1.94493757756931,-1.,-0.168455741607556));
#32618=CARTESIAN_POINT('Ctrl Pts',(1.94493757756931,1.,-0.168455741607556));
#32619=CARTESIAN_POINT('Ctrl Pts',(1.93915639211581,-1.,-0.169534904817491));
#32620=CARTESIAN_POINT('Ctrl Pts',(1.93915639211581,1.,-0.169534904817491));
#32621=CARTESIAN_POINT('Ctrl Pts',(1.93329183155539,-1.,-0.170541253116202));
#32622=CARTESIAN_POINT('Ctrl Pts',(1.93329183155539,1.,-0.170541253116202));
#32623=CARTESIAN_POINT('Ctrl Pts',(1.92731093582036,-1.,-0.171471191532988));
#32624=CARTESIAN_POINT('Ctrl Pts',(1.92731093582036,1.,-0.171471191532988));
#32625=CARTESIAN_POINT('Ctrl Pts',(1.9212233439798,-1.,-0.172321621259514));
#32626=CARTESIAN_POINT('Ctrl Pts',(1.9212233439798,1.,-0.172321621259514));
#32627=CARTESIAN_POINT('Ctrl Pts',(1.91511429159527,-1.,-0.173090695383496));
#32628=CARTESIAN_POINT('Ctrl Pts',(1.91511429159527,1.,-0.173090695383496));
#32629=CARTESIAN_POINT('Ctrl Pts',(1.90911693975267,-1.,-0.173776635257817));
#32630=CARTESIAN_POINT('Ctrl Pts',(1.90911693975267,1.,-0.173776635257817));
#32631=CARTESIAN_POINT('Ctrl Pts',(1.90335253862834,-1.,-0.174375518661085));
#32632=CARTESIAN_POINT('Ctrl Pts',(1.90335253862834,1.,-0.174375518661085));
#32633=CARTESIAN_POINT('Ctrl Pts',(1.89788101117132,-1.,-0.174879405091263));
#32634=CARTESIAN_POINT('Ctrl Pts',(1.89788101117132,1.,-0.174879405091263));
#32635=CARTESIAN_POINT('Ctrl Pts',(1.892646301985,-1.,-0.175274276190844));
#32636=CARTESIAN_POINT('Ctrl Pts',(1.892646301985,1.,-0.175274276190844));
#32637=CARTESIAN_POINT('Ctrl Pts',(1.88742606273259,-1.,-0.175538155840648));
#32638=CARTESIAN_POINT('Ctrl Pts',(1.88742606273259,1.,-0.175538155840648));
#32639=CARTESIAN_POINT('Ctrl Pts',(1.88188663145367,-1.,-0.175644148889699));
#32640=CARTESIAN_POINT('Ctrl Pts',(1.88188663145367,1.,-0.175644148889699));
#32641=CARTESIAN_POINT('Ctrl Pts',(1.87563767773588,-1.,-0.175563480746485));
#32642=CARTESIAN_POINT('Ctrl Pts',(1.87563767773588,1.,-0.175563480746485));
#32643=CARTESIAN_POINT('Ctrl Pts',(1.86828349694799,-1.,-0.175268337590758));
#32644=CARTESIAN_POINT('Ctrl Pts',(1.86828349694799,1.,-0.175268337590758));
#32645=CARTESIAN_POINT('Ctrl Pts',(1.85948367088837,-1.,-0.17473525927603));
#32646=CARTESIAN_POINT('Ctrl Pts',(1.85948367088837,1.,-0.17473525927603));
#32647=CARTESIAN_POINT('Ctrl Pts',(1.8489811319852,-1.,-0.173946627587732));
#32648=CARTESIAN_POINT('Ctrl Pts',(1.8489811319852,1.,-0.173946627587732));
#32649=CARTESIAN_POINT('Ctrl Pts',(1.83658380527692,-1.,-0.1728894428919));
#32650=CARTESIAN_POINT('Ctrl Pts',(1.83658380527692,1.,-0.1728894428919));
#32651=CARTESIAN_POINT('Ctrl Pts',(1.82215766811545,-1.,-0.171554770204119));
#32652=CARTESIAN_POINT('Ctrl Pts',(1.82215766811545,1.,-0.171554770204119));
#32653=CARTESIAN_POINT('Ctrl Pts',(1.80561530629706,-1.,-0.169936923904608));
#32654=CARTESIAN_POINT('Ctrl Pts',(1.80561530629706,1.,-0.169936923904608));
#32655=CARTESIAN_POINT('Ctrl Pts',(1.7869064998507,-1.,-0.168032772805197));
#32656=CARTESIAN_POINT('Ctrl Pts',(1.7869064998507,1.,-0.168032772805197));
#32657=CARTESIAN_POINT('Ctrl Pts',(1.77018771684844,-1.,-0.1662793551464));
#32658=CARTESIAN_POINT('Ctrl Pts',(1.77018771684844,1.,-0.1662793551464));
#32659=CARTESIAN_POINT('Ctrl Pts',(1.75666056638427,-1.,-0.164834765707159));
#32660=CARTESIAN_POINT('Ctrl Pts',(1.75666056638427,1.,-0.164834765707159));
#32661=CARTESIAN_POINT('Ctrl Pts',(1.7472034950333,-1.,-0.163814161002002));
#32662=CARTESIAN_POINT('Ctrl Pts',(1.7472034950333,1.,-0.163814161002002));
#32663=CARTESIAN_POINT('Ctrl Pts',(1.74236521665491,-1.,-0.163289472382896));
#32664=CARTESIAN_POINT('Ctrl Pts',(1.74236521665491,1.,-0.163289472382896));
#32665=CARTESIAN_POINT('',(2.19890268624765,1.,-0.0694764450219582));
#32666=CARTESIAN_POINT('Ctrl Pts',(2.19890268624765,1.,-0.0694764450219582));
#32667=CARTESIAN_POINT('Ctrl Pts',(2.19777582085423,1.,-0.0701143536325491));
#32668=CARTESIAN_POINT('Ctrl Pts',(2.19552129484002,1.,-0.0713863779526155));
#32669=CARTESIAN_POINT('Ctrl Pts',(2.19213712013662,1.,-0.0732830357306726));
#32670=CARTESIAN_POINT('Ctrl Pts',(2.1876201139953,1.,-0.0757891465836149));
#32671=CARTESIAN_POINT('Ctrl Pts',(2.18196589448887,1.,-0.0788837727685244));
#32672=CARTESIAN_POINT('Ctrl Pts',(2.176303712113,1.,-0.0819402680872767));
#32673=CARTESIAN_POINT('Ctrl Pts',(2.17063357870952,1.,-0.0849584620835374));
#32674=CARTESIAN_POINT('Ctrl Pts',(2.16495552645014,1.,-0.0879381291386924));
#32675=CARTESIAN_POINT('Ctrl Pts',(2.15926961544516,1.,-0.0908789888107267));
#32676=CARTESIAN_POINT('Ctrl Pts',(2.1535759397817,1.,-0.0937807218867645));
#32677=CARTESIAN_POINT('Ctrl Pts',(2.14787463531795,1.,-0.096642985230546));
#32678=CARTESIAN_POINT('Ctrl Pts',(2.14216588396025,1.,-0.0994654261990917));
#32679=CARTESIAN_POINT('Ctrl Pts',(2.13644992667165,1.,-0.102247700556101));
#32680=CARTESIAN_POINT('Ctrl Pts',(2.13072704887293,1.,-0.10498947915274));
#32681=CARTESIAN_POINT('Ctrl Pts',(2.12499752307,1.,-0.10769043523109));
#32682=CARTESIAN_POINT('Ctrl Pts',(2.11926155590865,1.,-0.110350236135025));
#32683=CARTESIAN_POINT('Ctrl Pts',(2.11351924490306,1.,-0.112968534419737));
#32684=CARTESIAN_POINT('Ctrl Pts',(2.10777050261309,1.,-0.115544957687927));
#32685=CARTESIAN_POINT('Ctrl Pts',(2.102015121329,1.,-0.118079107988356));
#32686=CARTESIAN_POINT('Ctrl Pts',(2.0962529286773,1.,-0.120570567965122));
#32687=CARTESIAN_POINT('Ctrl Pts',(2.09048392424825,1.,-0.123018905621083));
#32688=CARTESIAN_POINT('Ctrl Pts',(2.08470840653643,1.,-0.125423679412062));
#32689=CARTESIAN_POINT('Ctrl Pts',(2.07892715110987,1.,-0.12778444527612));
#32690=CARTESIAN_POINT('Ctrl Pts',(2.07314114713063,1.,-0.130100748328404));
#32691=CARTESIAN_POINT('Ctrl Pts',(2.06735123910326,1.,-0.132372111547711));
#32692=CARTESIAN_POINT('Ctrl Pts',(2.06155781517842,1.,-0.134598026192106));
#32693=CARTESIAN_POINT('Ctrl Pts',(2.05576044414264,1.,-0.136777941218044));
#32694=CARTESIAN_POINT('Ctrl Pts',(2.04995762001328,1.,-0.138911255368966));
#32695=CARTESIAN_POINT('Ctrl Pts',(2.04414757947916,1.,-0.140997332152546));
#32696=CARTESIAN_POINT('Ctrl Pts',(2.03832911025912,1.,-0.143035515058209));
#32697=CARTESIAN_POINT('Ctrl Pts',(2.03250223739942,1.,-0.145025140186058));
#32698=CARTESIAN_POINT('Ctrl Pts',(2.02666926182017,1.,-0.146965557332583));
#32699=CARTESIAN_POINT('Ctrl Pts',(2.02083464969894,1.,-0.148856124775337));
#32700=CARTESIAN_POINT('Ctrl Pts',(2.01500291940238,1.,-0.150696157673078));
#32701=CARTESIAN_POINT('Ctrl Pts',(2.00917680318424,1.,-0.15248488362145));
#32702=CARTESIAN_POINT('Ctrl Pts',(2.00335565310543,1.,-0.154221403049722));
#32703=CARTESIAN_POINT('Ctrl Pts',(1.99753284771497,1.,-0.155904629548784));
#32704=CARTESIAN_POINT('Ctrl Pts',(1.99169810931908,1.,-0.157533331459227));
#32705=CARTESIAN_POINT('Ctrl Pts',(1.98584238283292,1.,-0.159106226437299));
#32706=CARTESIAN_POINT('Ctrl Pts',(1.97996195437559,1.,-0.160622060784611));
#32707=CARTESIAN_POINT('Ctrl Pts',(1.97406280235188,1.,-0.162079693556289));
#32708=CARTESIAN_POINT('Ctrl Pts',(1.96816512677967,1.,-0.163478185457734));
#32709=CARTESIAN_POINT('Ctrl Pts',(1.96229379940136,1.,-0.164816568920269));
#32710=CARTESIAN_POINT('Ctrl Pts',(1.9564675971873,1.,-0.166093592002813));
#32711=CARTESIAN_POINT('Ctrl Pts',(1.95069027794294,1.,-0.167307501784476));
#32712=CARTESIAN_POINT('Ctrl Pts',(1.94493757756931,1.,-0.168455741607556));
#32713=CARTESIAN_POINT('Ctrl Pts',(1.93915639211581,1.,-0.169534904817491));
#32714=CARTESIAN_POINT('Ctrl Pts',(1.93329183155539,1.,-0.170541253116202));
#32715=CARTESIAN_POINT('Ctrl Pts',(1.92731093582036,1.,-0.171471191532988));
#32716=CARTESIAN_POINT('Ctrl Pts',(1.9212233439798,1.,-0.172321621259514));
#32717=CARTESIAN_POINT('Ctrl Pts',(1.91511429159527,1.,-0.173090695383496));
#32718=CARTESIAN_POINT('Ctrl Pts',(1.90911693975267,1.,-0.173776635257817));
#32719=CARTESIAN_POINT('Ctrl Pts',(1.90335253862834,1.,-0.174375518661085));
#32720=CARTESIAN_POINT('Ctrl Pts',(1.89788101117132,1.,-0.174879405091263));
#32721=CARTESIAN_POINT('Ctrl Pts',(1.892646301985,1.,-0.175274276190844));
#32722=CARTESIAN_POINT('Ctrl Pts',(1.88742606273259,1.,-0.175538155840648));
#32723=CARTESIAN_POINT('Ctrl Pts',(1.88188663145367,1.,-0.175644148889699));
#32724=CARTESIAN_POINT('Ctrl Pts',(1.87563767773588,1.,-0.175563480746485));
#32725=CARTESIAN_POINT('Ctrl Pts',(1.86828349694799,1.,-0.175268337590758));
#32726=CARTESIAN_POINT('Ctrl Pts',(1.85948367088837,1.,-0.17473525927603));
#32727=CARTESIAN_POINT('Ctrl Pts',(1.8489811319852,1.,-0.173946627587732));
#32728=CARTESIAN_POINT('Ctrl Pts',(1.83658380527692,1.,-0.1728894428919));
#32729=CARTESIAN_POINT('Ctrl Pts',(1.82215766811545,1.,-0.171554770204119));
#32730=CARTESIAN_POINT('Ctrl Pts',(1.80561530629706,1.,-0.169936923904608));
#32731=CARTESIAN_POINT('Ctrl Pts',(1.7869064998507,1.,-0.168032772805197));
#32732=CARTESIAN_POINT('Ctrl Pts',(1.77018771684844,1.,-0.1662793551464));
#32733=CARTESIAN_POINT('Ctrl Pts',(1.75666056638427,1.,-0.164834765707159));
#32734=CARTESIAN_POINT('Ctrl Pts',(1.7472034950333,1.,-0.163814161002002));
#32735=CARTESIAN_POINT('Ctrl Pts',(1.74236521665491,1.,-0.163289472382896));
#32736=CARTESIAN_POINT('',(2.19890268624765,0.,-0.0694764450219582));
#32737=CARTESIAN_POINT('Origin',(2.19890268624765,0.,0.0694764450219582));
#32738=CARTESIAN_POINT('',(2.19890268624765,1.,0.0694764450219582));
#32739=CARTESIAN_POINT('',(2.19890268624765,1.,-0.0694764450219582));
#32740=CARTESIAN_POINT('',(2.19890268624765,0.,0.0694764450219582));
#32741=CARTESIAN_POINT('Ctrl Pts',(1.74236521665491,-1.,0.163289472382896));
#32742=CARTESIAN_POINT('Ctrl Pts',(1.74236521665491,1.,0.163289472382896));
#32743=CARTESIAN_POINT('Ctrl Pts',(1.74720349503904,-1.,0.163814161002474));
#32744=CARTESIAN_POINT('Ctrl Pts',(1.74720349503904,1.,0.163814161002474));
#32745=CARTESIAN_POINT('Ctrl Pts',(1.75666056640041,-1.,0.164834765708484));
#32746=CARTESIAN_POINT('Ctrl Pts',(1.75666056640041,1.,0.164834765708484));
#32747=CARTESIAN_POINT('Ctrl Pts',(1.77018771687692,-1.,0.166279355148738));
#32748=CARTESIAN_POINT('Ctrl Pts',(1.77018771687692,1.,0.166279355148738));
#32749=CARTESIAN_POINT('Ctrl Pts',(1.78690649988931,-1.,0.16803277280837));
#32750=CARTESIAN_POINT('Ctrl Pts',(1.78690649988931,1.,0.16803277280837));
#32751=CARTESIAN_POINT('Ctrl Pts',(1.80561530633924,-1.,0.169936923908078));
#32752=CARTESIAN_POINT('Ctrl Pts',(1.80561530633924,1.,0.169936923908078));
#32753=CARTESIAN_POINT('Ctrl Pts',(1.82215766815414,-1.,0.171554770207306));
#32754=CARTESIAN_POINT('Ctrl Pts',(1.82215766815414,1.,0.171554770207306));
#32755=CARTESIAN_POINT('Ctrl Pts',(1.83658380530747,-1.,0.17288944289442));
#32756=CARTESIAN_POINT('Ctrl Pts',(1.83658380530747,1.,0.17288944289442));
#32757=CARTESIAN_POINT('Ctrl Pts',(1.84898113200543,-1.,0.173946627589401));
#32758=CARTESIAN_POINT('Ctrl Pts',(1.84898113200543,1.,0.173946627589401));
#32759=CARTESIAN_POINT('Ctrl Pts',(1.85948367089838,-1.,0.174735259276856));
#32760=CARTESIAN_POINT('Ctrl Pts',(1.85948367089838,1.,0.174735259276856));
#32761=CARTESIAN_POINT('Ctrl Pts',(1.86828349694972,-1.,0.1752683375909));
#32762=CARTESIAN_POINT('Ctrl Pts',(1.86828349694972,1.,0.1752683375909));
#32763=CARTESIAN_POINT('Ctrl Pts',(1.87563767773249,-1.,0.175563480746205));
#32764=CARTESIAN_POINT('Ctrl Pts',(1.87563767773249,1.,0.175563480746205));
#32765=CARTESIAN_POINT('Ctrl Pts',(1.88188663144846,-1.,0.175644148889271));
#32766=CARTESIAN_POINT('Ctrl Pts',(1.88188663144846,1.,0.175644148889271));
#32767=CARTESIAN_POINT('Ctrl Pts',(1.88742606272818,-1.,0.175538155840286));
#32768=CARTESIAN_POINT('Ctrl Pts',(1.88742606272818,1.,0.175538155840286));
#32769=CARTESIAN_POINT('Ctrl Pts',(1.89264630198279,-1.,0.175274276190664));
#32770=CARTESIAN_POINT('Ctrl Pts',(1.89264630198279,1.,0.175274276190664));
#32771=CARTESIAN_POINT('Ctrl Pts',(1.89788101117148,-1.,0.174879405091277));
#32772=CARTESIAN_POINT('Ctrl Pts',(1.89788101117148,1.,0.174879405091277));
#32773=CARTESIAN_POINT('Ctrl Pts',(1.90335253863003,-1.,0.174375518661222));
#32774=CARTESIAN_POINT('Ctrl Pts',(1.90335253863003,1.,0.174375518661222));
#32775=CARTESIAN_POINT('Ctrl Pts',(1.90911693975475,-1.,0.173776635257983));
#32776=CARTESIAN_POINT('Ctrl Pts',(1.90911693975475,1.,0.173776635257983));
#32777=CARTESIAN_POINT('Ctrl Pts',(1.91511429159681,-1.,0.173090695383619));
#32778=CARTESIAN_POINT('Ctrl Pts',(1.91511429159681,1.,0.173090695383619));
#32779=CARTESIAN_POINT('Ctrl Pts',(1.92122334398034,-1.,0.172321621259556));
#32780=CARTESIAN_POINT('Ctrl Pts',(1.92122334398034,1.,0.172321621259556));
#32781=CARTESIAN_POINT('Ctrl Pts',(1.92731093582,-1.,0.17147119153296));
#32782=CARTESIAN_POINT('Ctrl Pts',(1.92731093582,1.,0.17147119153296));
#32783=CARTESIAN_POINT('Ctrl Pts',(1.93329183155455,-1.,0.170541253116136));
#32784=CARTESIAN_POINT('Ctrl Pts',(1.93329183155455,1.,0.170541253116136));
#32785=CARTESIAN_POINT('Ctrl Pts',(1.93915639211497,-1.,0.169534904817425));
#32786=CARTESIAN_POINT('Ctrl Pts',(1.93915639211497,1.,0.169534904817425));
#32787=CARTESIAN_POINT('Ctrl Pts',(1.94493757756879,-1.,0.168455741607515));
#32788=CARTESIAN_POINT('Ctrl Pts',(1.94493757756879,1.,0.168455741607515));
#32789=CARTESIAN_POINT('Ctrl Pts',(1.95069027794286,-1.,0.167307501784469));
#32790=CARTESIAN_POINT('Ctrl Pts',(1.95069027794286,1.,0.167307501784469));
#32791=CARTESIAN_POINT('Ctrl Pts',(1.95646759718755,-1.,0.166093592002832));
#32792=CARTESIAN_POINT('Ctrl Pts',(1.95646759718755,1.,0.166093592002832));
#32793=CARTESIAN_POINT('Ctrl Pts',(1.96229379940174,-1.,0.1648165689203));
#32794=CARTESIAN_POINT('Ctrl Pts',(1.96229379940174,1.,0.1648165689203));
#32795=CARTESIAN_POINT('Ctrl Pts',(1.96816512678,-1.,0.16347818545776));
#32796=CARTESIAN_POINT('Ctrl Pts',(1.96816512678,1.,0.16347818545776));
#32797=CARTESIAN_POINT('Ctrl Pts',(1.97406280235204,-1.,0.162079693556302));
#32798=CARTESIAN_POINT('Ctrl Pts',(1.97406280235204,1.,0.162079693556302));
#32799=CARTESIAN_POINT('Ctrl Pts',(1.97996195437557,-1.,0.16062206078461));
#32800=CARTESIAN_POINT('Ctrl Pts',(1.97996195437557,1.,0.16062206078461));
#32801=CARTESIAN_POINT('Ctrl Pts',(1.98584238283279,-1.,0.159106226437288));
#32802=CARTESIAN_POINT('Ctrl Pts',(1.98584238283279,1.,0.159106226437288));
#32803=CARTESIAN_POINT('Ctrl Pts',(1.99169810931893,-1.,0.157533331459215));
#32804=CARTESIAN_POINT('Ctrl Pts',(1.99169810931893,1.,0.157533331459215));
#32805=CARTESIAN_POINT('Ctrl Pts',(1.99753284771487,-1.,0.155904629548774));
#32806=CARTESIAN_POINT('Ctrl Pts',(1.99753284771487,1.,0.155904629548774));
#32807=CARTESIAN_POINT('Ctrl Pts',(2.00335565310539,-1.,0.154221403049719));
#32808=CARTESIAN_POINT('Ctrl Pts',(2.00335565310539,1.,0.154221403049719));
#32809=CARTESIAN_POINT('Ctrl Pts',(2.00917680318426,-1.,0.152484883621452));
#32810=CARTESIAN_POINT('Ctrl Pts',(2.00917680318426,1.,0.152484883621452));
#32811=CARTESIAN_POINT('Ctrl Pts',(2.01500291940243,-1.,0.150696157673084));
#32812=CARTESIAN_POINT('Ctrl Pts',(2.01500291940243,1.,0.150696157673084));
#32813=CARTESIAN_POINT('Ctrl Pts',(2.02083464969897,-1.,0.148856124775342));
#32814=CARTESIAN_POINT('Ctrl Pts',(2.02083464969897,1.,0.148856124775342));
#32815=CARTESIAN_POINT('Ctrl Pts',(2.02666926182017,-1.,0.146965557332586));
#32816=CARTESIAN_POINT('Ctrl Pts',(2.02666926182017,1.,0.146965557332586));
#32817=CARTESIAN_POINT('Ctrl Pts',(2.03250223739941,-1.,0.145025140186058));
#32818=CARTESIAN_POINT('Ctrl Pts',(2.03250223739941,1.,0.145025140186058));
#32819=CARTESIAN_POINT('Ctrl Pts',(2.03832911025913,-1.,0.143035515058208));
#32820=CARTESIAN_POINT('Ctrl Pts',(2.03832911025913,1.,0.143035515058208));
#32821=CARTESIAN_POINT('Ctrl Pts',(2.04414757947919,-1.,0.140997332152545));
#32822=CARTESIAN_POINT('Ctrl Pts',(2.04414757947919,1.,0.140997332152545));
#32823=CARTESIAN_POINT('Ctrl Pts',(2.04995762001333,-1.,0.138911255368966));
#32824=CARTESIAN_POINT('Ctrl Pts',(2.04995762001333,1.,0.138911255368966));
#32825=CARTESIAN_POINT('Ctrl Pts',(2.0557604441427,-1.,0.136777941218044));
#32826=CARTESIAN_POINT('Ctrl Pts',(2.0557604441427,1.,0.136777941218044));
#32827=CARTESIAN_POINT('Ctrl Pts',(2.06155781517844,-1.,0.134598026192107));
#32828=CARTESIAN_POINT('Ctrl Pts',(2.06155781517844,1.,0.134598026192107));
#32829=CARTESIAN_POINT('Ctrl Pts',(2.06735123910319,-1.,0.132372111547709));
#32830=CARTESIAN_POINT('Ctrl Pts',(2.06735123910319,1.,0.132372111547709));
#32831=CARTESIAN_POINT('Ctrl Pts',(2.07314114713047,-1.,0.1301007483284));
#32832=CARTESIAN_POINT('Ctrl Pts',(2.07314114713047,1.,0.1301007483284));
#32833=CARTESIAN_POINT('Ctrl Pts',(2.07892715110967,-1.,0.127784445276116));
#32834=CARTESIAN_POINT('Ctrl Pts',(2.07892715110967,1.,0.127784445276116));
#32835=CARTESIAN_POINT('Ctrl Pts',(2.08470840653628,-1.,0.125423679412058));
#32836=CARTESIAN_POINT('Ctrl Pts',(2.08470840653628,1.,0.125423679412058));
#32837=CARTESIAN_POINT('Ctrl Pts',(2.09048392424826,-1.,0.123018905621083));
#32838=CARTESIAN_POINT('Ctrl Pts',(2.09048392424826,1.,0.123018905621083));
#32839=CARTESIAN_POINT('Ctrl Pts',(2.09625292867756,-1.,0.120570567965129));
#32840=CARTESIAN_POINT('Ctrl Pts',(2.09625292867756,1.,0.120570567965129));
#32841=CARTESIAN_POINT('Ctrl Pts',(2.10201512132945,-1.,0.118079107988368));
#32842=CARTESIAN_POINT('Ctrl Pts',(2.10201512132945,1.,0.118079107988368));
#32843=CARTESIAN_POINT('Ctrl Pts',(2.10777050261359,-1.,0.11554495768794));
#32844=CARTESIAN_POINT('Ctrl Pts',(2.10777050261359,1.,0.11554495768794));
#32845=CARTESIAN_POINT('Ctrl Pts',(2.11351924490335,-1.,0.112968534419746));
#32846=CARTESIAN_POINT('Ctrl Pts',(2.11351924490335,1.,0.112968534419746));
#32847=CARTESIAN_POINT('Ctrl Pts',(2.11926155590849,-1.,0.11035023613502));
#32848=CARTESIAN_POINT('Ctrl Pts',(2.11926155590849,1.,0.11035023613502));
#32849=CARTESIAN_POINT('Ctrl Pts',(2.12499752306927,-1.,0.107690435231068));
#32850=CARTESIAN_POINT('Ctrl Pts',(2.12499752306927,1.,0.107690435231068));
#32851=CARTESIAN_POINT('Ctrl Pts',(2.1307270488718,-1.,0.104989479152703));
#32852=CARTESIAN_POINT('Ctrl Pts',(2.1307270488718,1.,0.104989479152703));
#32853=CARTESIAN_POINT('Ctrl Pts',(2.13644992667052,-1.,0.102247700556063));
#32854=CARTESIAN_POINT('Ctrl Pts',(2.13644992667052,1.,0.102247700556063));
#32855=CARTESIAN_POINT('Ctrl Pts',(2.14216588395974,-1.,0.0994654261990741));
#32856=CARTESIAN_POINT('Ctrl Pts',(2.14216588395974,1.,0.0994654261990741));
#32857=CARTESIAN_POINT('Ctrl Pts',(2.14787463531864,-1.,0.0966429852305688));
#32858=CARTESIAN_POINT('Ctrl Pts',(2.14787463531864,1.,0.0966429852305688));
#32859=CARTESIAN_POINT('Ctrl Pts',(2.15357593978377,-1.,0.0937807218868344));
#32860=CARTESIAN_POINT('Ctrl Pts',(2.15357593978377,1.,0.0937807218868344));
#32861=CARTESIAN_POINT('Ctrl Pts',(2.15926961544808,-1.,0.0908789888108265));
#32862=CARTESIAN_POINT('Ctrl Pts',(2.15926961544808,1.,0.0908789888108265));
#32863=CARTESIAN_POINT('Ctrl Pts',(2.16495552645275,-1.,0.0879381291387821));
#32864=CARTESIAN_POINT('Ctrl Pts',(2.16495552645275,1.,0.0879381291387821));
#32865=CARTESIAN_POINT('Ctrl Pts',(2.17063357871031,-1.,0.0849584620835642));
#32866=CARTESIAN_POINT('Ctrl Pts',(2.17063357871031,1.,0.0849584620835642));
#32867=CARTESIAN_POINT('Ctrl Pts',(2.1763037121106,-1.,0.0819402680871938));
#32868=CARTESIAN_POINT('Ctrl Pts',(2.1763037121106,1.,0.0819402680871938));
#32869=CARTESIAN_POINT('Ctrl Pts',(2.18196589448304,-1.,0.0788837727683226));
#32870=CARTESIAN_POINT('Ctrl Pts',(2.18196589448304,1.,0.0788837727683226));
#32871=CARTESIAN_POINT('Ctrl Pts',(2.1876201139874,-1.,0.075789146583341));
#32872=CARTESIAN_POINT('Ctrl Pts',(2.1876201139874,1.,0.075789146583341));
#32873=CARTESIAN_POINT('Ctrl Pts',(2.19213712012956,-1.,0.0732830357304275));
#32874=CARTESIAN_POINT('Ctrl Pts',(2.19213712012956,1.,0.0732830357304275));
#32875=CARTESIAN_POINT('Ctrl Pts',(2.19552129483562,-1.,0.0713863779524626));
#32876=CARTESIAN_POINT('Ctrl Pts',(2.19552129483562,1.,0.0713863779524626));
#32877=CARTESIAN_POINT('Ctrl Pts',(2.19777582085261,-1.,0.0701143536324925));
#32878=CARTESIAN_POINT('Ctrl Pts',(2.19777582085261,1.,0.0701143536324925));
#32879=CARTESIAN_POINT('Ctrl Pts',(2.19890268624765,-1.,0.0694764450219582));
#32880=CARTESIAN_POINT('Ctrl Pts',(2.19890268624765,1.,0.0694764450219582));
#32881=CARTESIAN_POINT('',(1.74236521665491,1.,0.163289472382896));
#32882=CARTESIAN_POINT('Ctrl Pts',(1.74236521665491,1.,0.163289472382896));
#32883=CARTESIAN_POINT('Ctrl Pts',(1.74720349503904,1.,0.163814161002474));
#32884=CARTESIAN_POINT('Ctrl Pts',(1.75666056640041,1.,0.164834765708484));
#32885=CARTESIAN_POINT('Ctrl Pts',(1.77018771687692,1.,0.166279355148738));
#32886=CARTESIAN_POINT('Ctrl Pts',(1.78690649988931,1.,0.16803277280837));
#32887=CARTESIAN_POINT('Ctrl Pts',(1.80561530633924,1.,0.169936923908078));
#32888=CARTESIAN_POINT('Ctrl Pts',(1.82215766815414,1.,0.171554770207306));
#32889=CARTESIAN_POINT('Ctrl Pts',(1.83658380530747,1.,0.17288944289442));
#32890=CARTESIAN_POINT('Ctrl Pts',(1.84898113200543,1.,0.173946627589401));
#32891=CARTESIAN_POINT('Ctrl Pts',(1.85948367089838,1.,0.174735259276856));
#32892=CARTESIAN_POINT('Ctrl Pts',(1.86828349694972,1.,0.1752683375909));
#32893=CARTESIAN_POINT('Ctrl Pts',(1.87563767773249,1.,0.175563480746205));
#32894=CARTESIAN_POINT('Ctrl Pts',(1.88188663144846,1.,0.175644148889271));
#32895=CARTESIAN_POINT('Ctrl Pts',(1.88742606272818,1.,0.175538155840286));
#32896=CARTESIAN_POINT('Ctrl Pts',(1.89264630198279,1.,0.175274276190664));
#32897=CARTESIAN_POINT('Ctrl Pts',(1.89788101117148,1.,0.174879405091277));
#32898=CARTESIAN_POINT('Ctrl Pts',(1.90335253863003,1.,0.174375518661222));
#32899=CARTESIAN_POINT('Ctrl Pts',(1.90911693975475,1.,0.173776635257983));
#32900=CARTESIAN_POINT('Ctrl Pts',(1.91511429159681,1.,0.173090695383619));
#32901=CARTESIAN_POINT('Ctrl Pts',(1.92122334398034,1.,0.172321621259556));
#32902=CARTESIAN_POINT('Ctrl Pts',(1.92731093582,1.,0.17147119153296));
#32903=CARTESIAN_POINT('Ctrl Pts',(1.93329183155455,1.,0.170541253116136));
#32904=CARTESIAN_POINT('Ctrl Pts',(1.93915639211497,1.,0.169534904817425));
#32905=CARTESIAN_POINT('Ctrl Pts',(1.94493757756879,1.,0.168455741607515));
#32906=CARTESIAN_POINT('Ctrl Pts',(1.95069027794286,1.,0.167307501784469));
#32907=CARTESIAN_POINT('Ctrl Pts',(1.95646759718755,1.,0.166093592002832));
#32908=CARTESIAN_POINT('Ctrl Pts',(1.96229379940174,1.,0.1648165689203));
#32909=CARTESIAN_POINT('Ctrl Pts',(1.96816512678,1.,0.16347818545776));
#32910=CARTESIAN_POINT('Ctrl Pts',(1.97406280235204,1.,0.162079693556302));
#32911=CARTESIAN_POINT('Ctrl Pts',(1.97996195437557,1.,0.16062206078461));
#32912=CARTESIAN_POINT('Ctrl Pts',(1.98584238283279,1.,0.159106226437288));
#32913=CARTESIAN_POINT('Ctrl Pts',(1.99169810931893,1.,0.157533331459215));
#32914=CARTESIAN_POINT('Ctrl Pts',(1.99753284771487,1.,0.155904629548774));
#32915=CARTESIAN_POINT('Ctrl Pts',(2.00335565310539,1.,0.154221403049719));
#32916=CARTESIAN_POINT('Ctrl Pts',(2.00917680318426,1.,0.152484883621452));
#32917=CARTESIAN_POINT('Ctrl Pts',(2.01500291940243,1.,0.150696157673084));
#32918=CARTESIAN_POINT('Ctrl Pts',(2.02083464969897,1.,0.148856124775342));
#32919=CARTESIAN_POINT('Ctrl Pts',(2.02666926182017,1.,0.146965557332586));
#32920=CARTESIAN_POINT('Ctrl Pts',(2.03250223739941,1.,0.145025140186058));
#32921=CARTESIAN_POINT('Ctrl Pts',(2.03832911025913,1.,0.143035515058208));
#32922=CARTESIAN_POINT('Ctrl Pts',(2.04414757947919,1.,0.140997332152545));
#32923=CARTESIAN_POINT('Ctrl Pts',(2.04995762001333,1.,0.138911255368966));
#32924=CARTESIAN_POINT('Ctrl Pts',(2.0557604441427,1.,0.136777941218044));
#32925=CARTESIAN_POINT('Ctrl Pts',(2.06155781517844,1.,0.134598026192107));
#32926=CARTESIAN_POINT('Ctrl Pts',(2.06735123910319,1.,0.132372111547709));
#32927=CARTESIAN_POINT('Ctrl Pts',(2.07314114713047,1.,0.1301007483284));
#32928=CARTESIAN_POINT('Ctrl Pts',(2.07892715110967,1.,0.127784445276116));
#32929=CARTESIAN_POINT('Ctrl Pts',(2.08470840653628,1.,0.125423679412058));
#32930=CARTESIAN_POINT('Ctrl Pts',(2.09048392424826,1.,0.123018905621083));
#32931=CARTESIAN_POINT('Ctrl Pts',(2.09625292867756,1.,0.120570567965129));
#32932=CARTESIAN_POINT('Ctrl Pts',(2.10201512132945,1.,0.118079107988368));
#32933=CARTESIAN_POINT('Ctrl Pts',(2.10777050261359,1.,0.11554495768794));
#32934=CARTESIAN_POINT('Ctrl Pts',(2.11351924490335,1.,0.112968534419746));
#32935=CARTESIAN_POINT('Ctrl Pts',(2.11926155590849,1.,0.11035023613502));
#32936=CARTESIAN_POINT('Ctrl Pts',(2.12499752306927,1.,0.107690435231068));
#32937=CARTESIAN_POINT('Ctrl Pts',(2.1307270488718,1.,0.104989479152703));
#32938=CARTESIAN_POINT('Ctrl Pts',(2.13644992667052,1.,0.102247700556063));
#32939=CARTESIAN_POINT('Ctrl Pts',(2.14216588395974,1.,0.0994654261990741));
#32940=CARTESIAN_POINT('Ctrl Pts',(2.14787463531864,1.,0.0966429852305688));
#32941=CARTESIAN_POINT('Ctrl Pts',(2.15357593978377,1.,0.0937807218868344));
#32942=CARTESIAN_POINT('Ctrl Pts',(2.15926961544808,1.,0.0908789888108265));
#32943=CARTESIAN_POINT('Ctrl Pts',(2.16495552645275,1.,0.0879381291387821));
#32944=CARTESIAN_POINT('Ctrl Pts',(2.17063357871031,1.,0.0849584620835642));
#32945=CARTESIAN_POINT('Ctrl Pts',(2.1763037121106,1.,0.0819402680871938));
#32946=CARTESIAN_POINT('Ctrl Pts',(2.18196589448304,1.,0.0788837727683226));
#32947=CARTESIAN_POINT('Ctrl Pts',(2.1876201139874,1.,0.075789146583341));
#32948=CARTESIAN_POINT('Ctrl Pts',(2.19213712012956,1.,0.0732830357304275));
#32949=CARTESIAN_POINT('Ctrl Pts',(2.19552129483562,1.,0.0713863779524626));
#32950=CARTESIAN_POINT('Ctrl Pts',(2.19777582085261,1.,0.0701143536324925));
#32951=CARTESIAN_POINT('Ctrl Pts',(2.19890268624765,1.,0.0694764450219582));
#32952=CARTESIAN_POINT('',(1.74236521665491,0.,0.163289472382896));
#32953=CARTESIAN_POINT('Origin',(0.,1.,0.));
#32954=CARTESIAN_POINT('Origin',(0.,1.,0.));
#32955=CARTESIAN_POINT('Origin',(0.,0.,0.));
#33241=UNCERTAINTY_MEASURE_WITH_UNIT(LENGTH_MEASURE(0.001),#33300,
'DISTANCE_ACCURACY_VALUE',
'Maximum model space distance between geometric entities at asserted c
onnectivities');
#33247=UNCERTAINTY_MEASURE_WITH_UNIT(LENGTH_MEASURE(0.001),#33300,
'DISTANCE_ACCURACY_VALUE',
'Maximum model space distance between geometric entities at asserted c
onnectivities');
#33293=(
GEOMETRIC_REPRESENTATION_CONTEXT(3)
GLOBAL_UNCERTAINTY_ASSIGNED_CONTEXT((#33241))
GLOBAL_UNIT_ASSIGNED_CONTEXT((#33300,#33302,#33303))
REPRESENTATION_CONTEXT('','3D')
);
#33299=(
GEOMETRIC_REPRESENTATION_CONTEXT(3)
GLOBAL_UNCERTAINTY_ASSIGNED_CONTEXT((#33247))
GLOBAL_UNIT_ASSIGNED_CONTEXT((#33300,#33302,#33303))
REPRESENTATION_CONTEXT('','3D')
);
#33300=(
LENGTH_UNIT()
NAMED_UNIT(*)
SI_UNIT(.CENTI.,.METRE.)
);
#33302=(
NAMED_UNIT(*)
PLANE_ANGLE_UNIT()
SI_UNIT($,.RADIAN.)
);
#33303=(
NAMED_UNIT(*)
SI_UNIT($,.STERADIAN.)
SOLID_ANGLE_UNIT()
);
#33349=SHAPE_DEFINITION_REPRESENTATION(#33411,#33531);
#33411=PRODUCT_DEFINITION_SHAPE('',$,#33583);
#33531=SHAPE_REPRESENTATION('',(#14134),#33293);
#33537=PRODUCT_DEFINITION_CONTEXT('part definition',#33692,'design');
#33583=PRODUCT_DEFINITION('Spur Gear - Module 2, 20 Teeth, 12 mm Bore',
'Spur Gear - Module 2, 20 Teeth, 12 mm Bore',#33634,#33537);
#33634=PRODUCT_DEFINITION_FORMATION('',$,#33739);
#33692=APPLICATION_CONTEXT(
'Core Data for Automotive Mechanical Design Process');
#33693=PRODUCT_CONTEXT('part definition',#33692,'mechanical');
#33739=PRODUCT('Spur Gear - Module 2, 20 Teeth, 12 mm Bore',
'Spur Gear - Module 2, 20 Teeth, 12 mm Bore',
'Spur Gear - Module 2, 20 Teeth, 12 mm Bore',(#33693));
#33822=COLOUR_RGB('Off White',0.89,0.88,0.83);
#33823=FILL_AREA_STYLE_COLOUR('',#33822);
#33824=FILL_AREA_STYLE('',(#33823));
#33825=SURFACE_STYLE_FILL_AREA(#33824);
#33826=SURFACE_SIDE_STYLE('',(#33825));
#33827=SURFACE_STYLE_USAGE(.BOTH.,#33826);
#33828=PRESENTATION_STYLE_ASSIGNMENT((#33827));
ENDSEC;
END-ISO-10303-21;
